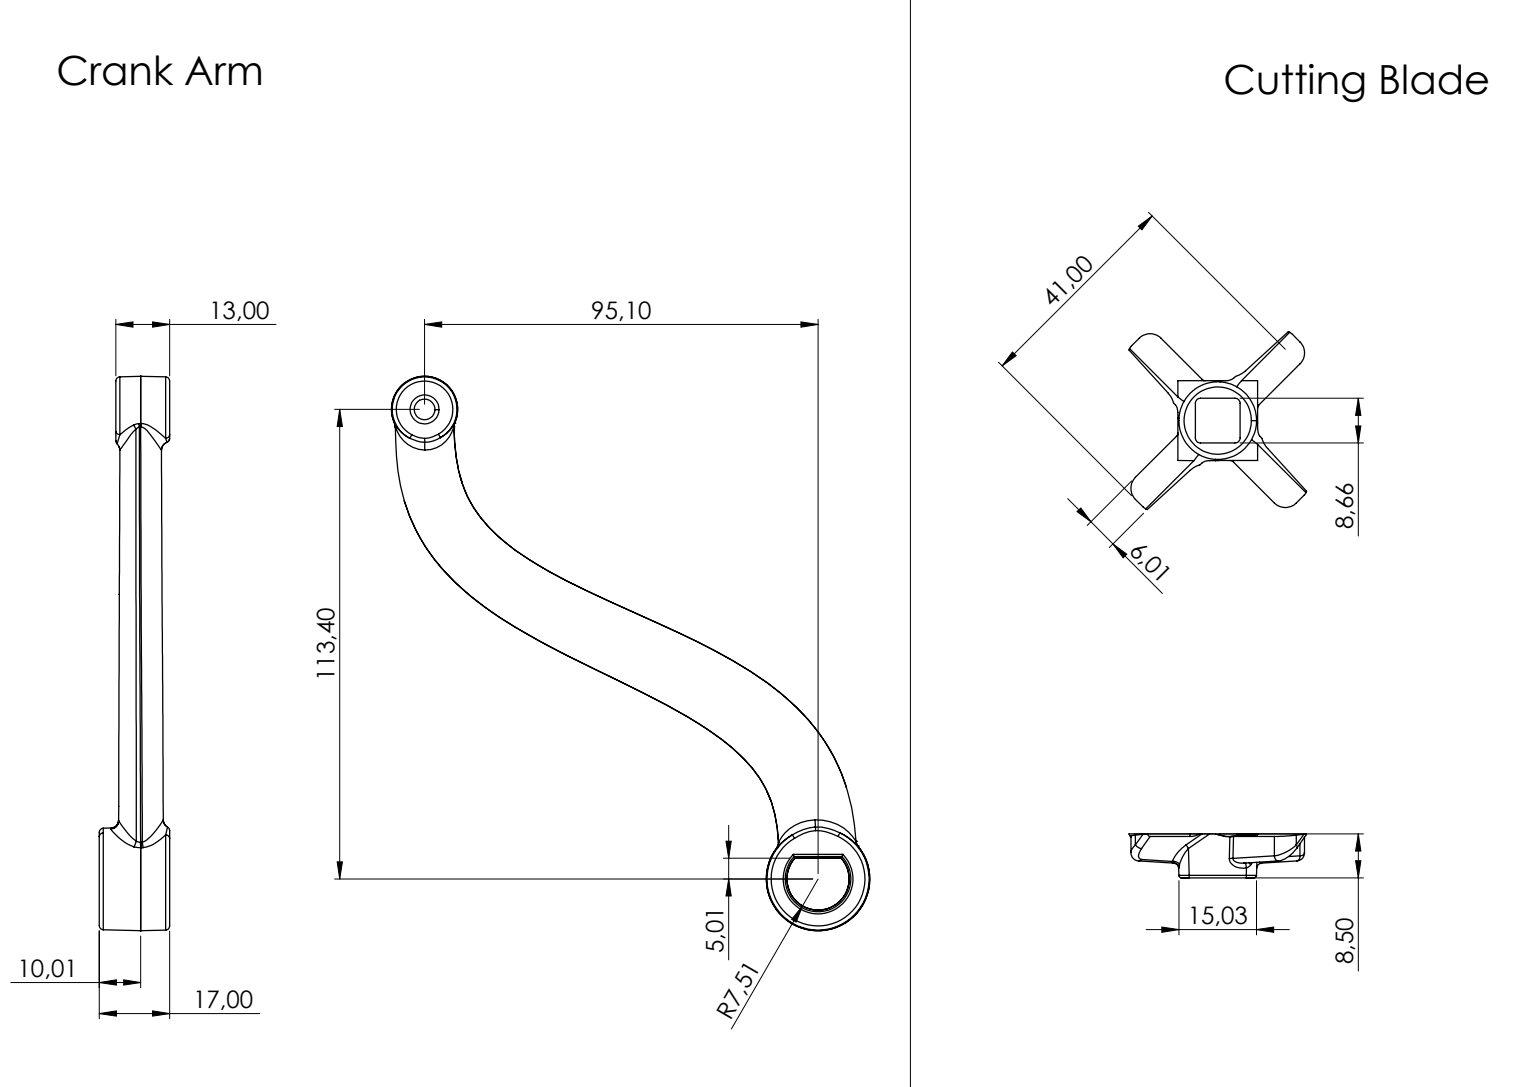
ISO-10303-21;
HEADER;
FILE_DESCRIPTION (('STEP AP214'),
    '1' );
FILE_NAME ('Crank Arm.step',
    '2026-10-06T09:49:54',
    ( '' ),
    ( '' ),
    'SwSTEP 2.0',
    'SolidWorks 2020',
    '' );
FILE_SCHEMA (( 'AUTOMOTIVE_DESIGN' ));
ENDSEC;

DATA;
#26=CARTESIAN_POINT ( 'NONE',  ( 1.285879139104720042E-15, 1391.913060387289988, 209.1218459572589836 ) ) ;
#31=CARTESIAN_POINT ( 'NONE',  ( -109.1321487942470014, 1384.869787291219836, 311.2644937792119322 ) ) ;
#38=CARTESIAN_POINT ( 'NONE',  ( -12.43709857819999876, 1391.584050621440156, 209.7498280055400244 ) ) ;
#39=CARTESIAN_POINT ( 'NONE',  ( -76.44887139282280941, 1385.142738521940146, 277.8929079653030385 ) ) ;
#40=CARTESIAN_POINT ( 'NONE',  ( -11.42765938226460065, 1391.913060387289988, 211.2666090369880010 ) ) ;
#42=ORIENTED_EDGE ( 'NONE', *, *, #61891, .F. ) ;
#48=CARTESIAN_POINT ( 'NONE',  ( -109.4839102700000097, 1384.920896159549784, 311.2841190732590348 ) ) ;
#82=CARTESIAN_POINT ( 'NONE',  ( -12.50903734399489942, 1378.842647904740033, 209.0065662253330174 ) ) ;
#89=ORIENTED_EDGE ( 'NONE', *, *, #96759, .T. ) ;
#109=CARTESIAN_POINT ( 'NONE',  ( -98.27039657997829636, 1384.868559307870100, 295.9020111865049785 ) ) ;
#127=CARTESIAN_POINT ( 'NONE',  ( -16.54254117820000047, 1379.596826475559965, 208.2028925074129688 ) ) ;
#137=DIRECTION ( 'NONE',  ( -1.000000000000000000, 0.000000000000000000, 0.000000000000000000 ) ) ;
#154=DIRECTION ( 'NONE',  ( -0.02617375475769094517, 0.9996573249755578150, 0.0004088821302708953143 ) ) ;
#161=CARTESIAN_POINT ( 'NONE',  ( -7.567241880450000124, 1385.515695150829970, 219.0512258816089854 ) ) ;
#174=EDGE_CURVE ( 'NONE', #66491, #29176, #106889, .T. ) ;
#176=CARTESIAN_POINT ( 'NONE',  ( -12.26345067459182658, 1378.041391332198373, 210.3086285185297868 ) ) ;
#182=CARTESIAN_POINT ( 'NONE',  ( -76.22674438190679780, 1384.646826080419942, 301.0779023118020064 ) ) ;
#183=CARTESIAN_POINT ( 'NONE',  ( -21.60464161394589766, 1384.953571151939968, 202.1045221056799903 ) ) ;
#189=CIRCLE ( 'NONE', #57423, 12.49965726619999984 ) ;
#199=CIRCLE ( 'NONE', #3805, 0.5000000000000157652 ) ;
#212=CARTESIAN_POINT ( 'NONE',  ( -31.38187927383859943, 1379.627610869280034, 219.3043553578710032 ) ) ;
#218=CARTESIAN_POINT ( 'NONE',  ( -106.9777543680000065, 1379.497227361900059, 308.7284971550590171 ) ) ;
#247=CARTESIAN_POINT ( 'NONE',  ( -18.61085923841566014, 1379.601406803549708, 208.6983520666371419 ) ) ;
#248=CARTESIAN_POINT ( 'NONE',  ( -18.76550561599999867, 1380.296266888499986, 210.4015402955490117 ) ) ;
#274=CARTESIAN_POINT ( 'NONE',  ( -62.99252469870000937, 1388.208599921950054, 284.2099993179589887 ) ) ;
#276=CARTESIAN_POINT ( 'NONE',  ( -56.29735061249719763, 1385.085427587770027, 274.2983070328880331 ) ) ;
#299=CARTESIAN_POINT ( 'NONE',  ( -107.7923298369999969, 1386.973993580999831, 297.6574877858589616 ) ) ;
#353=CARTESIAN_POINT ( 'NONE',  ( -8.173822499230000815, 1384.405547763340110, 199.6789892872290011 ) ) ;
#361=EDGE_LOOP ( 'NONE', ( #97319, #80641, #79673, #74910 ) ) ;
#362=DIRECTION ( 'NONE',  ( 1.836970198721029688E-16, 1.000000000000000000, -2.953460612019999929E-19 ) ) ;
#374=ORIENTED_EDGE ( 'NONE', *, *, #31699, .T. ) ;
#375=CARTESIAN_POINT ( 'NONE',  ( -109.5441724410000006, 1374.437034645689891, 304.2218460466590386 ) ) ;
#379=AXIS2_PLACEMENT_3D ( 'NONE', #95016, #67622, #7691 ) ;
#382=CARTESIAN_POINT ( 'NONE',  ( -39.58883837791880467, 1384.581576029320104, 212.5204386266630081 ) ) ;
#389=CARTESIAN_POINT ( 'NONE',  ( -36.13018326403506109, 1379.645813938799392, 224.1534624346936937 ) ) ;
#392=ADVANCED_FACE ( 'NONE', ( #11528 ), #84870, .F. ) ;
#395=CARTESIAN_POINT ( 'NONE',  ( -68.60472032309999690, 1379.747634528509707, 279.7221279746590312 ) ) ;
#404=CARTESIAN_POINT ( 'NONE',  ( -73.55923423229999969, 1384.652831667379814, 298.9494481685590017 ) ) ;
#406=CARTESIAN_POINT ( 'NONE',  ( -13.74298021802130165, 1385.299105108359981, 219.1768037944160028 ) ) ;
#424=CARTESIAN_POINT ( 'NONE',  ( -109.1307141485102790, 1384.906036703127711, 311.2647582669765711 ) ) ;
#446=CARTESIAN_POINT ( 'NONE',  ( -54.30401535559919779, 1383.804998114640057, 270.0689160511349769 ) ) ;
#453=CARTESIAN_POINT ( 'NONE',  ( -53.45887188369999876, 1384.635297440300064, 230.7554238970589893 ) ) ;
#463=CARTESIAN_POINT ( 'NONE',  ( -108.1525126060000019, 1382.602476773729904, 297.8175945742589761 ) ) ;
#465=CARTESIAN_POINT ( 'NONE',  ( -8.752237007995399054, 1384.883920018590061, 220.6821560429810063 ) ) ;
#486=CARTESIAN_POINT ( 'NONE',  ( -105.7100346900000005, 1391.009939533860006, 306.5104643349590106 ) ) ;
#499=EDGE_CURVE ( 'NONE', #98535, #40166, #189, .T. ) ;
#526=EDGE_CURVE ( 'NONE', #91726, #23648, #37737, .T. ) ;
#530=DIRECTION ( 'NONE',  ( 0.03782478994198348876, 0.9992229352747146187, 0.01108200734653209431 ) ) ;
#535=CARTESIAN_POINT ( 'NONE',  ( -8.746878246584900021E-16, 1386.598172472869919, 199.6218459572590120 ) ) ;
#536=CARTESIAN_POINT ( 'NONE',  ( -9.252564866275420741, 1386.194685219555595, 218.4639695156267578 ) ) ;
#544=CARTESIAN_POINT ( 'NONE',  ( -9.786751275049999421, 1380.128435987210196, 216.7642765186190275 ) ) ;
#550=CARTESIAN_POINT ( 'NONE',  ( -13.17267676139999999, 1389.960074679450145, 205.5617118964289887 ) ) ;
#580=CARTESIAN_POINT ( 'NONE',  ( -109.8949752469999908, 1384.902872212460125, 297.0284569597590121 ) ) ;
#584=CARTESIAN_POINT ( 'NONE',  ( -13.93561471908700078, 1390.368461153759881, 210.8007146514599981 ) ) ;
#588=CARTESIAN_POINT ( 'NONE',  ( -107.2899050854710055, 1379.886892357829993, 309.1794776302379546 ) ) ;
#590=CARTESIAN_POINT ( 'NONE',  ( -12.92544628329999945, 1379.594338187410131, 211.1425626820590082 ) ) ;
#591=CARTESIAN_POINT ( 'NONE',  ( -11.31021147849999942, 1391.913060277239993, 206.0247873240190302 ) ) ;
#592=CARTESIAN_POINT ( 'NONE',  ( -73.83470183118490127, 1385.130927357710107, 273.3978214202909953 ) ) ;
#593=CARTESIAN_POINT ( 'NONE',  ( -9.878631019772029731, 1391.913060387289988, 214.6972032143189892 ) ) ;
#628=B_SPLINE_CURVE_WITH_KNOTS ( 'NONE', 3,
 ( #92990, #23025, #91894, #57227, #91357, #49357, #48822, #7343, #24119, #83486, #42053, #109808, #82946 ),
 .UNSPECIFIED., .F., .F.,
 ( 4, 3, 3, 3, 4 ),
 ( -3.958900035302570064, -3.804518807040609740, -3.535848030339469705, -3.399392778577199792, -3.112795747787960199 ),
 .UNSPECIFIED. ) ;
#653=CARTESIAN_POINT ( 'NONE',  ( -88.76367195209469685, 1384.833741781400022, 291.7667102089239961 ) ) ;
#654=ORIENTED_EDGE ( 'NONE', *, *, #54816, .F. ) ;
#670=CARTESIAN_POINT ( 'NONE',  ( -18.79413418600000085, 1379.714553871910084, 209.1009770162550012 ) ) ;
#686=CARTESIAN_POINT ( 'NONE',  ( -8.604752758000000057, 1384.917533019219945, 199.8686412392590057 ) ) ;
#691=CARTESIAN_POINT ( 'NONE',  ( 12.50000000000000000, 1384.913060387289988, 209.1218459572589836 ) ) ;
#723=CARTESIAN_POINT ( 'NONE',  ( -63.98295147832750018, 1384.681148330740143, 287.2755451078210172 ) ) ;
#724=CARTESIAN_POINT ( 'NONE',  ( -27.30672991563199759, 1384.963778074569746, 204.2309128032860031 ) ) ;
#737=ADVANCED_FACE ( 'NONE', ( #27645 ), #103907, .T. ) ;
#741=CARTESIAN_POINT ( 'NONE',  ( -8.579104367239999362, 1382.291193835669901, 200.1141359521089953 ) ) ;
#756=CARTESIAN_POINT ( 'NONE',  ( -59.53909452845530126, 1379.721836142610073, 264.8166016163610266 ) ) ;
#762=CARTESIAN_POINT ( 'NONE',  ( -107.5863934789999945, 1379.032352484299963, 308.9389182505590270 ) ) ;
#779=CARTESIAN_POINT ( 'NONE',  ( -5.013279353754826140, 1375.417533171782679, 203.5257404570949973 ) ) ;
#789=CARTESIAN_POINT ( 'NONE',  ( -57.75160514174648796, 1379.717046060986377, 256.2888408195211696 ) ) ;
#790=CARTESIAN_POINT ( 'NONE',  ( -26.65670438269999920, 1376.179549128069993, 211.2412313610989827 ) ) ;
#794=CARTESIAN_POINT ( 'NONE',  ( -105.5244021762739948, 1378.591211549419995, 305.0228942085889798 ) ) ;
#796=ORIENTED_EDGE ( 'NONE', *, *, #6343, .F. ) ;
#817=CARTESIAN_POINT ( 'NONE',  ( -73.59349969589999318, 1386.581895584289896, 298.9135147644589665 ) ) ;
#842=ADVANCED_FACE ( 'NONE', ( #71348 ), #98540, .T. ) ;
#846=CARTESIAN_POINT ( 'NONE',  ( -109.2380410539999929, 1385.254002988119964, 297.1509341280589638 ) ) ;
#862=CARTESIAN_POINT ( 'NONE',  ( -16.22265104649770251, 1384.873541373520084, 219.7134262672329896 ) ) ;
#891=EDGE_LOOP ( 'NONE', ( #56379, #88097, #94429, #5501 ) ) ;
#908=B_SPLINE_SURFACE_WITH_KNOTS ( 'NONE', 5, 5, ( 
 ( #76165, #109767, #85650, #40900, #100792, #42561 ),
 ( #24083, #8951, #42016, #68898, #58817, #50433 ),
 ( #50973, #580, #49321, #49872, #23545, #57737 ),
 ( #109231, #76714, #83447, #43124, #32515, #51518 ),
 ( #58272, #7306, #75632, #6742, #92956, #67235 ),
 ( #93499, #67780, #16770, #91855, #85103, #33047 ) ),
 .UNSPECIFIED., .F., .F., .F.,
 ( 6, 6 ),
 ( 6, 6 ),
 ( 29.54622938989999881, 29.61002813500000030 ),
 ( 0.000000000000000000, 2.000000000000000000 ),
 .UNSPECIFIED. ) ;
#920=CARTESIAN_POINT ( 'NONE',  ( -113.4000000000000057, 1374.720597897390007, 302.6503168488589495 ) ) ;
#922=CARTESIAN_POINT ( 'NONE',  ( -106.1401956836040057, 1378.913060387289988, 302.5623463823779957 ) ) ;
#927=CARTESIAN_POINT ( 'NONE',  ( -75.49934453870000084, 1384.893650425089845, 276.6853632062590123 ) ) ;
#928=CARTESIAN_POINT ( 'NONE',  ( -51.30093226525310257, 1384.625592632969756, 227.3549881365390206 ) ) ;
#930=CARTESIAN_POINT ( 'NONE',  ( -109.1320112420000044, 1384.953741877089897, 311.2644403302589353 ) ) ;
#939=CARTESIAN_POINT ( 'NONE',  ( -68.65285585769998988, 1379.747727628990106, 279.8365758267589740 ) ) ;
#947=CARTESIAN_POINT ( 'NONE',  ( -54.13887208369999371, 1385.096747890979941, 270.3642349231589606 ) ) ;
#993=CARTESIAN_POINT ( 'NONE',  ( -69.93979052779329209, 1383.785293178040092, 294.7370205497300049 ) ) ;
#994=CIRCLE ( 'NONE', #29578, 2.000079901618746270 ) ;
#995=CARTESIAN_POINT ( 'NONE',  ( -108.2039566672529958, 1378.913060387289988, 299.7295690038039879 ) ) ;
#1001=CARTESIAN_POINT ( 'NONE',  ( -59.38610754540000158, 1383.797318715759957, 279.8430129459590034 ) ) ;
#1013=CARTESIAN_POINT ( 'NONE',  ( -107.7596963679999931, 1382.859817520469733, 297.6961126062590210 ) ) ;
#1046=CARTESIAN_POINT ( 'NONE',  ( -9.503490513250000049, 1386.215136675220037, 200.2136258941289952 ) ) ;
#1081=ORIENTED_EDGE ( 'NONE', *, *, #10293, .T. ) ;
#1084=B_SPLINE_SURFACE_WITH_KNOTS ( 'NONE', 5, 5, ( 
 ( #42749, #102620, #93139, #762, #85849, #103180 ),
 ( #34890, #218, #51153, #9687, #84733, #92581 ),
 ( #33232, #25920, #67975, #26482, #60118, #94804 ),
 ( #15853, #33779, #18079, #52274, #42199, #76350 ),
 ( #75802, #78002, #24807, #32689, #110499, #109953 ),
 ( #66869, #100977, #24273, #102083, #67421, #101520 ),
 ( #25366, #70203, #78561, #19744, #46081, #11906 ),
 ( #105977, #61246, #70749, #11367, #10810, #46631 ),
 ( #12446, #89158, #54491, #28149, #104860, #88626 ) ),
 .UNSPECIFIED., .F., .F., .F.,
 ( 6, 3, 6 ),
 ( 6, 6 ),
 ( 0.000000000000000000, 5.531936552890000414, 12.17660274970000067 ),
 ( 0.000000000000000000, 1.000000000000000000 ),
 .UNSPECIFIED. ) ;
#1086=CARTESIAN_POINT ( 'NONE',  ( -13.39809219260000006, 1386.967483829560024, 218.7383260501090092 ) ) ;
#1095=CARTESIAN_POINT ( 'NONE',  ( -10.13100692099999911, 1382.082910451279986, 217.5460056582589914 ) ) ;
#1101=CARTESIAN_POINT ( 'NONE',  ( -11.29470234270000084, 1390.474510999679978, 203.7985412330889972 ) ) ;
#1129=CARTESIAN_POINT ( 'NONE',  ( -8.083483728235815846, 1386.109445660887104, 199.6283091834757215 ) ) ;
#1136=CARTESIAN_POINT ( 'NONE',  ( -13.26126580242469899, 1390.209151648439956, 212.6158348635119921 ) ) ;
#1140=CARTESIAN_POINT ( 'NONE',  ( -108.8427904636022134, 1381.850845790319909, 310.6994421841279745 ) ) ;
#1141=CARTESIAN_POINT ( 'NONE',  ( -12.26108091377107634, 1377.626920165065258, 208.0100024370453298 ) ) ;
#1144=CARTESIAN_POINT ( 'NONE',  ( -86.70549396914439910, 1385.182048704240060, 290.2386611732610504 ) ) ;
#1146=CARTESIAN_POINT ( 'NONE',  ( -9.946516861848831326, 1391.913060387289988, 214.5797999757839989 ) ) ;
#1147=CARTESIAN_POINT ( 'NONE',  ( -32.53397683490000247, 1379.726329037039932, 216.1069825312089847 ) ) ;
#1175=DIRECTION ( 'NONE',  ( -0.9998780014336184907, 0.000000000000000000, 0.01561993114942984012 ) ) ;
#1203=CARTESIAN_POINT ( 'NONE',  ( -97.03291587454688738, 1384.864417997589953, 295.5831496746029643 ) ) ;
#1220=CARTESIAN_POINT ( 'NONE',  ( -16.52535657530000179, 1379.585817439869743, 208.2843806234300246 ) ) ;
#1224=CARTESIAN_POINT ( 'NONE',  ( -68.75533708345575690, 1379.747887839387431, 280.3280563178295210 ) ) ;
#1239=CARTESIAN_POINT ( 'NONE',  ( -13.57816498729999921, 1379.569537801319939, 207.8818212186490086 ) ) ;
#1266=AXIS2_PLACEMENT_3D ( 'NONE', #76000, #101734, #93889 ) ;
#1271=CARTESIAN_POINT ( 'NONE',  ( -77.89971934322829838, 1384.643069586999900, 302.3865563694679963 ) ) ;
#1272=CARTESIAN_POINT ( 'NONE',  ( -18.95953277411649651, 1384.948900335349890, 201.3970670253520154 ) ) ;
#1289=CARTESIAN_POINT ( 'NONE',  ( -8.219449892280000114, 1384.003553985900226, 199.7324766670489851 ) ) ;
#1301=CIRCLE ( 'NONE', #74597, 2.000013666866326201 ) ;
#1302=CARTESIAN_POINT ( 'NONE',  ( -66.37701120922260145, 1379.742216766350111, 277.0613536044180023 ) ) ;
#1310=CARTESIAN_POINT ( 'NONE',  ( -7.767687465479999886, 1384.983142744430097, 218.9170564598889825 ) ) ;
#1329=AXIS2_PLACEMENT_3D ( 'NONE', #10990, #55217, #12641 ) ;
#1333=CARTESIAN_POINT ( 'NONE',  ( -49.27402874327646742, 1379.685930775072848, 238.1797779762692926 ) ) ;
#1349=CARTESIAN_POINT ( 'NONE',  ( 3.555115653736739510E-15, 1384.926148861439970, 209.1218459572589836 ) ) ;
#1352=CARTESIAN_POINT ( 'NONE',  ( -104.6408027911641483, 1379.604531764216517, 304.0225355773446836 ) ) ;
#1361=CARTESIAN_POINT ( 'NONE',  ( -73.55519582189999994, 1385.011955127469946, 298.9534985252589649 ) ) ;
#1372=CARTESIAN_POINT ( 'NONE',  ( -108.8616956595720069, 1383.655566382730058, 311.0497432310580166 ) ) ;
#1421=CARTESIAN_POINT ( 'NONE',  ( -109.5441724370000003, 1379.437061298989875, 305.1680627026370303 ) ) ;
#1450=B_SPLINE_SURFACE_WITH_KNOTS ( 'NONE', 5, 5, ( 
 ( #90304, #23657, #57839, #21975, #56167, #91966 ),
 ( #81906, #38256, #5775, #72439, #106571, #29857 ),
 ( #39364, #98160, #89765, #73538, #75188, #85766 ),
 ( #58381, #66797, #17432, #24733, #33156, #58930 ),
 ( #75733, #25842, #67896, #686, #7958, #109877 ),
 ( #110422, #67345, #101443, #93061, #16335, #17998 ) ),
 .UNSPECIFIED., .F., .F., .F.,
 ( 6, 6 ),
 ( 6, 6 ),
 ( 0.9322655043309999723, 1.047387711740000116 ),
 ( 0.000000000000000000, 2.000000000000000000 ),
 .UNSPECIFIED. ) ;
#1454=CARTESIAN_POINT ( 'NONE',  ( -87.43041093610000303, 1379.577971548199912, 299.9734862988590294 ) ) ;
#1456=ADVANCED_FACE ( 'NONE', ( #108738 ), #94755, .F. ) ;
#1466=CARTESIAN_POINT ( 'NONE',  ( -58.30221543510000259, 1384.791840522580060, 240.0691493971590091 ) ) ;
#1468=CARTESIAN_POINT ( 'NONE',  ( -65.89286211545359606, 1384.710728713680055, 257.0461978634630213 ) ) ;
#1471=CARTESIAN_POINT ( 'NONE',  ( -103.5990824459999970, 1389.912137903419989, 305.4537645068589882 ) ) ;
#1480=CARTESIAN_POINT ( 'NONE',  ( -68.67274465469999711, 1379.748163774529985, 279.9618448723590518 ) ) ;
#1482=CARTESIAN_POINT ( 'NONE',  ( -115.5939564047259296, 1379.013060387289897, 305.4204098037694735 ) ) ;
#1489=CARTESIAN_POINT ( 'NONE',  ( -38.49223698079999423, 1385.058880994630044, 239.3118539506589855 ) ) ;
#1491=CARTESIAN_POINT ( 'NONE',  ( -105.7942887633819993, 1378.913060387289988, 304.0474587704230203 ) ) ;
#1508=B_SPLINE_CURVE_WITH_KNOTS ( 'NONE', 3,
 ( #110150, #9352, #101176, #24470, #42390, #60313 ),
 .UNSPECIFIED., .F., .F.,
 ( 4, 2, 4 ),
 ( 0.000000000000000000, 0.5000000000000000000, 1.000000000000000000 ),
 .UNSPECIFIED. ) ;
#1535=CIRCLE ( 'NONE', #87369, 12.26364123839999998 ) ;
#1538=CARTESIAN_POINT ( 'NONE',  ( -75.52559667918460207, 1383.780383530929839, 300.2699059305949731 ) ) ;
#1545=VERTEX_POINT ( 'NONE', #63867 ) ;
#1547=CARTESIAN_POINT ( 'NONE',  ( -87.19453865519999169, 1382.337400661289848, 307.1204035211590053 ) ) ;
#1557=CARTESIAN_POINT ( 'NONE',  ( -109.2768968829999920, 1384.496076674440019, 297.1408104247589677 ) ) ;
#1573=FACE_OUTER_BOUND ( 'NONE', #66351, .T. ) ;
#1601=EDGE_CURVE ( 'NONE', #93351, #108323, #72640, .T. ) ;
#1634=CARTESIAN_POINT ( 'NONE',  ( -20.33527840200000014, 1390.981646659919761, 210.8560405308990084 ) ) ;
#1635=CARTESIAN_POINT ( 'NONE',  ( -14.24353422718318463, 1390.369519709444148, 210.8398536836253356 ) ) ;
#1645=CARTESIAN_POINT ( 'NONE',  ( -8.680550271810000496, 1382.887713811429876, 218.3027530060789729 ) ) ;
#1662=CARTESIAN_POINT ( 'NONE',  ( -106.3976693117229928, 1390.939243848519936, 307.7527733253859878 ) ) ;
#1671=CARTESIAN_POINT ( 'NONE',  ( -31.84935467931069297, 1383.839719338520126, 229.8416280207219984 ) ) ;
#1680=CARTESIAN_POINT ( 'NONE',  ( -1.458447685501650145E-16, 1382.910363916049846, 199.8625637235290071 ) ) ;
#1687=CARTESIAN_POINT ( 'NONE',  ( -14.52654072983339972, 1379.768571760160057, 208.3454318067070119 ) ) ;
#1695=CARTESIAN_POINT ( 'NONE',  ( -12.08187496630000091, 1391.708070121689843, 207.0208056324590018 ) ) ;
#1696=CARTESIAN_POINT ( 'NONE',  ( -98.94538731745480220, 1385.218168442259866, 296.0687099710040115 ) ) ;
#1731=FACE_OUTER_BOUND ( 'NONE', #74136, .T. ) ;
#1739=CARTESIAN_POINT ( 'NONE',  ( -13.86717347501279995, 1379.678627288110192, 208.3009849253440109 ) ) ;
#1749=ORIENTED_EDGE ( 'NONE', *, *, #3895, .F. ) ;
#1763=CARTESIAN_POINT ( 'NONE',  ( -102.6485531311329993, 1384.882470662279957, 296.6730287615140469 ) ) ;
#1781=CARTESIAN_POINT ( 'NONE',  ( -41.95996988479999601, 1379.671663521220125, 226.0894461641589999 ) ) ;
#1784=CARTESIAN_POINT ( 'NONE',  ( -68.56276905708799063, 1379.747764319654607, 280.1490247722647950 ) ) ;
#1797=ORIENTED_EDGE ( 'NONE', *, *, #100031, .F. ) ;
#1799=CARTESIAN_POINT ( 'NONE',  ( -7.545064063707340729, 1384.907232462019920, 219.0876311385090105 ) ) ;
#1817=DIRECTION ( 'NONE',  ( 0.1225044380228070551, 0.9831695928899274461, -0.1355367635786350333 ) ) ;
#1824=CARTESIAN_POINT ( 'NONE',  ( -7.628194758486819715, 1383.866806825199774, 218.9897990120470013 ) ) ;
#1837=CARTESIAN_POINT ( 'NONE',  ( -69.10968088804719400, 1384.665037752149829, 294.0407317603679758 ) ) ;
#1838=CARTESIAN_POINT ( 'NONE',  ( -15.47609788629169891, 1384.942714744960085, 200.6910050388860043 ) ) ;
#1852=CARTESIAN_POINT ( 'NONE',  ( -106.6950745027010043, 1391.913060387289988, 305.9031442834140080 ) ) ;
#1857=CARTESIAN_POINT ( 'NONE',  ( -14.08318393682589864, 1379.709325990200114, 211.5303917806009792 ) ) ;
#1871=CARTESIAN_POINT ( 'NONE',  ( -65.43163292693739663, 1379.743657604059763, 275.4463174256679849 ) ) ;
#1903=CARTESIAN_POINT ( 'NONE',  ( -44.66902661210603043, 1379.669579522011190, 230.0472852312407497 ) ) ;
#1915=EDGE_CURVE ( 'NONE', #68857, #40412, #43486, .T. ) ;
#1924=CARTESIAN_POINT ( 'NONE',  ( -105.0581303879369983, 1379.236400313860031, 304.0328620142400382 ) ) ;
#1933=CARTESIAN_POINT ( 'NONE',  ( -74.25289801200000284, 1388.141632471819776, 298.2335420860590034 ) ) ;
#1944=CARTESIAN_POINT ( 'NONE',  ( -105.6599733740739993, 1378.369188341159997, 305.5461949359690266 ) ) ;
#1967=AXIS2_PLACEMENT_3D ( 'NONE', #95143, #19521, #53727 ) ;
#1972=CARTESIAN_POINT ( 'NONE',  ( -9.627136608023121767, 1384.891069265470151, 218.7309310236159945 ) ) ;
#2027=CARTESIAN_POINT ( 'NONE',  ( -77.18524044800000183, 1379.656469663269945, 292.4664101653590365 ) ) ;
#2034=CARTESIAN_POINT ( 'NONE',  ( -113.4000000000000057, 1385.138976307909843, 297.2272069998589927 ) ) ;
#2035=CARTESIAN_POINT ( 'NONE',  ( -60.36450283880899548, 1384.675237924389876, 244.7949774597909993 ) ) ;
#2047=CARTESIAN_POINT ( 'NONE',  ( -65.32973268749998397, 1379.744446857699813, 273.2270638632589908 ) ) ;
#2055=CARTESIAN_POINT ( 'NONE',  ( -38.48821451509999747, 1384.926710553620069, 239.3141293533589931 ) ) ;
#2103=CARTESIAN_POINT ( 'NONE',  ( -101.9385972633359927, 1383.762759256019990, 310.8318512473720148 ) ) ;
#2106=CARTESIAN_POINT ( 'NONE',  ( -109.0682903905509988, 1384.413520338990111, 311.2316106067269743 ) ) ;
#2112=CARTESIAN_POINT ( 'NONE',  ( -85.86261655710001151, 1384.821806127680020, 289.6800030968590249 ) ) ;
#2122=CARTESIAN_POINT ( 'NONE',  ( -109.9959328080000063, 1384.355667310579975, 296.9977477969590041 ) ) ;
#2199=CARTESIAN_POINT ( 'NONE',  ( -24.70417392370000087, 1389.604960788569997, 206.5185001640990095 ) ) ;
#2238=CARTESIAN_POINT ( 'NONE',  ( -35.56111957166950077, 1383.834697306850103, 234.6955540351449940 ) ) ;
#2248=CARTESIAN_POINT ( 'NONE',  ( -105.0581303879369983, 1379.236400313860031, 304.0328620142400382 ) ) ;
#2249=CARTESIAN_POINT ( 'NONE',  ( -8.296934851823509760, 1386.806139525614526, 199.8388016180733473 ) ) ;
#2255=CARTESIAN_POINT ( 'NONE',  ( -12.31958819330829868, 1391.699967522870111, 210.6753496357469828 ) ) ;
#2259=ADVANCED_FACE ( 'NONE', ( #50931 ), #6146, .T. ) ;
#2263=CARTESIAN_POINT ( 'NONE',  ( -7.966114795899199130, 1384.917223774180002, 199.4892816035240060 ) ) ;
#2264=CARTESIAN_POINT ( 'NONE',  ( -102.2538918586309933, 1385.226474943340008, 296.6373044331759843 ) ) ;
#2291=CARTESIAN_POINT ( 'NONE',  ( -106.6038969349999945, 1381.976044154610008, 298.3535665123590093 ) ) ;
#2321=CARTESIAN_POINT ( 'NONE',  ( -12.25307189289999954, 1391.743053431310045, 210.3744810088190036 ) ) ;
#2339=CARTESIAN_POINT ( 'NONE',  ( -44.27735363219999698, 1379.663868217249956, 229.4728106293590031 ) ) ;
#2343=CARTESIAN_POINT ( 'NONE',  ( -67.15060528499047621, 1379.747519056922101, 278.1647121854331886 ) ) ;
#2350=CARTESIAN_POINT ( 'NONE',  ( -67.08107980928619440, 1385.034953735319959, 291.5504916563910456 ) ) ;
#2352=CARTESIAN_POINT ( 'NONE',  ( -8.970890765399998301, 1384.951408361539961, 199.9338804842589923 ) ) ;
#2366=DIRECTION ( 'NONE',  ( 0.0001171895853481130984, -0.004053780167009412259, -0.9999917765326665764 ) ) ;
#2385=CARTESIAN_POINT ( 'NONE',  ( -7.768355502971520110, 1383.288536228370049, 218.8604790520440133 ) ) ;
#2399=CARTESIAN_POINT ( 'NONE',  ( -76.64144279794061276, 1384.645875352879784, 301.4166218965220310 ) ) ;
#2400=CARTESIAN_POINT ( 'NONE',  ( -31.39107788089150120, 1384.971443476370041, 206.3467394566210089 ) ) ;
#2407=CARTESIAN_POINT ( 'NONE',  ( -8.847848347470000263, 1384.943898188619869, 199.9248160043189841 ) ) ;
#2417=CARTESIAN_POINT ( 'NONE',  ( -9.813982587879999997, 1383.225161719749849, 200.4195862986289853 ) ) ;
#2430=CARTESIAN_POINT ( 'NONE',  ( -65.82654097011999283, 1379.741992558670063, 276.1399068737349580 ) ) ;
#2443=CARTESIAN_POINT ( 'NONE',  ( -106.0207696801649888, 1378.913060388890017, 305.3967244531619940 ) ) ;
#2456=CIRCLE ( 'NONE', #52702, 8.432239102140000497 ) ;
#2460=CARTESIAN_POINT ( 'NONE',  ( -8.862374925020001015, 1384.916129524170174, 218.6851829152190305 ) ) ;
#2463=CARTESIAN_POINT ( 'NONE',  ( -49.26428229891999422, 1379.685895086444134, 238.1610838164967845 ) ) ;
#2477=CARTESIAN_POINT ( 'NONE',  ( 10.11243515225073253, 1384.926148861439970, 216.4689601570716206 ) ) ;
#2484=CARTESIAN_POINT ( 'NONE',  ( -104.8708816957486079, 1379.440243493634625, 304.0281164857488534 ) ) ;
#2487=CARTESIAN_POINT ( 'NONE',  ( -9.094257307180781069, 1384.874748761890260, 199.9429999480310016 ) ) ;
#2492=CARTESIAN_POINT ( 'NONE',  ( -102.7364941740000006, 1384.940050820800025, 311.2335147922589726 ) ) ;
#2503=CARTESIAN_POINT ( 'NONE',  ( -105.9021060456189929, 1378.331563972840058, 306.6119379298179979 ) ) ;
#2529=CARTESIAN_POINT ( 'NONE',  ( -21.51311642161260096, 1384.857552017839907, 221.6326953624779890 ) ) ;
#2563=CARTESIAN_POINT ( 'NONE',  ( -107.2481891120000057, 1387.964334016630119, 309.9317261882590628 ) ) ;
#2585=CARTESIAN_POINT ( 'NONE',  ( -77.18524045069999318, 1374.656469662890004, 292.4664101653590365 ) ) ;
#2586=CARTESIAN_POINT ( 'NONE',  ( -106.9163825377050046, 1378.913060387289988, 301.2728918013489761 ) ) ;
#2594=DIRECTION ( 'NONE',  ( -1.000000000000000000, 0.000000000000000000, 0.000000000000000000 ) ) ;
#2597=CARTESIAN_POINT ( 'NONE',  ( -8.743435183079999007, 1384.548231727749908, 218.5812667456789882 ) ) ;
#2602=CARTESIAN_POINT ( 'NONE',  ( -65.82430152899999598, 1379.749194687180079, 274.2810710116589803 ) ) ;
#2611=CARTESIAN_POINT ( 'NONE',  ( -47.38272174249999580, 1385.138016709929843, 256.2741787814589998 ) ) ;
#2613=CARTESIAN_POINT ( 'NONE',  ( -33.03375078350489957, 1385.219055440710008, 231.5328850939089875 ) ) ;
#2657=CARTESIAN_POINT ( 'NONE',  ( -93.71881660438820916, 1383.767977992140004, 309.5718267011319540 ) ) ;
#2659=CARTESIAN_POINT ( 'NONE',  ( -109.2480983758639894, 1384.372607579929991, 311.2262217477910440 ) ) ;
#2666=CARTESIAN_POINT ( 'NONE',  ( -92.78435512849998190, 1384.849527344140142, 294.1459074807589786 ) ) ;
#2672=CARTESIAN_POINT ( 'NONE',  ( -109.3498435130000104, 1384.940401497779931, 297.1386112594590259 ) ) ;
#2704=CARTESIAN_POINT ( 'NONE',  ( -113.4000000000000057, 1390.913060387289988, 304.2218459572590064 ) ) ;
#2737=CARTESIAN_POINT ( 'NONE',  ( -11.65147249325539924, 1391.913060387150153, 208.7366933367970034 ) ) ;
#2748=CARTESIAN_POINT ( 'NONE',  ( -25.91586689989999925, 1384.961148014880109, 203.4475886829490037 ) ) ;
#2755=CARTESIAN_POINT ( 'NONE',  ( -8.001312726290001009, 1383.415254610280044, 218.6981543553289953 ) ) ;
#2773=CARTESIAN_POINT ( 'NONE',  ( -109.8950784940000034, 1385.179886903279794, 297.0358873837590181 ) ) ;
#2777=FACE_OUTER_BOUND ( 'NONE', #106070, .T. ) ;
#2784=CARTESIAN_POINT ( 'NONE',  ( -23.70810543552709859, 1383.849544535609994, 222.6483769287150096 ) ) ;
#2787=DIRECTION ( 'NONE',  ( 1.835183309750130004E-16, 1.000000000000000000, 1.599799320660000123E-19 ) ) ;
#2792=CARTESIAN_POINT ( 'NONE',  ( -8.911791977641406959, 1388.063585253917608, 200.4736995634368100 ) ) ;
#2801=CARTESIAN_POINT ( 'NONE',  ( -12.56550536004469976, 1389.228114667070031, 215.4313542344819723 ) ) ;
#2808=CARTESIAN_POINT ( 'NONE',  ( -104.7009857956030032, 1385.232336910320100, 296.9001550543150074 ) ) ;
#2831=ORIENTED_EDGE ( 'NONE', *, *, #37412, .T. ) ;
#2837=LINE ( 'NONE', #28569, #78414 ) ;
#2881=CARTESIAN_POINT ( 'NONE',  ( -108.8461099330000081, 1385.969494106900129, 297.2525754554590094 ) ) ;
#2886=EDGE_CURVE ( 'NONE', #77278, #33852, #29899, .T. ) ;
#2889=CARTESIAN_POINT ( 'NONE',  ( -62.71435643172744534, 1379.746901600607089, 270.6043089139369613 ) ) ;
#2895=CARTESIAN_POINT ( 'NONE',  ( -55.66345240404490369, 1385.088922544829984, 273.0910554044640435 ) ) ;
#2897=CARTESIAN_POINT ( 'NONE',  ( -8.848347859410001348, 1384.947984491080206, 199.9153136718090025 ) ) ;
#2923=CIRCLE ( 'NONE', #49338, 3.500000000000003109 ) ;
#2924=CARTESIAN_POINT ( 'NONE',  ( -12.31353720152530151, 1377.792119713679995, 208.8773538342209974 ) ) ;
#2944=CARTESIAN_POINT ( 'NONE',  ( -109.1111611177930030, 1384.583257041720117, 311.2497810013429671 ) ) ;
#2945=CARTESIAN_POINT ( 'NONE',  ( -30.61862460611610359, 1384.969957910880112, 205.9038405460119918 ) ) ;
#2961=CARTESIAN_POINT ( 'NONE',  ( -107.1805148838380006, 1391.913060387289988, 307.0819323254360143 ) ) ;
#2965=CARTESIAN_POINT ( 'NONE',  ( -12.26059043289999906, 1378.259319071080199, 207.8536745223389914 ) ) ;
#2977=CARTESIAN_POINT ( 'NONE',  ( -67.97495219347740658, 1379.746072679010013, 279.4294113511920159 ) ) ;
#2983=CARTESIAN_POINT ( 'NONE',  ( -109.1312185580000005, 1384.935967175139922, 311.2646235902590206 ) ) ;
#2999=CARTESIAN_POINT ( 'NONE',  ( -11.03495751070000175, 1391.553749705140035, 203.9031261639289880 ) ) ;
#3000=ORIENTED_EDGE ( 'NONE', *, *, #54836, .F. ) ;
#3006=CARTESIAN_POINT ( 'NONE',  ( -8.298094033859999996, 1384.915121724699929, 218.7036151108189870 ) ) ;
#3009=CARTESIAN_POINT ( 'NONE',  ( -68.43938665331394589, 1379.747307078699578, 279.3521370341155148 ) ) ;
#3011=ADVANCED_FACE ( 'NONE', ( #66387 ), #102765, .F. ) ;
#3016=ORIENTED_EDGE ( 'NONE', *, *, #24009, .F. ) ;
#3023=CARTESIAN_POINT ( 'NONE',  ( -23.99542451635583262, 1379.613613144763121, 214.7981695600689704 ) ) ;
#3042=CARTESIAN_POINT ( 'NONE',  ( -75.53845940079999366, 1389.374618531590158, 296.9084575487589746 ) ) ;
#3054=CARTESIAN_POINT ( 'NONE',  ( -105.4833704291039993, 1380.472658686770046, 307.8541256062359821 ) ) ;
#3080=CARTESIAN_POINT ( 'NONE',  ( -26.69200297127330046, 1384.840286869720103, 224.9839128895910108 ) ) ;
#3096=CARTESIAN_POINT ( 'NONE',  ( -14.31906343784990021, 1380.323795378649947, 209.9058136714729983 ) ) ;
#3103=CARTESIAN_POINT ( 'NONE',  ( -76.47832706378659395, 1379.656496316390076, 293.1148347572179773 ) ) ;
#3112=CARTESIAN_POINT ( 'NONE',  ( -8.737946438520001635, 1383.987033302019881, 218.5474386001390030 ) ) ;
#3136=CARTESIAN_POINT ( 'NONE',  ( -94.75917112700000189, 1379.224093153639842, 301.3391293692590125 ) ) ;
#3137=CARTESIAN_POINT ( 'NONE',  ( -105.8293410826149881, 1378.913060387450059, 303.6100817853489957 ) ) ;
#3149=CARTESIAN_POINT ( 'NONE',  ( -3.078458293690000236, 1384.210421809239961, 218.5154548192989807 ) ) ;
#3154=CARTESIAN_POINT ( 'NONE',  ( -65.39677373169999441, 1379.739124186490017, 273.1945630607590374 ) ) ;
#3164=CARTESIAN_POINT ( 'NONE',  ( -102.7364477239999871, 1384.825249911479887, 311.2346497062589492 ) ) ;
#3166=CARTESIAN_POINT ( 'NONE',  ( -36.10181457510150693, 1385.203388602290033, 235.7704352495559874 ) ) ;
#3170=DIRECTION ( 'NONE',  ( -0.9076061524720632212, 0.000000000000000000, 0.4198226673190215696 ) ) ;
#3175=CARTESIAN_POINT ( 'NONE',  ( -5.789140635075909813, 1391.897372272190069, 215.0545055588169987 ) ) ;
#3196=CARTESIAN_POINT ( 'NONE',  ( -111.2060435952740676, 1390.913060387289988, 303.0232821107484824 ) ) ;
#3212=CARTESIAN_POINT ( 'NONE',  ( -93.31501789313530537, 1383.768231546839843, 309.4758065345690170 ) ) ;
#3218=B_SPLINE_CURVE_WITH_KNOTS ( 'NONE', 3,
 ( #27078, #69654, #94819, #779, #62355, #77478 ),
 .UNSPECIFIED., .F., .F.,
 ( 4, 2, 4 ),
 ( -0.08353783071465489818, -0.08289724164866060785, -0.08222331866850060567 ),
 .UNSPECIFIED. ) ;
#3219=CARTESIAN_POINT ( 'NONE',  ( -84.23427087509999467, 1380.672444284130052, 291.6063032490590103 ) ) ;
#3224=CARTESIAN_POINT ( 'NONE',  ( -109.8949053929999877, 1384.921907949040133, 297.0284378280589976 ) ) ;
#3296=ADVANCED_FACE ( 'NONE', ( #71789 ), #3304, .T. ) ;
#3298=CARTESIAN_POINT ( 'NONE',  ( -37.25179242459999784, 1388.439297844689918, 234.7543419479590057 ) ) ;
#3299=CARTESIAN_POINT ( 'NONE',  ( -9.094257307180781069, 1384.874748761890260, 199.9429999480310016 ) ) ;
#3304=TOROIDAL_SURFACE ( 'NONE', #110537, 8.432239102140000497, 0.5000000000000000000 ) ;
#3320=AXIS2_PLACEMENT_3D ( 'NONE', #70591, #45924, #21217 ) ;
#3327=B_SPLINE_CURVE_WITH_KNOTS ( 'NONE', 3,
 ( #6516, #74842, #32271, #58038, #92718, #103883, #76476, #101651, #34476, #27183, #50725, #75926, #77041 ),
 .UNSPECIFIED., .F., .F.,
 ( 4, 3, 3, 3, 4 ),
 ( 0.9031056323884600889, 0.9451379527402459235, 0.9933535966189359634, 1.028735865613630063, 1.041569240497630000 ),
 .UNSPECIFIED. ) ;
#3328=FACE_OUTER_BOUND ( 'NONE', #62628, .T. ) ;
#3339=CARTESIAN_POINT ( 'NONE',  ( -22.49235462320989853, 1383.850897880320190, 221.9470685874750018 ) ) ;
#3345=ORIENTED_EDGE ( 'NONE', *, *, #72188, .T. ) ;
#3347=CARTESIAN_POINT ( 'NONE',  ( -10.88383664749751745, 1390.636386471471496, 203.2482663326153158 ) ) ;
#3353=CARTESIAN_POINT ( 'NONE',  ( -11.56183394306549950, 1388.455280331700123, 216.7304925199499905 ) ) ;
#3361=CARTESIAN_POINT ( 'NONE',  ( -89.02070098190330327, 1385.189645878620240, 291.9514036105480272 ) ) ;
#3362=DIRECTION ( 'NONE',  ( 1.836970198721029688E-16, 1.000000000000000000, 0.000000000000000000 ) ) ;
#3401=CARTESIAN_POINT ( 'NONE',  ( -6.355004503879999156, 1384.926023117790010, 199.7181650675090054 ) ) ;
#3403=ORIENTED_EDGE ( 'NONE', *, *, #51030, .F. ) ;
#3440=CARTESIAN_POINT ( 'NONE',  ( -55.35242389386650075, 1385.090656389910237, 272.4922876094810249 ) ) ;
#3441=B_SPLINE_SURFACE_WITH_KNOTS ( 'NONE', 5, 5, ( 
 ( #25923, #43857, #8032, #33234, #60120, #94238 ),
 ( #17513, #51711, #30752, #105829, #55426, #64933 ),
 ( #55974, #72777, #4468, #90098, #37506, #95362 ),
 ( #18623, #39145, #12847, #72237, #99046, #106363 ),
 ( #13381, #29649, #89558, #81154, #98505, #106904 ),
 ( #47028, #35450, #47569, #30191, #64385, #20679 ),
 ( #38597, #107457, #21773, #11752, #81694, #5000 ),
 ( #22324, #1310, #80058, #45923, #73320, #56526 ),
 ( #63836, #69638, #3930, #97948, #46484, #54336 ) ),
 .UNSPECIFIED., .F., .F., .F.,
 ( 6, 3, 6 ),
 ( 6, 6 ),
 ( 10.04884080650000122, 10.52102568589999976, 10.99321056540000008 ),
 ( 0.000000000000000000, 2.000000000000000000 ),
 .UNSPECIFIED. ) ;
#3465=VECTOR ( 'NONE', #20873, 1000.000000000000000 ) ;
#3469=CARTESIAN_POINT ( 'NONE',  ( -13.68999425486880028, 1379.602495655479970, 208.0136990666040049 ) ) ;
#3476=CARTESIAN_POINT ( 'NONE',  ( -7.655626746931960547, 1383.726789944049870, 218.9639101100850098 ) ) ;
#3490=CARTESIAN_POINT ( 'NONE',  ( -95.18509927322880060, 1384.609717790749983, 310.0734934036659638 ) ) ;
#3491=CARTESIAN_POINT ( 'NONE',  ( -46.36155058326189504, 1385.007142338620042, 220.0507881939000185 ) ) ;
#3492=CARTESIAN_POINT ( 'NONE',  ( -5.436526647126479261, 1374.917605893529981, 214.9039629178479913 ) ) ;
#3498=CARTESIAN_POINT ( 'NONE',  ( -8.604502001330001093, 1384.928348898680042, 199.8686409361690153 ) ) ;
#3525=CARTESIAN_POINT ( 'NONE',  ( -67.80648804034809984, 1379.745630162259886, 279.2148224231119684 ) ) ;
#3556=CARTESIAN_POINT ( 'NONE',  ( -8.022926871310001928, 1384.932834875369963, 218.7874489595089926 ) ) ;
#3559=CARTESIAN_POINT ( 'NONE',  ( -12.34121275650000094, 1378.648013544750029, 208.9830469583500019 ) ) ;
#3560=CARTESIAN_POINT ( 'NONE',  ( -63.72440971995120407, 1379.735940357757272, 269.6083204700776719 ) ) ;
#3573=DIRECTION ( 'NONE',  ( 1.836970198721029688E-16, 1.000000000000000000, -1.262177448353620010E-31 ) ) ;
#3603=CARTESIAN_POINT ( 'NONE',  ( -106.8758219270079906, 1380.995759212869871, 309.1925272263990223 ) ) ;
#3628=CARTESIAN_POINT ( 'NONE',  ( -39.33111985152770274, 1384.790562297770066, 240.9749358342589858 ) ) ;
#3630=CARTESIAN_POINT ( 'NONE',  ( -105.7427259770000063, 1378.913061773969957, 302.9732994362589693 ) ) ;
#3655=CARTESIAN_POINT ( 'NONE',  ( -62.88192661074859302, 1379.821258371850035, 270.0876200625010028 ) ) ;
#3658=CARTESIAN_POINT ( 'NONE',  ( -16.67901052306879706, 1379.616296946549937, 212.0685361777370304 ) ) ;
#3665=CARTESIAN_POINT ( 'NONE',  ( -105.3795479729999869, 1390.980567596649962, 304.2017031079589628 ) ) ;
#3689=CARTESIAN_POINT ( 'NONE',  ( -79.28273665509999546, 1377.156469662599875, 290.5424571711589579 ) ) ;
#3695=CARTESIAN_POINT ( 'NONE',  ( -106.7756681249999957, 1385.009182713600012, 297.1165651138589965 ) ) ;
#3705=CARTESIAN_POINT ( 'NONE',  ( -65.00001850430001582, 1379.749314314899948, 272.6104031607590059 ) ) ;
#3707=CARTESIAN_POINT ( 'NONE',  ( -109.9855944279999989, 1384.926148861439970, 311.4562326602589906 ) ) ;
#3711=ORIENTED_EDGE ( 'NONE', *, *, #526, .T. ) ;
#3716=CARTESIAN_POINT ( 'NONE',  ( -25.11140045820960154, 1385.255350696510050, 223.7582419935289977 ) ) ;
#3718=CIRCLE ( 'NONE', #78837, 7.513264357030008611 ) ;
#3749=CARTESIAN_POINT ( 'NONE',  ( -105.0536199400000044, 1379.378595376449994, 303.3386746932590086 ) ) ;
#3762=CARTESIAN_POINT ( 'NONE',  ( -92.91140151093370037, 1383.768484979190134, 309.3741002178249460 ) ) ;
#3763=CARTESIAN_POINT ( 'NONE',  ( -109.6813523066950182, 1383.874575646420226, 311.2769763007889878 ) ) ;
#3767=CARTESIAN_POINT ( 'NONE',  ( -106.7756681350000036, 1384.894991215109940, 297.1173194602590115 ) ) ;
#3773=CARTESIAN_POINT ( 'NONE',  ( -109.7179059649999999, 1384.924775326750023, 297.0861727099589871 ) ) ;
#3805=AXIS2_PLACEMENT_3D ( 'NONE', #47369, #8103, #110024 ) ;
#3853=CARTESIAN_POINT ( 'NONE',  ( -9.092535821413379793, 1384.806370746179937, 199.9443633485050213 ) ) ;
#3868=VECTOR ( 'NONE', #53553, 1000.000000000000000 ) ;
#3872=CARTESIAN_POINT ( 'NONE',  ( -12.31045119098629925, 1378.376187953739873, 209.7947064970520046 ) ) ;
#3875=CARTESIAN_POINT ( 'NONE',  ( -109.7216215100000056, 1385.013037790159842, 297.0870309045589579 ) ) ;
#3885=CARTESIAN_POINT ( 'NONE',  ( -19.85258526977679949, 1383.853738160929879, 220.7008533539980135 ) ) ;
#3894=CARTESIAN_POINT ( 'NONE',  ( -17.51956951369999871, 1383.856177979750100, 219.7926916635590260 ) ) ;
#3895=EDGE_CURVE ( 'NONE', #110498, #7502, #103397, .T. ) ;
#3901=CARTESIAN_POINT ( 'NONE',  ( -10.88641269510000065, 1390.488938065530192, 215.1023730057590058 ) ) ;
#3909=CARTESIAN_POINT ( 'NONE',  ( -90.62803924738049943, 1385.194695644730018, 292.9449760712819852 ) ) ;
#3911=CARTESIAN_POINT ( 'NONE',  ( -68.68489780340000550, 1379.748151576980035, 279.9908545622590168 ) ) ;
#3930=CARTESIAN_POINT ( 'NONE',  ( -8.022927361009998037, 1384.932834884869862, 218.7874485825090005 ) ) ;
#3953=CARTESIAN_POINT ( 'NONE',  ( -3.078458355199999996, 1384.777566036459802, 199.6697850883389833 ) ) ;
#3968=ORIENTED_EDGE ( 'NONE', *, *, #56195, .T. ) ;
#3981=CARTESIAN_POINT ( 'NONE',  ( -108.2868634315222067, 1380.916857273249434, 298.2057793955574425 ) ) ;
#3992=CARTESIAN_POINT ( 'NONE',  ( -81.63072053611109880, 1384.989726998269816, 304.8882203442400396 ) ) ;
#3995=EDGE_LOOP ( 'NONE', ( #51836, #93827, #100561, #103653, #100469 ) ) ;
#4021=CARTESIAN_POINT ( 'NONE',  ( -7.702631097496129620, 1383.525349896430043, 218.9204624055510067 ) ) ;
#4035=CARTESIAN_POINT ( 'NONE',  ( -88.81502644064428864, 1384.621400043609810, 308.2893549430740450 ) ) ;
#4036=CARTESIAN_POINT ( 'NONE',  ( -37.08409534967810117, 1384.983166705460008, 210.3120036977730081 ) ) ;
#4044=CARTESIAN_POINT ( 'NONE',  ( -109.4838093930000014, 1384.905744133400049, 311.2841432912590562 ) ) ;
#4052=CARTESIAN_POINT ( 'NONE',  ( -107.0252682235529988, 1391.913060387289988, 306.7492100420760153 ) ) ;
#4056=CARTESIAN_POINT ( 'NONE',  ( -11.72622114699999862, 1378.269058748980115, 205.1826066712690135 ) ) ;
#4068=CARTESIAN_POINT ( 'NONE',  ( -68.16711561486698656, 1379.746493480949994, 279.7015904451550341 ) ) ;
#4095=CARTESIAN_POINT ( 'NONE',  ( -8.023454095920000029, 1384.914900298040038, 218.7875189542389762 ) ) ;
#4098=CARTESIAN_POINT ( 'NONE',  ( -68.38408895284545963, 1379.747196019225385, 279.2321024377919798 ) ) ;
#4102=CARTESIAN_POINT ( 'NONE',  ( -55.49204166402299876, 1384.646788494520024, 234.8063369579010100 ) ) ;
#4109=CARTESIAN_POINT ( 'NONE',  ( -7.966081143649218710, 1384.918389534460175, 199.4892681243580057 ) ) ;
#4117=DIRECTION ( 'NONE',  ( 0.9991156138703696232, -3.961952592064073292E-33, -0.04204747460233797945 ) ) ;
#4136=EDGE_CURVE ( 'NONE', #61054, #22898, #54923, .T. ) ;
#4161=DIRECTION ( 'NONE',  ( 0.07285353650440702655, -0.004327861288661672377, 0.9973332601670652497 ) ) ;
#4163=CARTESIAN_POINT ( 'NONE',  ( -26.14268957564699747, 1384.842186362059920, 224.5499447472220140 ) ) ;
#4164=CARTESIAN_POINT ( 'NONE',  ( -105.1761031979999927, 1379.258906148879987, 302.7941945437589766 ) ) ;
#4182=CARTESIAN_POINT ( 'NONE',  ( -56.99285471647699808, 1379.895685281439910, 259.6123875215530461 ) ) ;
#4186=ORIENTED_EDGE ( 'NONE', *, *, #47356, .F. ) ;
#4193=CARTESIAN_POINT ( 'NONE',  ( -9.075785912040000625, 1383.961100907409900, 218.5571957096990161 ) ) ;
#4215=CARTESIAN_POINT ( 'NONE',  ( -13.72133526636149981, 1380.332343284469971, 209.6969764857090013 ) ) ;
#4219=CARTESIAN_POINT ( 'NONE',  ( -56.57961477790000515, 1375.243914315939946, 252.6055042413589717 ) ) ;
#4230=CARTESIAN_POINT ( 'NONE',  ( -22.68195036590000058, 1384.853989887049920, 222.0405270882590116 ) ) ;
#4235=CARTESIAN_POINT ( 'NONE',  ( -67.66215561869999817, 1379.745947391239952, 277.8420489690590216 ) ) ;
#4244=CARTESIAN_POINT ( 'NONE',  ( -81.17886098919998972, 1384.990453609069846, 304.9592558327589700 ) ) ;
#4247=CARTESIAN_POINT ( 'NONE',  ( -25.62888669017269905, 1385.253130175059823, 224.1332055726419981 ) ) ;
#4271=EDGE_CURVE ( 'NONE', #33840, #61557, #45293, .T. ) ;
#4279=CARTESIAN_POINT ( 'NONE',  ( -105.5774848019999865, 1391.233264612319999, 302.6220608442590105 ) ) ;
#4285=CARTESIAN_POINT ( 'NONE',  ( -105.5846564840000070, 1377.935450406140035, 304.0481634900589825 ) ) ;
#4296=EDGE_CURVE ( 'NONE', #46346, #13675, #23821, .T. ) ;
#4299=CARTESIAN_POINT ( 'NONE',  ( -108.9848104056970044, 1383.828915778130067, 311.1014354137989812 ) ) ;
#4308=CARTESIAN_POINT ( 'NONE',  ( -109.8956305769999915, 1384.931289674369964, 297.0283802634589847 ) ) ;
#4350=B_SPLINE_CURVE_WITH_KNOTS ( 'NONE', 3,
 ( #14924, #82143, #55873, #65924, #13819, #65375, #98394, #39601, #73772, #107896, #37954, #38485, #106790, #72663, #55318, #13269, #12742, #91098, #73206, #49119, #99479, #23334, #64832, #46925, #56966, #30080, #100046, #4886, #14376, #82704, #81043, #89994, #4357, #106252, #29538, #107350, #63725, #47459, #97835, #39027, #30646, #8182, #17109, #32833, #40697, #92201, #76504, #15474, #77073, #51299, #33945, #110653, #7642, #24428, #93298, #16560, #83801, #41254, #68679, #101682, #32301, #66485, #92747, #50754, #84891, #58616, #16024, #17670, #102786, #109565, #26081, #93839, #60272, #382, #68139, #23873, #74869, #7098, #59719, #109018, #84351, #102250, #24971, #100592, #42349, #25529, #94390, #50223, #33380, #41796, #75956, #110107, #49669, #85436, #67576, #83251, #59178, #58069, #67027, #75428, #8734, #42917, #34503, #6547, #101133, #63476, #97595, #52431, #9853, #38773, #70352, #928, #20866, #64015, #104464, #72949, #44575, #78719, #35051, #38226, #36168, #107085, #98126, #30374, #47195, #4102, #103342, #43471, #86557, #29829, #9308, #52982, #13009, #4635, #89188, #72409, #87114, #44021, #69233, #61394, #55061, #10404, #95515, #94967, #55612, #2035, #81321, #89735, #21402, #12481, #64564, #98683, #18236, #29281, #18785, #106540, #78157, #51872, #86008, #69795, #46663, #77616, #26644, #60842, #1468, #80796, #35602, #103913, #27213, #57809, #57269, #40427, #74052, #39333, #81875, #73506, #82444, #92472, #65653, #23626, #6279, #15207, #109847, #41544, #75700, #107641, #99770, #23059, #66219, #47740, #74603, #65103, #5177, #66766, #30925, #99215, #14113, #33124, #82987, #22493, #100338, #91396, #15742, #5742, #49943, #56694, #91933, #90830, #49398, #84081, #14673, #39885, #21944, #109304, #48304, #83524, #108181, #6818, #100866, #108739, #32030, #48861, #40977, #75157, #31472, #32590, #24157, #58347, #7379, #67311, #56137, #90272, #13554, #51597, #76241, #68971, #25257, #18510, #68417, #60568, #653, #26373, #50504, #103072, #52707, #60009, #85180, #101408, #77896, #33668, #52156, #76792, #94688, #35336, #51047, #58896, #110388, #17961, #67860, #95246, #69525, #86289, #86842, #7923, #43745, #10134, #101971, #1203, #59460, #16300, #103645, #44306, #84626, #109, #34784, #9573, #42639, #34231, #35901, #78449, #16845, #42093, #8466, #26943, #61132, #1763, #24700, #93029, #93570, #102519, #25811, #94130, #17401, #9029, #85730, #43200, #77351, #89590, #45420, #20176, #79562, #45957, #46516, #11258 ),
 .UNSPECIFIED., .F., .F.,
 ( 4, 3, 3, 3, 3, 3, 3, 3, 3, 3, 3, 3, 3, 3, 3, 3, 3, 3, 3, 3, 3, 3, 3, 3, 3, 3, 3, 3, 3, 3, 3, 3, 3, 3, 3, 3, 3, 3, 3, 3, 3, 3, 3, 3, 3, 3, 3, 3, 3, 3, 3, 3, 3, 3, 3, 3, 3, 3, 3, 3, 3, 3, 3, 3, 3, 3, 3, 3, 3, 3, 3, 3, 3, 3, 3, 3, 3, 3, 3, 3, 3, 3, 3, 3, 3, 3, 3, 3, 3, 3, 3, 3, 3, 3, 3, 3, 3, 3, 3, 3, 3, 4 ),
 ( 8.528903892709999823, 10.11079874316899918, 11.96402179552659994, 13.55545591726709986, 14.93540995916639957, 15.39383910902119901, 16.53784965764519654, 17.65533335631520018, 18.74952487047229965, 19.85344026384639804, 20.89947257251949964, 21.93049568398669891, 22.94770232675979571, 23.95212381599139917, 24.93878849665829733, 25.91622982162849809, 26.88014850494499797, 27.58084801746479542, 28.63695919667589607, 29.71615375306799933, 30.81911651081409786, 31.94529991305369521, 33.12652436437380032, 34.29236762325579946, 35.45927563792669446, 36.61824151545220474, 37.81245501749270232, 38.92511934700599596, 40.01843177764789772, 41.08438201573959958, 41.39509552361419509, 42.90409533968830402, 44.42289876441959962, 45.95738695247120376, 47.50856733623960082, 49.07757088809649559, 50.66567512639480242, 52.27433300125469628, 53.93242794869799894, 55.59996648682680132, 57.29321361784219846, 59.01465425201970305, 60.78527615218369817, 62.58728134439490276, 64.44454181919989821, 65.53909258080051359, 67.04475135045599643, 68.62894058153921151, 70.27967536058729081, 72.01761458325029253, 73.87891071221881134, 75.94929923628670565, 78.63951486550050163, 80.97143900281349715, 82.94603025408429176, 84.75425470534629824, 86.41460430148269722, 88.01672707843430032, 89.54556736663739969, 90.91108773679130195, 93.82957164518428783, 96.80547043545971064, 99.57405818404620845, 102.2141381765199952, 104.7420692361749985, 107.1759481923769926, 109.5308444734030076, 111.7884715630940065, 113.9994590479840042, 116.1473335953590009, 117.6367619673870024, 119.0967884077180088, 120.5520899153760013, 122.0392533098840175, 123.4344489772180253, 124.8001882596219900, 126.1366051610670098, 127.4449720650600142, 128.7132937358369986, 129.9615380000630012, 131.2054675357509836, 132.4493970714400177, 133.6727958913919565, 135.0110548064769773, 136.6141698558100188, 138.3143900939450077, 139.6965082775570011, 140.9764010850390150, 142.1130208664269787, 143.2066028786510117, 144.2502205449540043, 144.8160795074840053, 146.1142711068380038, 147.4422065578220042, 148.8126880694590000, 150.2044901557419792, 151.6094053898760023, 153.0744782599189762, 154.4631086672829952, 155.8325814729020067, 157.1697943162390061, 157.4696968700480113 ),
 .UNSPECIFIED. ) ;
#4357=CARTESIAN_POINT ( 'NONE',  ( -24.53717461995699978, 1384.543544838199978, 203.1111072970969929 ) ) ;
#4388=B_SPLINE_CURVE_WITH_KNOTS ( 'NONE', 5,
 ( #32962, #32430, #90110, #76090, #88222, #34630 ),
 .UNSPECIFIED., .F., .F.,
 ( 6, 6 ),
 ( -1.999999982688239974, 0.000000000000000000 ),
 .UNSPECIFIED. ) ;
#4410=CARTESIAN_POINT ( 'NONE',  ( -109.7017504620000068, 1385.317244295069941, 297.1054320267589901 ) ) ;
#4412=ORIENTED_EDGE ( 'NONE', *, *, #61891, .T. ) ;
#4423=CARTESIAN_POINT ( 'NONE',  ( -45.92082474586209884, 1383.818659492949791, 252.9957497693810069 ) ) ;
#4431=CARTESIAN_POINT ( 'NONE',  ( -39.64173303379999425, 1383.033670297620120, 212.5860353986090274 ) ) ;
#4438=CARTESIAN_POINT ( 'NONE',  ( -11.41029669623840093, 1391.349546573489988, 213.9346477860329969 ) ) ;
#4448=CARTESIAN_POINT ( 'NONE',  ( -68.33454988889999981, 1379.748399532440089, 279.2380605676589767 ) ) ;
#4459=CARTESIAN_POINT ( 'NONE',  ( -109.3962244350000077, 1384.944647467069899, 311.2791233102589672 ) ) ;
#4468=CARTESIAN_POINT ( 'NONE',  ( -8.034992631979999800, 1385.326470000059999, 218.7648172177289894 ) ) ;
#4490=CARTESIAN_POINT ( 'NONE',  ( -2.274251696913569793E-15, 1384.485850024879937, 199.6505477045689929 ) ) ;
#4492=ORIENTED_EDGE ( 'NONE', *, *, #36509, .T. ) ;
#4520=CARTESIAN_POINT ( 'NONE',  ( 0.000000000000000000, 1384.913060387289988, 209.1218459572589836 ) ) ;
#4526=CARTESIAN_POINT ( 'NONE',  ( -101.2221464535970057, 1384.943467076989918, 310.9552930315260255 ) ) ;
#4529=CARTESIAN_POINT ( 'NONE',  ( -9.481266696980000575, 1388.680743057909922, 201.1014716156689985 ) ) ;
#4553=EDGE_CURVE ( 'NONE', #23910, #49801, #58521, .T. ) ;
#4571=CARTESIAN_POINT ( 'NONE',  ( -90.82321950335810357, 1384.617696737160259, 308.9652747753909807 ) ) ;
#4572=CARTESIAN_POINT ( 'NONE',  ( -43.37668113294960648, 1384.998540390349945, 216.4009036113180002 ) ) ;
#4579=CARTESIAN_POINT ( 'NONE',  ( -109.9850615409999932, 1384.906745092810070, 311.4561455232590106 ) ) ;
#4603=CARTESIAN_POINT ( 'NONE',  ( -68.34061848820969942, 1379.747312853899984, 279.8872088319540126 ) ) ;
#4631=CARTESIAN_POINT ( 'NONE',  ( -63.44223337645949101, 1379.735152652233410, 269.0017066445272462 ) ) ;
#4635=CARTESIAN_POINT ( 'NONE',  ( -57.67880930100110248, 1384.659099901070249, 239.1381722207320024 ) ) ;
#4696=CARTESIAN_POINT ( 'NONE',  ( -40.12232014923479539, 1384.787011377809904, 242.3469171355359890 ) ) ;
#4717=CARTESIAN_POINT ( 'NONE',  ( -75.76943313550691528, 1379.211134910969804, 293.7650760281990188 ) ) ;
#4728=CARTESIAN_POINT ( 'NONE',  ( -104.4930944259999990, 1390.118374325210198, 304.1821532511589794 ) ) ;
#4744=CARTESIAN_POINT ( 'NONE',  ( -109.8576740279066115, 1385.955398400293006, 311.3643922957008385 ) ) ;
#4752=CARTESIAN_POINT ( 'NONE',  ( -56.57961477790000515, 1379.628839295709895, 252.6055042428589843 ) ) ;
#4763=CARTESIAN_POINT ( 'NONE',  ( -67.10855885389999287, 1384.077638385570026, 292.1367942583589752 ) ) ;
#4768=CARTESIAN_POINT ( 'NONE',  ( -50.74207601739999518, 1379.687644451550113, 241.2614600171590098 ) ) ;
#4775=CARTESIAN_POINT ( 'NONE',  ( -86.93157266469999911, 1384.741940548570028, 307.7299721360590183 ) ) ;
#4777=CARTESIAN_POINT ( 'NONE',  ( -26.43298866905689692, 1385.249642334559894, 224.7510168897049994 ) ) ;
#4782=CARTESIAN_POINT ( 'NONE',  ( -107.2902847454959954, 1391.913060387289988, 307.3027153792770036 ) ) ;
#4803=CARTESIAN_POINT ( 'NONE',  ( -105.5084658100000041, 1391.296568505289997, 303.1147108145589755 ) ) ;
#4828=CARTESIAN_POINT ( 'NONE',  ( -113.4000000000000057, 1379.423458858030017, 303.3195241032590275 ) ) ;
#4834=CARTESIAN_POINT ( 'NONE',  ( -1.658081806242819971E-15, 1375.886883438980021, 209.1218459572589836 ) ) ;
#4869=CARTESIAN_POINT ( 'NONE',  ( -11.15738487964140013, 1390.939238811560017, 203.8452351040699853 ) ) ;
#4886=CARTESIAN_POINT ( 'NONE',  ( -22.47842407610009730, 1384.538925626759919, 202.4009993073999851 ) ) ;
#4893=EDGE_CURVE ( 'NONE', #106524, #26498, #73231, .T. ) ;
#4900=CARTESIAN_POINT ( 'NONE',  ( -68.78495875209999610, 1379.747964692090136, 280.2437115059590269 ) ) ;
#4915=CARTESIAN_POINT ( 'NONE',  ( -9.100602447694548403, 1384.657749302420143, 199.9536881146249812 ) ) ;
#4930=CARTESIAN_POINT ( 'NONE',  ( -5.432410439650000811, 1391.426148861440197, 209.1218459572589836 ) ) ;
#4949=CARTESIAN_POINT ( 'NONE',  ( -40.03127858458480404, 1383.828107059689955, 241.8368436171929829 ) ) ;
#4959=CARTESIAN_POINT ( 'NONE',  ( -22.77753075879999756, 1378.937177693190051, 211.3942171327190067 ) ) ;
#4965=CARTESIAN_POINT ( 'NONE',  ( -12.48191901824699990, 1389.982499505159922, 213.9369507849619936 ) ) ;
#4974=CARTESIAN_POINT ( 'NONE',  ( -108.9665184055720033, 1385.242083167919873, 297.1409723503389841 ) ) ;
#4976=CARTESIAN_POINT ( 'NONE',  ( -67.96433663839999895, 1379.748578009009861, 278.4994408155590122 ) ) ;
#4984=EDGE_CURVE ( 'NONE', #6840, #23910, #66807, .T. ) ;
#4988=CARTESIAN_POINT ( 'NONE',  ( -109.8240211180000045, 1384.930942008709962, 311.3852198412590155 ) ) ;
#4993=B_SPLINE_CURVE_WITH_KNOTS ( 'NONE', 5,
 ( #19595, #71146, #87935, #54882, #49107, #71715, #12295, #96876, #2291, #80620, #5433, #45927, #45388, #105267, #20145, #80062, #54342, #70594 ),
 .UNSPECIFIED., .F., .F.,
 ( 6, 3, 3, 3, 3, 6 ),
 ( 0.000000000000000000, 0.2202946003694152555, 0.3397378414386151846, 0.5088681883646077875, 0.8372692437405104826, 1.000000000000000000 ),
 .UNSPECIFIED. ) ;
#5000=CARTESIAN_POINT ( 'NONE',  ( -8.859600949860000796, 1385.023751217870085, 218.6831814923290267 ) ) ;
#5001=CARTESIAN_POINT ( 'NONE',  ( -14.44139730133570154, 1379.629733965419973, 208.1340535457149770 ) ) ;
#5028=CONICAL_SURFACE ( 'NONE', #96245, 0.9999999999999857891, 0.7853981633970000820 ) ;
#5049=CARTESIAN_POINT ( 'NONE',  ( -109.3435511536187903, 1382.472266926233942, 297.4003323660738261 ) ) ;
#5061=CARTESIAN_POINT ( 'NONE',  ( -92.03063779543769840, 1384.964829711410175, 309.3299059855730206 ) ) ;
#5062=CARTESIAN_POINT ( 'NONE',  ( -8.618443112799999639, 1386.703020315259892, 200.0643205304990033 ) ) ;
#5105=CARTESIAN_POINT ( 'NONE',  ( -12.30373392569999957, 1378.362863315840059, 209.9037182927540073 ) ) ;
#5106=CARTESIAN_POINT ( 'NONE',  ( -107.0634112298879899, 1384.587327643060007, 311.2343609292589690 ) ) ;
#5107=CARTESIAN_POINT ( 'NONE',  ( -54.03892782705099762, 1385.034468983960096, 232.0668901380410034 ) ) ;
#5119=CARTESIAN_POINT ( 'NONE',  ( -109.4871642380000054, 1384.813187038689875, 311.2830328522589980 ) ) ;
#5141=CARTESIAN_POINT ( 'NONE',  ( -68.16062186043509996, 1379.746616918160043, 279.7065836077829886 ) ) ;
#5146=ORIENTED_EDGE ( 'NONE', *, *, #42524, .F. ) ;
#5156=PRODUCT_CONTEXT ( 'NONE', #93479, 'mechanical' ) ;
#5172=CARTESIAN_POINT ( 'NONE',  ( -68.07264245651541046, 1379.746555617447939, 278.5801731380780097 ) ) ;
#5177=CARTESIAN_POINT ( 'NONE',  ( -74.59470942271289573, 1384.765139218380000, 274.7532847296519662 ) ) ;
#5209=CARTESIAN_POINT ( 'NONE',  ( -113.4000000000000057, 1386.449969320030050, 311.2218459572590064 ) ) ;
#5215=CARTESIAN_POINT ( 'NONE',  ( -109.9659341548349971, 1384.416896023069967, 311.4329124691320203 ) ) ;
#5228=DIRECTION ( 'NONE',  ( 0.9996573249755517088, 0.02617694830808742559, 0.000000000000000000 ) ) ;
#5246=CARTESIAN_POINT ( 'NONE',  ( -29.34764347683880104, 1384.830841659480029, 227.3863593227910087 ) ) ;
#5250=CARTESIAN_POINT ( 'NONE',  ( -105.4205408459999944, 1379.023436635359985, 302.8723641076589956 ) ) ;
#5271=CARTESIAN_POINT ( 'NONE',  ( -86.54208378602990592, 1379.132636796130100, 301.6681089792259627 ) ) ;
#5274=CARTESIAN_POINT ( 'NONE',  ( -14.05185835220319923, 1379.611218837149863, 211.6671715642569893 ) ) ;
#5284=CARTESIAN_POINT ( 'NONE',  ( -8.407635077709999294, 1384.019446811960051, 218.5970489128289955 ) ) ;
#5301=CARTESIAN_POINT ( 'NONE',  ( -109.8944536047824130, 1385.812234818686193, 311.3867069332368374 ) ) ;
#5304=CARTESIAN_POINT ( 'NONE',  ( -13.19407264773069954, 1379.711643100160245, 208.4819402826470025 ) ) ;
#5308=CARTESIAN_POINT ( 'NONE',  ( -55.86512536059999690, 1374.936376805820146, 252.9328197391589867 ) ) ;
#5322=CARTESIAN_POINT ( 'NONE',  ( -89.66120661540000469, 1384.333980646620148, 308.7172663300589761 ) ) ;
#5326=CARTESIAN_POINT ( 'NONE',  ( -54.30030265850000859, 1379.725094345220214, 248.9924859156590173 ) ) ;
#5334=CARTESIAN_POINT ( 'NONE',  ( -109.9987472809999929, 1384.922094923150098, 311.2741087182590149 ) ) ;
#5335=CARTESIAN_POINT ( 'NONE',  ( -26.83711809360000089, 1388.514028352690048, 223.1242661799589939 ) ) ;
#5336=ORIENTED_EDGE ( 'NONE', *, *, #103310, .T. ) ;
#5337=CARTESIAN_POINT ( 'NONE',  ( -40.64111485381250333, 1385.178332084029762, 243.2412163901340136 ) ) ;
#5347=CARTESIAN_POINT ( 'NONE',  ( -7.968704128189949998, 1384.504568802437689, 199.5050640420236618 ) ) ;
#5364=CARTESIAN_POINT ( 'NONE',  ( -108.3356498620000110, 1388.869567454079970, 298.1379939792590221 ) ) ;
#5370=CARTESIAN_POINT ( 'NONE',  ( -105.4154991850000016, 1378.862308729909955, 303.3418524678589847 ) ) ;
#5384=CARTESIAN_POINT ( 'NONE',  ( -103.9411501300010059, 1383.761452288409828, 310.9608569221110201 ) ) ;
#5389=CARTESIAN_POINT ( 'NONE',  ( -109.9987472819999965, 1383.757409383979848, 311.0847451122589860 ) ) ;
#5420=CARTESIAN_POINT ( 'NONE',  ( -8.369575833189999869, 1384.742689880740045, 199.7789889385390154 ) ) ;
#5430=ORIENTED_EDGE ( 'NONE', *, *, #24009, .T. ) ;
#5433=CARTESIAN_POINT ( 'NONE',  ( -105.5320588160000028, 1381.208403848540001, 299.1971426474589748 ) ) ;
#5474=CARTESIAN_POINT ( 'NONE',  ( -14.08481621004247231, 1379.673254536278591, 211.5737053288229106 ) ) ;
#5478=DIRECTION ( 'NONE',  ( 1.836970198721029688E-16, 1.000000000000000000, 0.000000000000000000 ) ) ;
#5492=CARTESIAN_POINT ( 'NONE',  ( -106.4840262270000011, 1379.607751643809934, 300.2526974370589983 ) ) ;
#5501=ORIENTED_EDGE ( 'NONE', *, *, #56826, .F. ) ;
#5505=CARTESIAN_POINT ( 'NONE',  ( -113.4000000000000057, 1379.913060387289988, 304.2218459572590064 ) ) ;
#5508=B_SPLINE_CURVE_WITH_KNOTS ( 'NONE', 3,
 ( #93820, #15463, #17097, #110643 ),
 .UNSPECIFIED., .F., .F.,
 ( 4, 4 ),
 ( 0.7259150538130000330, 23.36254398669999688 ),
 .UNSPECIFIED. ) ;
#5511=CARTESIAN_POINT ( 'NONE',  ( -53.52129292230850410, 1383.806223322539836, 268.5146929885909799 ) ) ;
#5518=ORIENTED_EDGE ( 'NONE', *, *, #24049, .F. ) ;
#5520=CARTESIAN_POINT ( 'NONE',  ( -25.42483392789999641, 1381.467239109759930, 204.6897922305890063 ) ) ;
#5528=CARTESIAN_POINT ( 'NONE',  ( -8.237282586322759670, 1385.788991056809891, 218.6757492481600025 ) ) ;
#5532=CARTESIAN_POINT ( 'NONE',  ( -107.8192228660000040, 1380.324541384940176, 298.6453595191590011 ) ) ;
#5552=EDGE_CURVE ( 'NONE', #6840, #89045, #108619, .T. ) ;
#5554=FACE_OUTER_BOUND ( 'NONE', #89313, .T. ) ;
#5565=CARTESIAN_POINT ( 'NONE',  ( -14.25270368724149961, 1379.587364531829962, 207.9005521859079977 ) ) ;
#5579=CARTESIAN_POINT ( 'NONE',  ( -107.8301892023879986, 1378.913060387359792, 300.1602841119429854 ) ) ;
#5611=CARTESIAN_POINT ( 'NONE',  ( -109.0700496325590194, 1382.022296823163288, 297.5851204363052602 ) ) ;
#5624=CARTESIAN_POINT ( 'NONE',  ( -90.41568981223930734, 1384.968564493010035, 308.8481792632660472 ) ) ;
#5626=CARTESIAN_POINT ( 'NONE',  ( -8.184850705000000559, 1385.671368857289963, 199.6841148114490068 ) ) ;
#5640=CARTESIAN_POINT ( 'NONE',  ( -109.6028426828606541, 1386.884535610056219, 297.2361425596885738 ) ) ;
#5667=CARTESIAN_POINT ( 'NONE',  ( -105.3305948020004763, 1381.132964647196104, 308.7816990702884254 ) ) ;
#5674=CARTESIAN_POINT ( 'NONE',  ( -14.31906252709999983, 1380.323795378420073, 209.9058135456940022 ) ) ;
#5676=CARTESIAN_POINT ( 'NONE',  ( -49.73786273469480790, 1385.018151718609943, 224.8464017876140133 ) ) ;
#5706=CARTESIAN_POINT ( 'NONE',  ( -68.62400269330709079, 1379.747572044880144, 280.2354522863200259 ) ) ;
#5710=CARTESIAN_POINT ( 'NONE',  ( -8.799867317537470868, 1381.167308713387229, 217.8608335803399143 ) ) ;
#5719=CARTESIAN_POINT ( 'NONE',  ( -106.5054120343349808, 1378.913060387289988, 306.4287628433619943 ) ) ;
#5742=CARTESIAN_POINT ( 'NONE',  ( -78.64846761883408988, 1384.787391290499954, 281.2434142473900351 ) ) ;
#5772=CARTESIAN_POINT ( 'NONE',  ( -106.4193210029999932, 1386.474088513239849, 311.3161121332589687 ) ) ;
#5775=CARTESIAN_POINT ( 'NONE',  ( -8.371350849009999706, 1384.898375639480037, 199.7750114592789998 ) ) ;
#5780=CARTESIAN_POINT ( 'NONE',  ( -65.55053502199999116, 1379.787846393009886, 274.7583384239589464 ) ) ;
#5810=CARTESIAN_POINT ( 'NONE',  ( -108.6616353267809956, 1383.758284946439971, 311.0749865448200353 ) ) ;
#5813=CARTESIAN_POINT ( 'NONE',  ( -56.61892686578349299, 1384.709670891599899, 274.9079990654900030 ) ) ;
#5817=CARTESIAN_POINT ( 'NONE',  ( -106.0599097820000054, 1379.082397735959830, 301.3386546664589787 ) ) ;
#5827=CARTESIAN_POINT ( 'NONE',  ( -12.88197598446049952, 1379.383856360359914, 211.4143069029759943 ) ) ;
#5837=CARTESIAN_POINT ( 'NONE',  ( -11.18060534273650042, 1378.990352783300068, 211.8621521335040256 ) ) ;
#5864=CARTESIAN_POINT ( 'NONE',  ( -108.4554037492093812, 1388.504189957043081, 310.3907579481389121 ) ) ;
#5866=CARTESIAN_POINT ( 'NONE',  ( -13.86945421516830024, 1379.876352634179966, 208.3687925243430072 ) ) ;
#5867=ORIENTED_EDGE ( 'NONE', *, *, #25998, .F. ) ;
#5870=CARTESIAN_POINT ( 'NONE',  ( -55.15130194409999831, 1374.936376805820146, 253.2598301361589961 ) ) ;
#5881=CARTESIAN_POINT ( 'NONE',  ( -62.08642864540000517, 1384.386629093810143, 284.7566818690589798 ) ) ;
#5893=CARTESIAN_POINT ( 'NONE',  ( -49.90786910739999627, 1388.283118323920007, 226.7687942016589773 ) ) ;
#5895=CARTESIAN_POINT ( 'NONE',  ( -52.00221346620590168, 1385.110007062809927, 265.8307340536850347 ) ) ;
#5924=CARTESIAN_POINT ( 'NONE',  ( -107.3811602000000107, 1388.471954844699894, 298.6581246683589939 ) ) ;
#5926=CARTESIAN_POINT ( 'NONE',  ( -106.3262284460000018, 1391.611664250580134, 301.2004810296590449 ) ) ;
#5942=EDGE_CURVE ( 'NONE', #67300, #78937, #106545, .T. ) ;
#5945=CARTESIAN_POINT ( 'NONE',  ( -113.4000000000000057, 1380.809950924229952, 299.4484696716589838 ) ) ;
#5973=CARTESIAN_POINT ( 'NONE',  ( -8.846250282050000635, 1384.840587597319882, 199.9252785036290163 ) ) ;
#6003=CARTESIAN_POINT ( 'NONE',  ( -13.83438311809999810, 1379.888128081619925, 206.0089139935990090 ) ) ;
#6022=DIRECTION ( 'NONE',  ( 1.836970198721029688E-16, 1.000000000000000000, -1.793662034335764721E-47 ) ) ;
#6043=CARTESIAN_POINT ( 'NONE',  ( -109.1656546792999904, 1384.956445601399992, 297.1328575267269798 ) ) ;
#6055=DIRECTION ( 'NONE',  ( -1.000000000000000000, 0.000000000000000000, 0.000000000000000000 ) ) ;
#6060=CARTESIAN_POINT ( 'NONE',  ( -48.06877316588859372, 1383.815103002690194, 257.3679311951680120 ) ) ;
#6068=CARTESIAN_POINT ( 'NONE',  ( -27.74315420650000164, 1383.844892876249787, 225.5041886164589755 ) ) ;
#6072=CARTESIAN_POINT ( 'NONE',  ( -7.726443128496979895, 1385.956550061749795, 218.9144042117120250 ) ) ;
#6078=CARTESIAN_POINT ( 'NONE',  ( -104.5771061929999917, 1379.756820536730174, 302.9490267888589869 ) ) ;
#6094=CARTESIAN_POINT ( 'NONE',  ( -108.2808028870000072, 1386.465776205880047, 310.9170304772590043 ) ) ;
#6103=CARTESIAN_POINT ( 'NONE',  ( -14.20352129384949968, 1379.588683704130062, 207.8472577655950033 ) ) ;
#6115=CARTESIAN_POINT ( 'NONE',  ( -107.9362316764580072, 1378.913060387339783, 300.0379977988180258 ) ) ;
#6119=ORIENTED_EDGE ( 'NONE', *, *, #25408, .T. ) ;
#6121=CARTESIAN_POINT ( 'NONE',  ( -62.45667138380000694, 1385.073369564110180, 249.3006260568589880 ) ) ;
#6146=B_SPLINE_SURFACE_WITH_KNOTS ( 'NONE', 5, 5, ( 
 ( #94017, #8906, #50391, #66648, #41429, #92357, #59894, #85059, #23505 ),
 ( #8350, #24586, #42514, #76673, #40863, #110267, #85606, #31909, #110823 ),
 ( #58779, #66098, #83412, #25696, #34116, #68306, #76126, #84519, #49283 ),
 ( #100224, #93457, #24035, #102414, #33544, #17282, #25144, #57697, #41974 ),
 ( #6707, #67742, #100750, #51475, #15090, #16189, #74493, #109190, #108621 ),
 ( #91811, #32475, #75039, #109726, #59349, #7807, #33003, #58233, #16728 ),
 ( #75595, #92917, #15629, #101851, #49836, #7265, #83965, #67189, #101290 ),
 ( #95136, #544, #54261, #62113, #88388, #43083, #60446, #19514, #96798 ),
 ( #77785, #61009, #69964, #17838, #71070, #43635, #1095, #26823, #18397 ),
 ( #78333, #86730, #45306, #70518, #96237, #104633, #52595, #27930, #10021 ),
 ( #77244, #53719, #44752, #52041, #1645, #87856, #44191, #9470, #61554 ),
 ( #35223, #79444, #2755, #11144, #34668, #27372, #104078, #26258, #35781 ) ),
 .UNSPECIFIED., .F., .F., .F.,
 ( 6, 3, 3, 6 ),
 ( 6, 3, 6 ),
 ( 33.18405829000000296, 37.67969033829999859, 42.57359936619999985, 50.39824048690000069 ),
 ( 0.000000000000000000, 1.000000000000000000, 2.000000000000000000 ),
 .UNSPECIFIED. ) ;
#6149=TOROIDAL_SURFACE ( 'NONE', #7909, 11.34254167809999991, 1.000000000000000000 ) ;
#6152=CARTESIAN_POINT ( 'NONE',  ( -105.7010335431549919, 1391.686106122180036, 304.9005242218860303 ) ) ;
#6154=B_SPLINE_CURVE_WITH_KNOTS ( 'NONE', 3,
 ( #85637, #17871, #86758, #93487, #52621, #52069, #67222, #77811, #86202, #9493, #85088, #16757, #43660, #10047, #69436, #42003, #44220, #33032, #24611, #92945, #50420, #76151, #16217, #8379, #76700, #7834, #33575, #67767, #54292, #55379, #62711, #97360, #21172, #104109, #3885, #36352, #19544, #20629, #71665, #96830, #45881, #80018, #11176, #79475, #54833, #3339, #37463, #36904, #105785, #29068, #2784, #88957, #63251, #12249, #71099, #46438, #80570, #69994, #27397, #38016, #72196, #87885, #20099, #105223, #28510, #78363, #53175, #106316, #27958, #53752, #29598, #70544, #45336, #11708, #63783, #97900, #89511, #61580, #88418, #12802, #1671, #62141, #95712, #18978, #35812, #87317, #10612, #44781, #78931, #2238, #104661, #96267, #48073, #74942, #109089, #64335, #100653, #30143, #107962, #22834, #55929, #90049, #99550, #58134, #4949, #98458, #31259, #31810, #14989, #40213, #91166, #73835, #23939, #6611, #72727, #65439, #90608, #106851, #46982, #13887, #14441, #82205, #21727, #40763, #48638, #39667, #32370, #57040, #4423, #92267, #81106, #82767, #30705, #65999, #6060, #66551, #22275, #74393, #56476, #13332, #38548, #98998, #39091, #108519, #47523, #100118, #81645, #23403, #57591, #91715, #73269, #107409, #49186, #64891, #83315, #5511, #59790, #84423, #51367, #446, #109629, #110724, #34567, #69302, #41325, #51935, #7708, #67645, #68752, #8800, #34013, #93909, #68208, #60907, #84955, #35121, #32900, #102311, #59244, #8247, #42415, #101198, #76570, #16088, #102855, #110173, #50825, #101754, #58683, #93363, #25598, #86077, #15537, #9373, #43536, #49735, #41867, #94456, #83864, #26713, #33445, #7167, #17734, #25042, #75495, #77681, #993, #26151, #16628, #76020, #60339, #103409, #17177, #85503, #24494, #67095, #42982, #77141, #92817, #50295, #1538, #36231, #20506, #46320, #105659, #53613, #11037, #27832, #45204, #71538, #79345, #70977, #96701, #72078, #10476, #12127, #105092, #52495, #63133, #11586, #45762, #70416, #80449, #36784, #19972, #79899, #62584, #37896, #28382, #95583, #54715, #28944, #61457, #86624, #104536, #44647, #97234, #88842, #87186, #54166, #106192, #27273, #78227, #62013, #96133, #3762, #3212, #2657, #19411, #29474, #88291, #37341, #95033, #87755, #18302, #9917, #44089, #78789, #35672, #69859, #103978, #18851, #53048, #2103, #107289, #64773, #5384, #98883, #65310, #82078, #49060, #57468, #12682, #22150, #73715 ),
 .UNSPECIFIED., .F., .F.,
 ( 4, 3, 3, 3, 3, 3, 3, 3, 3, 3, 3, 3, 3, 3, 3, 3, 3, 3, 3, 3, 3, 3, 3, 3, 3, 3, 3, 3, 3, 3, 3, 3, 3, 3, 3, 3, 3, 3, 3, 3, 3, 3, 3, 3, 3, 3, 3, 3, 3, 3, 3, 3, 3, 3, 3, 3, 3, 3, 3, 3, 3, 3, 3, 3, 3, 3, 3, 3, 3, 3, 3, 3, 3, 3, 3, 3, 3, 3, 3, 3, 3, 3, 3, 3, 3, 3, 3, 3, 3, 3, 3, 3, 3, 3, 3, 3, 3, 3, 4 ),
 ( 9.791890430535840295, 11.09285369171509927, 12.23580266145529905, 13.32189124266249891, 14.35786517582680055, 15.39383910899119989, 16.43170384348270119, 17.51424454637329831, 18.65578198009049871, 19.94097596983310083, 21.40871796212839939, 23.18825047988780241, 24.57707236516490212, 25.82694388649679951, 26.96416132553860123, 27.58084801741189906, 28.69213975917609716, 29.83228324127160036, 31.00605439822959752, 32.21975478572630180, 33.50968302461040338, 34.86206544079449543, 36.29158701301099654, 37.84399942373840275, 39.41521477598699619, 40.90066773311090742, 41.39509552353548827, 43.78336362953579908, 46.21013510696290894, 48.47057239092100644, 50.60413741464040527, 52.51664332244290279, 54.35176539055790101, 56.12437305792799691, 57.84500552525899764, 59.52142888499740536, 61.14147335462639887, 62.73422932219951065, 64.28850022341509884, 65.53909258067669441, 67.16750662264719551, 68.87443876010290467, 70.68916954752430115, 72.66968054463819726, 75.04465672271381038, 77.84631887446640519, 79.90746703447679522, 81.76360575179620582, 83.49913842151880772, 85.15038425320570070, 86.70972796428270613, 88.22871214351719971, 89.69423399335190084, 90.91108773661989062, 92.83291460103269799, 94.80415031745300780, 96.80839894437879423, 98.81724224162638848, 100.7996825303579982, 102.7346356577239987, 104.5974014464039925, 106.3969924060370005, 108.1506441523539905, 109.8627096898800062, 111.5372853772309867, 113.1614624162640013, 114.7605425252640003, 116.3232191975509977, 117.6367619671650004, 119.0824689242389951, 120.5712865488890060, 122.0980518405219897, 123.6174000461700047, 125.1072950620849724, 126.5560501033809970, 128.0293868453329935, 129.3730365330290226, 130.6858248218609901, 131.9587287906659867, 132.4493970711910151, 133.5505940240470011, 134.6525636770870165, 135.7548240709300273, 136.8874810004660105, 137.9883391253270020, 139.0879140777240082, 140.1858124869349922, 141.2816593830939951, 142.3738793671560074, 143.4636526237109990, 144.5496010613929911, 144.8160795072120095, 146.5657509711560067, 148.3964307047820057, 150.2900657918840182, 152.1597978627970065, 153.9625895061970198, 155.6511879984489894, 157.1997893379999880 ),
 .UNSPECIFIED. ) ;
#6161=CARTESIAN_POINT ( 'NONE',  ( -101.9070034985570032, 1384.941843689829966, 311.0171509276760275 ) ) ;
#6163=CARTESIAN_POINT ( 'NONE',  ( -9.923943078109999760, 1386.701148096399947, 200.5013422001489687 ) ) ;
#6201=CARTESIAN_POINT ( 'NONE',  ( -103.8994048364797038, 1380.124163244008969, 306.1807731449942480 ) ) ;
#6209=CARTESIAN_POINT ( 'NONE',  ( -59.88312530457670135, 1385.060781597019968, 243.7364172681270134 ) ) ;
#6221=CARTESIAN_POINT ( 'NONE',  ( -109.6586398049999929, 1384.698294257620091, 311.3175481042590036 ) ) ;
#6222=DIRECTION ( 'NONE',  ( -0.02359658529091402182, 0.000000000000000000, 0.9997215618173935781 ) ) ;
#6227=CARTESIAN_POINT ( 'NONE',  ( -13.54126559747050074, 1379.893680670693811, 213.5390542146629684 ) ) ;
#6240=CARTESIAN_POINT ( 'NONE',  ( -68.56276905719998638, 1379.747764319660064, 280.1490247721590094 ) ) ;
#6243=CARTESIAN_POINT ( 'NONE',  ( -7.769784805680000517, 1383.283764732429972, 218.8591787099389876 ) ) ;
#6277=CARTESIAN_POINT ( 'NONE',  ( -10.94175501169999976, 1391.017587509790019, 214.8528411101989661 ) ) ;
#6279=CARTESIAN_POINT ( 'NONE',  ( -69.86210931808770397, 1384.736379523699952, 265.6221797416770301 ) ) ;
#6283=ORIENTED_EDGE ( 'NONE', *, *, #8891, .F. ) ;
#6303=ORIENTED_EDGE ( 'NONE', *, *, #22691, .T. ) ;
#6307=CARTESIAN_POINT ( 'NONE',  ( -113.4000000000000057, 1378.913060387289988, 304.2218459572590064 ) ) ;
#6333=CARTESIAN_POINT ( 'NONE',  ( -9.068330085084843617, 1389.039739579077832, 217.5674789938883293 ) ) ;
#6336=DIRECTION ( 'NONE',  ( -1.836970198721029688E-16, -1.000000000000000000, 0.000000000000000000 ) ) ;
#6343=EDGE_CURVE ( 'NONE', #110657, #68857, #33541, .T. ) ;
#6350=CARTESIAN_POINT ( 'NONE',  ( -44.91925906889510145, 1384.764579480920020, 251.3795836030480189 ) ) ;
#6356=CIRCLE ( 'NONE', #52821, 0.9999999999999956701 ) ;
#6368=CARTESIAN_POINT ( 'NONE',  ( -12.17177947439780006, 1377.637977345770196, 211.0179508916049826 ) ) ;
#6378=CARTESIAN_POINT ( 'NONE',  ( -18.28964772222979818, 1379.850932135969970, 212.2591649744949791 ) ) ;
#6380=CARTESIAN_POINT ( 'NONE',  ( -54.31440902440569829, 1379.704595983870149, 254.1403834083770334 ) ) ;
#6389=CARTESIAN_POINT ( 'NONE',  ( -2.541451598548929826E-15, 1375.913060387289988, 209.1218459572589836 ) ) ;
#6410=CARTESIAN_POINT ( 'NONE',  ( -109.5086524770909762, 1386.853415303551856, 311.1534610470823168 ) ) ;
#6412=CARTESIAN_POINT ( 'NONE',  ( -14.53481814003150063, 1379.710746619959991, 208.2793821099419915 ) ) ;
#6418=CARTESIAN_POINT ( 'NONE',  ( -51.56180980459999574, 1379.702544246149955, 241.8087128069590221 ) ) ;
#6428=ORIENTED_EDGE ( 'NONE', *, *, #31071, .T. ) ;
#6431=CARTESIAN_POINT ( 'NONE',  ( -36.11870846930000312, 1384.478883252080095, 235.4680142451589973 ) ) ;
#6445=CARTESIAN_POINT ( 'NONE',  ( -64.47258353809999676, 1386.692755172200123, 254.0625783103589868 ) ) ;
#6447=CARTESIAN_POINT ( 'NONE',  ( -43.14998543848509627, 1385.163626048319884, 247.9000986097850046 ) ) ;
#6470=CARTESIAN_POINT ( 'NONE',  ( -104.5812090319999896, 1389.496436508050010, 300.7817575048589447 ) ) ;
#6472=CARTESIAN_POINT ( 'NONE',  ( -105.6984031270000060, 1391.691901357969982, 303.4437319069589876 ) ) ;
#6489=ADVANCED_FACE ( 'NONE', ( #25185 ), #908, .F. ) ;
#6492=VERTEX_POINT ( 'NONE', #15131 ) ;
#6516=CARTESIAN_POINT ( 'NONE',  ( -110.0636332773229924, 1384.926148836659877, 296.9511394268049571 ) ) ;
#6533=ADVANCED_FACE ( 'NONE', ( #41472, #101331 ), #24621, .F. ) ;
#6547=CARTESIAN_POINT ( 'NONE',  ( -48.74781190723079760, 1384.614220091390052, 223.3886898673410144 ) ) ;
#6556=CARTESIAN_POINT ( 'NONE',  ( -14.17772861730700207, 1379.591530685439920, 207.8208986668599891 ) ) ;
#6561=CARTESIAN_POINT ( 'NONE',  ( -68.78255321330000527, 1379.747970357369923, 280.2961343352589552 ) ) ;
#6572=FACE_OUTER_BOUND ( 'NONE', #78820, .T. ) ;
#6611=CARTESIAN_POINT ( 'NONE',  ( -42.25319127006149955, 1383.824624454990044, 245.8538586339880112 ) ) ;
#6619=CARTESIAN_POINT ( 'NONE',  ( -50.83427392639999454, 1384.622306023270085, 226.1831986462590010 ) ) ;
#6629=CARTESIAN_POINT ( 'NONE',  ( -107.7291480230000076, 1380.506275884730030, 298.7287515308590287 ) ) ;
#6648=CARTESIAN_POINT ( 'NONE',  ( -109.9855944269999952, 1384.926148861439970, 311.4562326602589906 ) ) ;
#6676=ORIENTED_EDGE ( 'NONE', *, *, #54836, .T. ) ;
#6677=CARTESIAN_POINT ( 'NONE',  ( -68.70832551159999468, 1385.106080149109857, 263.4315270082590246 ) ) ;
#6707=CARTESIAN_POINT ( 'NONE',  ( -11.18595519959999862, 1378.367123367120030, 214.3754839606289977 ) ) ;
#6713=CARTESIAN_POINT ( 'NONE',  ( -107.6372536681080021, 1384.927886973209979, 311.2581927475170005 ) ) ;
#6714=CARTESIAN_POINT ( 'NONE',  ( -9.778401456010000103, 1386.774025706429939, 200.5312082851889954 ) ) ;
#6742=CARTESIAN_POINT ( 'NONE',  ( -109.5354675709999981, 1384.888714447859911, 297.1231980247589490 ) ) ;
#6744=CARTESIAN_POINT ( 'NONE',  ( -5.444242866291430616, 1391.534755755089918, 203.3364090815709915 ) ) ;
#6746=CARTESIAN_POINT ( 'NONE',  ( -104.0047667647111780, 1380.199657110949147, 306.4945035597083347 ) ) ;
#6752=CARTESIAN_POINT ( 'NONE',  ( -13.62224074200000068, 1380.247549972129946, 210.4815130236790139 ) ) ;
#6754=CARTESIAN_POINT ( 'NONE',  ( -56.94461646417340717, 1385.046987227980026, 237.6273277843820040 ) ) ;
#6765=CARTESIAN_POINT ( 'NONE',  ( -109.6535179219999918, 1384.622105623380094, 311.3127935212589819 ) ) ;
#6783=CARTESIAN_POINT ( 'NONE',  ( -68.71522126961548338, 1379.747817121739899, 280.3072533349409809 ) ) ;
#6785=CARTESIAN_POINT ( 'NONE',  ( -12.02612939183720009, 1377.659857216290220, 211.7505375168460091 ) ) ;
#6787=( GEOMETRIC_REPRESENTATION_CONTEXT ( 3 ) GLOBAL_UNCERTAINTY_ASSIGNED_CONTEXT ( ( #62554 ) ) GLOBAL_UNIT_ASSIGNED_CONTEXT ( ( #41521, #76220, #93548 ) ) REPRESENTATION_CONTEXT ( 'NONE', 'WORKASPACE' ) );
#6817=CARTESIAN_POINT ( 'NONE',  ( -10.07692313350000113, 1391.913060387289988, 214.3555494166390076 ) ) ;
#6818=CARTESIAN_POINT ( 'NONE',  ( -82.75703543348309665, 1384.807624658469877, 286.4509065024590200 ) ) ;
#6840=VERTEX_POINT ( 'NONE', #43364 ) ;
#6853=CARTESIAN_POINT ( 'NONE',  ( -109.9672919399559987, 1384.428774922700086, 311.4339036070600173 ) ) ;
#6857=DIRECTION ( 'NONE',  ( -6.162707975952100561E-15, -1.000000000000000000, -1.094450614310000083E-14 ) ) ;
#6872=CARTESIAN_POINT ( 'NONE',  ( -8.903760273451595708, 1388.803743861253452, 217.7495020015849434 ) ) ;
#6891=CARTESIAN_POINT ( 'NONE',  ( -49.76313179303890166, 1384.741186450630039, 261.2525457107669808 ) ) ;
#6892=CARTESIAN_POINT ( 'NONE',  ( -107.1386201206849904, 1391.913060387289988, 301.4226135078189941 ) ) ;
#6900=CARTESIAN_POINT ( 'NONE',  ( -9.709241970235968466, 1380.610007537143929, 201.4292193300254326 ) ) ;
#6915=CARTESIAN_POINT ( 'NONE',  ( -9.094910673856409389, 1384.931050598509955, 199.9427862989620053 ) ) ;
#6921=CARTESIAN_POINT ( 'NONE',  ( -41.40576702097160222, 1380.117442311619925, 227.6002273774099933 ) ) ;
#6923=CARTESIAN_POINT ( 'NONE',  ( -29.73889674292890106, 1379.618472333520003, 218.1103683386099874 ) ) ;
#6938=( NAMED_UNIT ( * ) PLANE_ANGLE_UNIT ( ) SI_UNIT ( $, .RADIAN. ) );
#6951=CARTESIAN_POINT ( 'NONE',  ( -108.9749535673422116, 1387.771090604488109, 310.7965837917592467 ) ) ;
#6959=CARTESIAN_POINT ( 'NONE',  ( -7.611657828400000270, 1376.295363933120143, 206.9293838565190242 ) ) ;
#6972=CARTESIAN_POINT ( 'NONE',  ( -86.94413116030000310, 1384.337889815429889, 307.7010151988590110 ) ) ;
#6987=CARTESIAN_POINT ( 'NONE',  ( -57.13410461910000038, 1390.772211217349877, 257.4385327720589771 ) ) ;
#6989=CARTESIAN_POINT ( 'NONE',  ( -44.92722774579330292, 1385.152941095250071, 251.3752464619300042 ) ) ;
#6998=CARTESIAN_POINT ( 'NONE',  ( -7.544733521170000401, 1384.899971913130003, 219.0877090843589770 ) ) ;
#7018=CARTESIAN_POINT ( 'NONE',  ( -108.7811652620000018, 1387.776015447450163, 297.7301139582590395 ) ) ;
#7026=B_SPLINE_CURVE_WITH_KNOTS ( 'NONE', 5,
 ( #86304, #104763, #105314, #44321, #45433, #28048, #96364, #19643, #53846, #2881, #87983, #79577 ),
 .UNSPECIFIED., .F., .F.,
 ( 6, 3, 3, 6 ),
 ( 0.000000000000000000, 0.5093891872483979899, 0.7698042424308239040, 1.000000000000000000 ),
 .UNSPECIFIED. ) ;
#7047=CARTESIAN_POINT ( 'NONE',  ( -8.861482052969998691, 1384.950957082100103, 218.6848127019790127 ) ) ;
#7053=CARTESIAN_POINT ( 'NONE',  ( -44.32302097390000029, 1380.083786706710043, 232.1686497034590104 ) ) ;
#7074=CARTESIAN_POINT ( 'NONE',  ( -8.156254627529998302, 1384.896657259020003, 199.6468325161289954 ) ) ;
#7093=CARTESIAN_POINT ( 'NONE',  ( -109.5441724459999904, 1379.129497135580095, 302.6503169382589817 ) ) ;
#7098=CARTESIAN_POINT ( 'NONE',  ( -40.95419143721069588, 1384.585776280029904, 213.8410145222069900 ) ) ;
#7167=CARTESIAN_POINT ( 'NONE',  ( -68.31774780045299167, 1383.786899405800114, 292.8199513039460271 ) ) ;
#7177=CARTESIAN_POINT ( 'NONE',  ( -53.33610125319999895, 1383.102638364699942, 230.8253073736590011 ) ) ;
#7188=CARTESIAN_POINT ( 'NONE',  ( -106.8622583199999951, 1380.214950530570150, 299.5452633442590127 ) ) ;
#7196=CARTESIAN_POINT ( 'NONE',  ( -12.02612939183720009, 1377.659857216290220, 211.7505375168460091 ) ) ;
#7209=CARTESIAN_POINT ( 'NONE',  ( -108.5111915540000069, 1387.700385856930097, 310.5423399582590491 ) ) ;
#7236=CARTESIAN_POINT ( 'NONE',  ( -50.84508920509999541, 1384.755135372010045, 226.1764230024589892 ) ) ;
#7245=CARTESIAN_POINT ( 'NONE',  ( -10.80488858036439836, 1391.913060387170162, 205.5034207131209882 ) ) ;
#7265=CARTESIAN_POINT ( 'NONE',  ( -11.52159655330000021, 1380.583467895319927, 215.6172400537489864 ) ) ;
#7272=CARTESIAN_POINT ( 'NONE',  ( -12.84952252529999939, 1390.894616655729806, 209.7716342346369913 ) ) ;
#7277=CARTESIAN_POINT ( 'NONE',  ( -8.861333410889999485, 1384.870662623839962, 218.6848950059789729 ) ) ;
#7287=AXIS2_PLACEMENT_3D ( 'NONE', #9205, #94857, #34942 ) ;
#7306=CARTESIAN_POINT ( 'NONE',  ( -109.8952781789999875, 1384.897890919899965, 297.0284440182589947 ) ) ;
#7311=CARTESIAN_POINT ( 'NONE',  ( -103.6636288076488341, 1379.952131678016485, 305.1582356039069737 ) ) ;
#7318=CARTESIAN_POINT ( 'NONE',  ( -53.14982994521080428, 1385.030877996189929, 230.4728250025019918 ) ) ;
#7320=CARTESIAN_POINT ( 'NONE',  ( -11.66275644280949919, 1391.913060387289988, 209.7846402079380255 ) ) ;
#7322=ORIENTED_EDGE ( 'NONE', *, *, #96614, .F. ) ;
#7330=CARTESIAN_POINT ( 'NONE',  ( -109.9814243290000064, 1384.586435984209857, 311.4451819562590345 ) ) ;
#7343=CARTESIAN_POINT ( 'NONE',  ( -109.1321617031399995, 1384.741658746849907, 311.2608059278249470 ) ) ;
#7345=CARTESIAN_POINT ( 'NONE',  ( -68.61213284361410558, 1379.747544145440088, 280.2245858376650176 ) ) ;
#7357=SURFACE_STYLE_FILL_AREA ( #76768 ) ;
#7364=CARTESIAN_POINT ( 'NONE',  ( -120.2678896395927666, 1379.913060387289988, 304.3291340586740716 ) ) ;
#7378=CARTESIAN_POINT ( 'NONE',  ( -12.18027861210000040, 1391.555521559479985, 211.6651143923290306 ) ) ;
#7379=CARTESIAN_POINT ( 'NONE',  ( -85.67554441382009145, 1384.820767901929912, 289.3504411783320052 ) ) ;
#7397=CARTESIAN_POINT ( 'NONE',  ( -65.11626332599999500, 1379.739664436940075, 272.5544191705590151 ) ) ;
#7449=CARTESIAN_POINT ( 'NONE',  ( -44.38402502188429821, 1384.767141598809758, 250.3222099174190021 ) ) ;
#7450=CARTESIAN_POINT ( 'NONE',  ( -106.6236903171660089, 1391.913060387289988, 302.6845673397129985 ) ) ;
#7452=CARTESIAN_POINT ( 'NONE',  ( -107.1425330629999877, 1379.500016098490050, 299.4908666160590087 ) ) ;
#7456=CARTESIAN_POINT ( 'NONE',  ( -9.730454605791324596, 1380.582231750482379, 201.4572460339118436 ) ) ;
#7465=CARTESIAN_POINT ( 'NONE',  ( -12.32144544124709995, 1378.870868370589960, 211.6518144768560035 ) ) ;
#7476=CARTESIAN_POINT ( 'NONE',  ( -3.771520276259990201, 1377.996768148150068, 211.7927965281820093 ) ) ;
#7479=CARTESIAN_POINT ( 'NONE',  ( -40.65834370721180591, 1379.654954877820046, 229.2787104343509839 ) ) ;
#7494=( NAMED_UNIT ( * ) SI_UNIT ( $, .STERADIAN. ) SOLID_ANGLE_UNIT ( ) );
#7502=VERTEX_POINT ( 'NONE', #106412 ) ;
#7511=CARTESIAN_POINT ( 'NONE',  ( -11.40322695539999920, 1375.342188321910044, 209.3118815522890088 ) ) ;
#7527=CARTESIAN_POINT ( 'NONE',  ( -113.4000000000000057, 1384.574445395800012, 311.2057750932590352 ) ) ;
#7541=CARTESIAN_POINT ( 'NONE',  ( -56.97380248630000210, 1389.509217074559956, 269.0144898038590213 ) ) ;
#7542=ORIENTED_EDGE ( 'NONE', *, *, #86442, .T. ) ;
#7543=CARTESIAN_POINT ( 'NONE',  ( -51.29381094165059807, 1385.114229371170040, 264.3850473588399836 ) ) ;
#7544=AXIS2_PLACEMENT_3D ( 'NONE', #45884, #2787, #35815 ) ;
#7568=CARTESIAN_POINT ( 'NONE',  ( -108.7478840269999978, 1386.424881223649891, 297.4056966952589960 ) ) ;
#7598=ADVANCED_FACE ( 'NONE', ( #85596 ), #95679, .F. ) ;
#7599=CARTESIAN_POINT ( 'NONE',  ( -12.29413384569110157, 1378.302811799279880, 210.0202395160829951 ) ) ;
#7616=CARTESIAN_POINT ( 'NONE',  ( -9.104938183539999841, 1384.618211218890110, 199.9573581933690036 ) ) ;
#7634=CARTESIAN_POINT ( 'NONE',  ( -109.5441724399999970, 1379.437034645699896, 304.2218460466590386 ) ) ;
#7642=CARTESIAN_POINT ( 'NONE',  ( -31.76456352044490572, 1384.560446604800063, 206.5901853932080030 ) ) ;
#7649=CARTESIAN_POINT ( 'NONE',  ( -18.22628348410981047, 1379.600014138350616, 212.7175748282816414 ) ) ;
#7651=CARTESIAN_POINT ( 'NONE',  ( -10.73113664029999903, 1382.357287394640252, 201.1356155892590039 ) ) ;
#7655=CARTESIAN_POINT ( 'NONE',  ( -68.30075113750000071, 1379.746851987089940, 279.1016318162590437 ) ) ;
#7673=EDGE_CURVE ( 'NONE', #109170, #48273, #85146, .T. ) ;
#7688=FACE_OUTER_BOUND ( 'NONE', #89830, .T. ) ;
#7691=DIRECTION ( 'NONE',  ( 1.000000000000000000, 0.000000000000000000, 0.000000000000000000 ) ) ;
#7708=CARTESIAN_POINT ( 'NONE',  ( -56.45588150975670061, 1383.801723053599972, 274.2314575997830275 ) ) ;
#7716=CARTESIAN_POINT ( 'NONE',  ( -51.11582849079999846, 1379.961985591460007, 254.5469988028590365 ) ) ;
#7718=ORIENTED_EDGE ( 'NONE', *, *, #56962, .F. ) ;
#7721=CARTESIAN_POINT ( 'NONE',  ( -8.747709872648618656, 1385.329978680540080, 218.6507686934189962 ) ) ;
#7723=DIRECTION ( 'NONE',  ( 5.497413460834789123E-05, 0.09152419561177496665, -0.9958028512689959255 ) ) ;
#7726=CARTESIAN_POINT ( 'NONE',  ( -107.4285199579999954, 1381.409267714380121, 298.6311223556590448 ) ) ;
#7749=CARTESIAN_POINT ( 'NONE',  ( -106.1392238060000039, 1388.866019527689787, 308.9234258288589672 ) ) ;
#7780=VERTEX_POINT ( 'NONE', #32348 ) ;
#7807=CARTESIAN_POINT ( 'NONE',  ( -11.79942310750000090, 1380.362273894700138, 215.1811282860990104 ) ) ;
#7814=CARTESIAN_POINT ( 'NONE',  ( -12.49220149360000143, 1391.410447351959874, 209.7524444900410003 ) ) ;
#7834=CARTESIAN_POINT ( 'NONE',  ( -16.59345386669420108, 1383.857040005859972, 219.6283172069809666 ) ) ;
#7850=CARTESIAN_POINT ( 'NONE',  ( -5.485381178602870555, 1391.646552095490051, 203.3186572502850140 ) ) ;
#7860=CARTESIAN_POINT ( 'NONE',  ( -80.90147208277250002, 1385.161082712429788, 284.2695106278820276 ) ) ;
#7862=CARTESIAN_POINT ( 'NONE',  ( -11.46257124287919993, 1391.913060387289988, 211.1273318420540193 ) ) ;
#7882=VERTEX_POINT ( 'NONE', #102829 ) ;
#7885=CARTESIAN_POINT ( 'NONE',  ( -68.65513241966479541, 1379.747663328290173, 280.2694831111389817 ) ) ;
#7887=CARTESIAN_POINT ( 'NONE',  ( -10.87959984532081315, 1378.671789283537464, 214.9412694382895950 ) ) ;
#7895=EDGE_CURVE ( 'NONE', #13762, #35724, #67873, .T. ) ;
#7898=CARTESIAN_POINT ( 'NONE',  ( -12.33979512284740032, 1378.416654683770048, 209.3708442725699967 ) ) ;
#7907=VERTEX_POINT ( 'NONE', #86600 ) ;
#7909=AXIS2_PLACEMENT_3D ( 'NONE', #48143, #74457, #48700 ) ;
#7912=CARTESIAN_POINT ( 'NONE',  ( -14.26759209886279933, 1380.297660956990057, 210.2716803301690334 ) ) ;
#7922=CARTESIAN_POINT ( 'NONE',  ( -10.33438234840000014, 1391.913060387289988, 213.9065263758590163 ) ) ;
#7923=CARTESIAN_POINT ( 'NONE',  ( -95.92809462355350547, 1384.860634349370230, 295.2544286719970046 ) ) ;
#7941=CARTESIAN_POINT ( 'NONE',  ( -56.72784561730000519, 1379.717687562220135, 254.3030452203590244 ) ) ;
#7946=ADVANCED_FACE ( 'NONE', ( #103954 ), #88770, .F. ) ;
#7958=CARTESIAN_POINT ( 'NONE',  ( -8.848550363540001129, 1384.918645891350025, 199.9247479929690030 ) ) ;
#7992=CARTESIAN_POINT ( 'NONE',  ( -11.92422183665363633, 1391.277242661766650, 212.8274714238102945 ) ) ;
#7994=CARTESIAN_POINT ( 'NONE',  ( -59.28208669626069849, 1384.698609697830079, 279.7264640965560147 ) ) ;
#7998=B_SPLINE_SURFACE_WITH_KNOTS ( 'NONE', 5, 5, ( 
 ( #10244, #44420, #93140, #70204, #16408, #84734 ),
 ( #8031, #33780, #76351, #102084, #93673, #59559 ),
 ( #89159, #72382, #97565, #53945, #11368, #2983 ),
 ( #106511, #37104, #10811, #97025, #104310, #71303 ),
 ( #28709, #29800, #11907, #20837, #27601, #38743 ),
 ( #37656, #46632, #80766, #54492, #80214, #105978 ) ),
 .UNSPECIFIED., .F., .F., .F.,
 ( 6, 6 ),
 ( 6, 6 ),
 ( 29.60743822950000137, 29.67279265790000053 ),
 ( 0.000000000000000000, 2.000000000000000000 ),
 .UNSPECIFIED. ) ;
#8003=CARTESIAN_POINT ( 'NONE',  ( -11.09965908892124986, 1378.958238937004126, 203.7193492967838324 ) ) ;
#8006=B_SPLINE_SURFACE_WITH_KNOTS ( 'NONE', 5, 5, ( 
 ( #30003, #107272, #23256, #40622, #57995, #64194 ),
 ( #91582, #23803, #5926, #38951, #92128, #64757 ),
 ( #48495, #14856, #80975, #13741, #73130, #46846 ),
 ( #4279, #82635, #100524, #38409, #98316, #40072 ),
 ( #74251, #83182, #6472, #47378, #108383, #31664 ),
 ( #89916, #56886, #98868, #47925, #21595, #55800 ) ),
 .UNSPECIFIED., .F., .F., .F.,
 ( 6, 6 ),
 ( 6, 6 ),
 ( 0.000000000000000000, 8.626417477929999578 ),
 ( 0.000000000000000000, 1.000000000000000000 ),
 .UNSPECIFIED. ) ;
#8010=CARTESIAN_POINT ( 'NONE',  ( -7.547972033258790958, 1385.319132597686121, 219.0723451529433987 ) ) ;
#8012=CARTESIAN_POINT ( 'NONE',  ( -12.11165857595690021, 1378.231759176429932, 211.4183186711239841 ) ) ;
#8024=CARTESIAN_POINT ( 'NONE',  ( -25.86321635541839825, 1379.618046691589825, 215.5872060442630129 ) ) ;
#8031=CARTESIAN_POINT ( 'NONE',  ( -109.9850237230000118, 1384.918752160720032, 311.4561207072590037 ) ) ;
#8032=CARTESIAN_POINT ( 'NONE',  ( -8.045796819630000485, 1385.423934774039935, 218.7531554344589892 ) ) ;
#8047=ORIENTED_EDGE ( 'NONE', *, *, #44567, .T. ) ;
#8048=ORIENTED_EDGE ( 'NONE', *, *, #5552, .T. ) ;
#8056=CARTESIAN_POINT ( 'NONE',  ( -7.543040680839999901, 1375.366160259910203, 209.1218465795010104 ) ) ;
#8067=EDGE_LOOP ( 'NONE', ( #90257, #48479, #13275, #15713, #25224 ) ) ;
#8070=DIRECTION ( 'NONE',  ( 0.03215278745245312569, -0.09160167974437756488, 0.9952765095826616726 ) ) ;
#8083=CARTESIAN_POINT ( 'NONE',  ( -73.03571372650000626, 1386.716914434789942, 272.3853015438590432 ) ) ;
#8085=CARTESIAN_POINT ( 'NONE',  ( -59.96058067096299737, 1385.066329289970099, 280.8915114855749948 ) ) ;
#8093=CARTESIAN_POINT ( 'NONE',  ( -8.580669785819999618, 1384.878224714429962, 218.6695462856689858 ) ) ;
#8103=DIRECTION ( 'NONE',  ( 0.5877852522921419576, -1.082133391535728970E-16, -0.8090169943751880366 ) ) ;
#8109=CARTESIAN_POINT ( 'NONE',  ( -109.3562791650000037, 1385.704763654729959, 297.1818586587590403 ) ) ;
#8141=CARTESIAN_POINT ( 'NONE',  ( -12.29651836606130111, 1378.320268164070058, 209.9934040429740207 ) ) ;
#8159=CARTESIAN_POINT ( 'NONE',  ( -8.395462808959999634, 1384.396046010230066, 199.8129347473389998 ) ) ;
#8182=CARTESIAN_POINT ( 'NONE',  ( -28.05711651015590036, 1384.551594447279967, 204.6011676599970031 ) ) ;
#8190=CARTESIAN_POINT ( 'NONE',  ( -64.48963914116505691, 1379.738450935989476, 274.0683424708428788 ) ) ;
#8194=CARTESIAN_POINT ( 'NONE',  ( -68.53407989799998745, 1379.748277114789971, 279.6522222015589705 ) ) ;
#8199=CARTESIAN_POINT ( 'NONE',  ( -7.965865502150356825, 1384.923562076983444, 199.4891873544885925 ) ) ;
#8237=EDGE_LOOP ( 'NONE', ( #98778, #49873, #65399 ) ) ;
#8247=CARTESIAN_POINT ( 'NONE',  ( -60.79172661048330184, 1383.795642611730045, 281.9543892178000419 ) ) ;
#8256=CARTESIAN_POINT ( 'NONE',  ( -44.05982002580000056, 1379.037918066350130, 230.4561377212590116 ) ) ;
#8268=CARTESIAN_POINT ( 'NONE',  ( -108.0221525909999940, 1382.696190293120026, 297.7913543730589936 ) ) ;
#8292=CARTESIAN_POINT ( 'NONE',  ( -106.9262462220000032, 1389.757047639990105, 308.9264214093590226 ) ) ;
#8341=CARTESIAN_POINT ( 'NONE',  ( -3.078458294640000315, 1387.009338736269910, 218.3238323482389944 ) ) ;
#8350=CARTESIAN_POINT ( 'NONE',  ( -11.90934194029999915, 1377.744960516140054, 212.2952750262290067 ) ) ;
#8357=CARTESIAN_POINT ( 'NONE',  ( -12.24194870120000012, 1391.816349958050068, 206.8907653080489979 ) ) ;
#8379=CARTESIAN_POINT ( 'NONE',  ( -15.99001483674529922, 1383.857625886600090, 219.4777900789640057 ) ) ;
#8402=CARTESIAN_POINT ( 'NONE',  ( -12.10628020709999930, 1391.855112016120074, 208.7312492313569976 ) ) ;
#8403=CARTESIAN_POINT ( 'NONE',  ( -85.40914635034850733, 1385.177617968390223, 289.1223791820979727 ) ) ;
#8404=CARTESIAN_POINT ( 'NONE',  ( -11.52275967872940043, 1391.913060387289988, 210.8564297640039911 ) ) ;
#8442=FILL_AREA_STYLE_COLOUR ( '', #96168 ) ;
#8443=CARTESIAN_POINT ( 'NONE',  ( -12.70021235298639972, 1379.087509944640033, 208.7980280935229871 ) ) ;
#8466=CARTESIAN_POINT ( 'NONE',  ( -101.4814120043199921, 1384.878864375810053, 296.5146955053820079 ) ) ;
#8483=CARTESIAN_POINT ( 'NONE',  ( -62.03809624990000060, 1379.749343316239901, 266.3689138319589915 ) ) ;
#8507=FACE_BOUND ( 'NONE', #89066, .T. ) ;
#8518=CARTESIAN_POINT ( 'NONE',  ( -10.67458942334280003, 1390.939239166159950, 215.3172498179779666 ) ) ;
#8535=CARTESIAN_POINT ( 'NONE',  ( -12.23039686304473506, 1377.875207865813309, 210.5705953414277189 ) ) ;
#8540=CARTESIAN_POINT ( 'NONE',  ( -66.03589273005509597, 1384.674347821650144, 290.1675141113110499 ) ) ;
#8546=CARTESIAN_POINT ( 'NONE',  ( -106.6639532879999877, 1379.150924026149823, 300.4020406703589856 ) ) ;
#8551=CARTESIAN_POINT ( 'NONE',  ( -8.361580061790082397, 1382.865204230077325, 199.9025052525546471 ) ) ;
#8559=CARTESIAN_POINT ( 'NONE',  ( -9.249153156179998447, 1382.907106044650163, 200.4653998181289865 ) ) ;
#8573=CARTESIAN_POINT ( 'NONE',  ( -31.33310914745869624, 1379.622867399459892, 219.3631401044190170 ) ) ;
#8629=CARTESIAN_POINT ( 'NONE',  ( -64.53706522309998661, 1385.084217465399888, 254.0329369609589776 ) ) ;
#8631=CARTESIAN_POINT ( 'NONE',  ( -61.29450154859880229, 1385.059859360860173, 283.1170003335910224 ) ) ;
#8642=CARTESIAN_POINT ( 'NONE',  ( -108.5927978296600003, 1383.291025085730098, 310.9196457646229987 ) ) ;
#8689=CARTESIAN_POINT ( 'NONE',  ( -28.76039927569999932, 1380.228231664269970, 215.0392276715589901 ) ) ;
#8701=VERTEX_POINT ( 'NONE', #100831 ) ;
#8729=CARTESIAN_POINT ( 'NONE',  ( -113.4000000000000057, 1375.342264060499929, 302.0293834673589686 ) ) ;
#8734=CARTESIAN_POINT ( 'NONE',  ( -47.74144289124880203, 1384.610046507420066, 221.9457723244100009 ) ) ;
#8746=CARTESIAN_POINT ( 'NONE',  ( -68.67770101600000032, 1379.747952267379787, 279.9599199388590023 ) ) ;
#8753=CARTESIAN_POINT ( 'NONE',  ( -25.94018854349999970, 1385.115782246259869, 224.2425052717590006 ) ) ;
#8755=CARTESIAN_POINT ( 'NONE',  ( -13.02200731483190133, 1385.301542061540204, 219.0627894650050109 ) ) ;
#8779=CARTESIAN_POINT ( 'NONE',  ( -7.544963895292410072, 1384.924630418719971, 219.0875845435980125 ) ) ;
#8800=CARTESIAN_POINT ( 'NONE',  ( -57.43579072256620321, 1383.800285040919789, 276.0605554277290139 ) ) ;
#8801=EDGE_CURVE ( 'NONE', #17951, #82950, #110035, .T. ) ;
#8802=FACE_OUTER_BOUND ( 'NONE', #12727, .T. ) ;
#8808=CARTESIAN_POINT ( 'NONE',  ( -43.68437696189999997, 1382.328028760530287, 247.2103273439589941 ) ) ;
#8813=DIRECTION ( 'NONE',  ( 0.000000000000000000, 0.000000000000000000, 1.000000000000000000 ) ) ;
#8818=CARTESIAN_POINT ( 'NONE',  ( -109.6762195290000079, 1383.310342075810013, 297.1796156746589759 ) ) ;
#8842=CARTESIAN_POINT ( 'NONE',  ( -108.6169391080000111, 1387.815304053930049, 310.5755581212589505 ) ) ;
#8871=VERTEX_POINT ( 'NONE', #66727 ) ;
#8881=CARTESIAN_POINT ( 'NONE',  ( -11.66261279208220181, 1391.913060387180167, 208.8812267457540202 ) ) ;
#8891=EDGE_CURVE ( 'NONE', #50916, #13762, #628, .T. ) ;
#8895=CARTESIAN_POINT ( 'NONE',  ( -1.311629847093230189E-15, 1388.651670832440004, 217.0323832392490147 ) ) ;
#8906=CARTESIAN_POINT ( 'NONE',  ( -12.04245058450000094, 1377.963961494360092, 211.7131635816590176 ) ) ;
#8911=CARTESIAN_POINT ( 'NONE',  ( -109.0150999517360049, 1384.924420285359929, 311.2646967347890268 ) ) ;
#8914=CARTESIAN_POINT ( 'NONE',  ( -11.02152004010000041, 1388.222241134549904, 201.9217105854090164 ) ) ;
#8920=CARTESIAN_POINT ( 'NONE',  ( -8.941769890295299561, 1384.291477174050215, 218.6298190130140142 ) ) ;
#8923=B_SPLINE_SURFACE_WITH_KNOTS ( 'NONE', 5, 5, ( 
 ( #95875, #19713, #44951, #19140, #79098, #94769 ),
 ( #88051, #69606, #37072, #3498, #87492, #96436 ),
 ( #53345, #43824, #10779, #71269, #80183, #103724 ),
 ( #45508, #28679, #28117, #62311, #103150, #36524 ),
 ( #27026, #46051, #70718, #27569, #2407, #11880 ),
 ( #61752, #37625, #26452, #11336, #60645, #18046 ) ),
 .UNSPECIFIED., .F., .F., .F.,
 ( 6, 6 ),
 ( 6, 6 ),
 ( 55.36927774709999994, 55.41785034089999584 ),
 ( 0.000000000000000000, 2.000000000000000000 ),
 .UNSPECIFIED. ) ;
#8951=CARTESIAN_POINT ( 'NONE',  ( -109.8948805359999881, 1384.905360643249878, 297.0284598854590286 ) ) ;
#8953=CARTESIAN_POINT ( 'NONE',  ( -5.932239102140000497, 1391.913060387289988, 203.1292509007990077 ) ) ;
#8954=CARTESIAN_POINT ( 'NONE',  ( -14.44996707430120075, 1380.126493376779763, 208.9404713352460021 ) ) ;
#8964=CARTESIAN_POINT ( 'NONE',  ( -11.29271012839999955, 1391.598770344190143, 204.5551124859889853 ) ) ;
#8965=CARTESIAN_POINT ( 'NONE',  ( -86.18995079829420547, 1385.180302516739857, 289.8088348423220282 ) ) ;
#8966=CARTESIAN_POINT ( 'NONE',  ( -11.61119566721579943, 1391.913060387289988, 210.3328882169209919 ) ) ;
#9004=CARTESIAN_POINT ( 'NONE',  ( -12.32239476379200127, 1378.308289425619932, 209.4637424472300040 ) ) ;
#9019=CARTESIAN_POINT ( 'NONE',  ( -14.16245236182539813, 1380.070782178959917, 210.9945578494510130 ) ) ;
#9029=CARTESIAN_POINT ( 'NONE',  ( -105.9631781526499879, 1384.892373102839883, 296.9815194618109899 ) ) ;
#9046=CARTESIAN_POINT ( 'NONE',  ( -37.70074109930000361, 1379.690292948239858, 220.7037071814589808 ) ) ;
#9066=AXIS2_PLACEMENT_3D ( 'NONE', #89631, #98025, #46558 ) ;
#9082=FACE_OUTER_BOUND ( 'NONE', #40093, .T. ) ;
#9105=CARTESIAN_POINT ( 'NONE',  ( -62.97033459889760110, 1384.684685141620093, 285.7574506432820272 ) ) ;
#9115=EDGE_CURVE ( 'NONE', #43749, #7780, #71276, .T. ) ;
#9142=CARTESIAN_POINT ( 'NONE',  ( -61.41519970972449727, 1379.731749473010041, 268.3043120641129917 ) ) ;
#9151=CARTESIAN_POINT ( 'NONE',  ( 11.33251049156513623, 1390.913060387289988, 208.6449207241230965 ) ) ;
#9159=SHAPE_REPRESENTATION_RELATIONSHIP ( 'NONE' , 'NONE' ,  #105979, #89391 ) ;
#9176=CARTESIAN_POINT ( 'NONE',  ( -48.43983358086703106, 1379.682889511459052, 236.6015797132022840 ) ) ;
#9177=CARTESIAN_POINT ( 'NONE',  ( 5.063121802906949550E-14, 1380.105522877180192, 207.5503168488490076 ) ) ;
#9205=CARTESIAN_POINT ( 'NONE',  ( 2.375285482014719999E-15, 1391.913060387289988, 209.1218459572589836 ) ) ;
#9208=CARTESIAN_POINT ( 'NONE',  ( -96.40267507759999432, 1388.053540364059927, 309.6952036672590225 ) ) ;
#9210=CARTESIAN_POINT ( 'NONE',  ( -61.96478079158669772, 1385.056723827129872, 284.1920504743239917 ) ) ;
#9221=CARTESIAN_POINT ( 'NONE',  ( -108.9104367519260137, 1382.394069908770007, 310.7972601483250514 ) ) ;
#9225=EDGE_CURVE ( 'NONE', #33248, #66491, #48837, .T. ) ;
#9235=CARTESIAN_POINT ( 'NONE',  ( -110.0482598020000040, 1385.373316571109854, 296.9711117078589950 ) ) ;
#9266=CARTESIAN_POINT ( 'NONE',  ( -109.9705007746040053, 1384.459140194019938, 311.4363103139680220 ) ) ;
#9300=CARTESIAN_POINT ( 'NONE',  ( -105.8625943240260057, 1378.913060387430050, 303.4239291982839859 ) ) ;
#9307=CARTESIAN_POINT ( 'NONE',  ( -37.20406409030000106, 1384.574232116320218, 210.1855829817990013 ) ) ;
#9308=CARTESIAN_POINT ( 'NONE',  ( -56.93619473763489935, 1384.654825375539986, 237.6350669292930036 ) ) ;
#9310=CARTESIAN_POINT ( 'NONE',  ( -14.47191459792289869, 1379.648775954749908, 208.1784578746709826 ) ) ;
#9313=ORIENTED_EDGE ( 'NONE', *, *, #24203, .F. ) ;
#9320=CARTESIAN_POINT ( 'NONE',  ( -68.46677781809999885, 1379.747208428909971, 279.4303135323589800 ) ) ;
#9329=CARTESIAN_POINT ( 'NONE',  ( -59.22773397600000322, 1384.821783028959999, 279.9294092910590166 ) ) ;
#9332=CARTESIAN_POINT ( 'NONE',  ( -15.66293008586210078, 1385.292435055019951, 219.5539821970690184 ) ) ;
#9342=CARTESIAN_POINT ( 'NONE',  ( -8.861482052969998691, 1384.950957082100103, 218.6848127019790127 ) ) ;
#9352=CARTESIAN_POINT ( 'NONE',  ( -103.9882530059674366, 1389.939798169118376, 304.1779183652306529 ) ) ;
#9373=CARTESIAN_POINT ( 'NONE',  ( -65.51159983505390016, 1383.789895811200040, 289.1595459118140070 ) ) ;
#9380=CARTESIAN_POINT ( 'NONE',  ( -79.49322724790000905, 1384.792572819600082, 282.9493281527590511 ) ) ;
#9390=CARTESIAN_POINT ( 'NONE',  ( -107.3889684650000049, 1382.148098258449863, 298.1845384890590367 ) ) ;
#9409=DIRECTION ( 'NONE',  ( 0.8775825618903714265, 0.000000000000000000, -0.4794255386042053368 ) ) ;
#9413=CARTESIAN_POINT ( 'NONE',  ( -108.8041703540000071, 1388.049276877389957, 310.6816495622589969 ) ) ;
#9470=CARTESIAN_POINT ( 'NONE',  ( -9.293841415499999314, 1383.221401683169915, 218.3140282643789760 ) ) ;
#9476=CARTESIAN_POINT ( 'NONE',  ( -12.37283350289999895, 1389.341656536749952, 203.7773294880390154 ) ) ;
#9493=CARTESIAN_POINT ( 'NONE',  ( -12.10555811194709896, 1383.861219994169915, 218.7921266527899888 ) ) ;
#9509=CARTESIAN_POINT ( 'NONE',  ( -13.79678095129150073, 1390.295210315099894, 211.7643565397299881 ) ) ;
#9512=CARTESIAN_POINT ( 'NONE',  ( -107.7718053235308275, 1380.453959893709680, 309.7418186890203060 ) ) ;
#9514=CARTESIAN_POINT ( 'NONE',  ( -12.28855864720000035, 1378.253615876029926, 210.0769071395779974 ) ) ;
#9515=CARTESIAN_POINT ( 'NONE',  ( -11.54008407269999914, 1391.635629144820086, 205.2048422470390108 ) ) ;
#9516=CARTESIAN_POINT ( 'NONE',  ( -69.45868144126460209, 1385.109595529130047, 264.7776320710389655 ) ) ;
#9552=CARTESIAN_POINT ( 'NONE',  ( -13.31507528231309934, 1379.509187062359842, 208.4414898241909953 ) ) ;
#9565=CARTESIAN_POINT ( 'NONE',  ( -14.22198381479079998, 1380.226902504789905, 210.5888445733199887 ) ) ;
#9573=CARTESIAN_POINT ( 'NONE',  ( -98.94755837794630793, 1384.870786900800113, 296.0572709506019464 ) ) ;
#9591=CARTESIAN_POINT ( 'NONE',  ( -30.40156113259999771, 1379.643953478429921, 214.3104896918690088 ) ) ;
#9634=DIRECTION ( 'NONE',  ( 0.02622235658550479270, -0.9995718917029567940, -0.01297772447215353626 ) ) ;
#9642=CARTESIAN_POINT ( 'NONE',  ( -83.32488467863339565, 1384.631840452700089, 305.8394389779119820 ) ) ;
#9643=CARTESIAN_POINT ( 'NONE',  ( -16.02315411856420013, 1384.943691493999950, 200.7859781080500170 ) ) ;
#9665=CARTESIAN_POINT ( 'NONE',  ( -8.762022473709999204, 1382.501695996660146, 200.2807315899889886 ) ) ;
#9681=CARTESIAN_POINT ( 'NONE',  ( -61.47253991419999863, 1379.746604392980089, 268.2739652322590018 ) ) ;
#9687=CARTESIAN_POINT ( 'NONE',  ( -107.2728094030000108, 1379.016579441009753, 308.4876107606589812 ) ) ;
#9716=CARTESIAN_POINT ( 'NONE',  ( -34.04422864232062551, 1379.637802395616518, 217.1019886382790389 ) ) ;
#9746=CARTESIAN_POINT ( 'NONE',  ( -89.08896662849998904, 1386.751329644390125, 292.3648858342590415 ) ) ;
#9758=CARTESIAN_POINT ( 'NONE',  ( -109.3809973283789958, 1382.669152972790243, 311.0761981651330643 ) ) ;
#9792=EDGE_CURVE ( 'NONE', #19741, #34413, #3218, .T. ) ;
#9812=CARTESIAN_POINT ( 'NONE',  ( -105.6263533753079997, 1379.015674155129773, 306.1169297802109668 ) ) ;
#9822=( BOUNDED_CURVE ( )  B_SPLINE_CURVE ( 3, ( #43569, #75527, #101787, #103448 ),
 .UNSPECIFIED., .F., .F. ) 
 B_SPLINE_CURVE_WITH_KNOTS ( ( 4, 4 ),
 ( 4.613321846721008868, 4.741587033746983870 ),
 .UNSPECIFIED. ) 
 CURVE ( )  GEOMETRIC_REPRESENTATION_ITEM ( )  RATIONAL_B_SPLINE_CURVE ( ( 1.000000000000000000, 0.9986294733265421719, 0.9986294733265421719, 1.000000000000000000 ) ) 
 REPRESENTATION_ITEM ( '' )  );
#9846=CARTESIAN_POINT ( 'NONE',  ( -69.36674279230000195, 1374.746858117589909, 280.1513224085589968 ) ) ;
#9847=CARTESIAN_POINT ( 'NONE',  ( -105.8174845808659938, 1378.913060387339783, 303.6992540374549776 ) ) ;
#9852=CARTESIAN_POINT ( 'NONE',  ( -89.15245910350000713, 1385.190331364289932, 292.2648985219589690 ) ) ;
#9853=CARTESIAN_POINT ( 'NONE',  ( -50.36207809872559693, 1384.621281085180044, 225.8468432978239662 ) ) ;
#9863=CARTESIAN_POINT ( 'NONE',  ( -68.59837639049999325, 1379.747520377230103, 279.7248781293590127 ) ) ;
#9866=CIRCLE ( 'NONE', #70828, 7.999657266239995401 ) ;
#9869=ORIENTED_EDGE ( 'NONE', *, *, #94615, .F. ) ;
#9872=CARTESIAN_POINT ( 'NONE',  ( -19.17332639309999820, 1385.003280231690042, 220.5251654938589922 ) ) ;
#9874=CARTESIAN_POINT ( 'NONE',  ( -18.64720036659560165, 1385.281482332319911, 220.4066171626870130 ) ) ;
#9885=CARTESIAN_POINT ( 'NONE',  ( -8.866353092783899825, 1385.153809896229859, 218.6758262535360018 ) ) ;
#9894=UNCERTAINTY_MEASURE_WITH_UNIT (LENGTH_MEASURE( 1.000000000000000082E-05 ), #22054, 'distance_accuracy_value', 'NONE');
#9915=DIRECTION ( 'NONE',  ( 0.01668530547205106240, -0.7071067811868640973, -0.7069098956591685079 ) ) ;
#9917=CARTESIAN_POINT ( 'NONE',  ( -96.51683378141680691, 1383.766218890880054, 310.1534002763809781 ) ) ;
#9925=CARTESIAN_POINT ( 'NONE',  ( -65.46515651720000051, 1380.024545039450004, 282.7246703598589761 ) ) ;
#9937=CARTESIAN_POINT ( 'NONE',  ( -109.6436185679999937, 1384.428537382530067, 297.1050702840590247 ) ) ;
#9979=EDGE_CURVE ( 'NONE', #93351, #6492, #101916, .T. ) ;
#10012=CARTESIAN_POINT ( 'NONE',  ( -8.711610717349350286E-16, 1387.020289398270052, 218.3670623203690013 ) ) ;
#10021=CARTESIAN_POINT ( 'NONE',  ( -9.959589622450000235, 1382.751681251990021, 218.0704319110489848 ) ) ;
#10047=CARTESIAN_POINT ( 'NONE',  ( -13.22271691091419932, 1383.860216996029976, 218.9433012605030058 ) ) ;
#10055=CARTESIAN_POINT ( 'NONE',  ( -8.325264604675567170, 1386.880005921131669, 199.8668364905755368 ) ) ;
#10062=CARTESIAN_POINT ( 'NONE',  ( -14.37394065297739942, 1380.292840319920060, 209.5077344925099965 ) ) ;
#10069=CARTESIAN_POINT ( 'NONE',  ( -11.65327852769999950, 1391.913060471080144, 207.1342100345190147 ) ) ;
#10070=CARTESIAN_POINT ( 'NONE',  ( -71.11683232987380165, 1385.117871785510260, 268.1819042305770040 ) ) ;
#10072=CARTESIAN_POINT ( 'NONE',  ( -65.00001850430001582, 1379.749314314899948, 272.6104031607590059 ) ) ;
#10078=DIRECTION ( 'NONE',  ( -0.02701649886402238826, 0.9995674067478985680, -0.01162360341768371545 ) ) ;
#10103=DIRECTION ( 'NONE',  ( 1.836970198721029688E-16, 1.000000000000000000, -7.703719777548939991E-34 ) ) ;
#10134=CARTESIAN_POINT ( 'NONE',  ( -96.48208606500890028, 1384.862543659289940, 295.4255336162560184 ) ) ;
#10151=CARTESIAN_POINT ( 'NONE',  ( -32.76203973510000367, 1379.634334059360071, 215.8302746649189885 ) ) ;
#10173=LINE ( 'NONE', #691, #62937 ) ;
#10183=DIRECTION ( 'NONE',  ( -4.481801771516530428E-20, -1.000000000000000000, -2.868959329816139585E-18 ) ) ;
#10186=CARTESIAN_POINT ( 'NONE',  ( -12.32335714446040065, 1378.400099640540020, 208.6449807495420146 ) ) ;
#10193=CARTESIAN_POINT ( 'NONE',  ( -7.595232024581050290, 1384.066046907910049, 219.0217700005140102 ) ) ;
#10206=CARTESIAN_POINT ( 'NONE',  ( -70.52881574989599756, 1384.661057111879927, 295.6545454185069843 ) ) ;
#10207=CARTESIAN_POINT ( 'NONE',  ( -16.57194402519859722, 1384.944668023739723, 200.8899537780140179 ) ) ;
#10223=CARTESIAN_POINT ( 'NONE',  ( -10.39382043080000173, 1382.190468632969896, 201.2536150431689919 ) ) ;
#10228=AXIS2_PLACEMENT_3D ( 'NONE', #75333, #50664, #76978 ) ;
#10237=CARTESIAN_POINT ( 'NONE',  ( -64.35649047367049036, 1379.742209816759896, 273.6236211245889649 ) ) ;
#10244=CARTESIAN_POINT ( 'NONE',  ( -109.9849727219999949, 1384.916905217840167, 311.4561123622590344 ) ) ;
#10267=CARTESIAN_POINT ( 'NONE',  ( -22.74071171259225821, 1379.610629053026287, 210.0440409253812675 ) ) ;
#10286=AXIS2_PLACEMENT_3D ( 'NONE', #107278, #80981, #64763 ) ;
#10293=EDGE_CURVE ( 'NONE', #6840, #110498, #24412, .T. ) ;
#10296=CARTESIAN_POINT ( 'NONE',  ( -96.24445620069998597, 1386.506167415560185, 310.5622141132590173 ) ) ;
#10310=CARTESIAN_POINT ( 'NONE',  ( -107.9019887798300061, 1382.633163608059931, 310.5403456482189881 ) ) ;
#10327=DIRECTION ( 'NONE',  ( 1.836970198721029688E-16, 1.000000000000000000, -2.953460612019999929E-19 ) ) ;
#10337=CARTESIAN_POINT ( 'NONE',  ( -22.01162841000270021, 1384.855953449889967, 221.8868375699159969 ) ) ;
#10357=CARTESIAN_POINT ( 'NONE',  ( -109.9782865922809947, 1384.547503231000064, 311.4425668244260237 ) ) ;
#10396=CARTESIAN_POINT ( 'NONE',  ( -77.77200720220001529, 1379.656469662929794, 291.9281914769590003 ) ) ;
#10398=CARTESIAN_POINT ( 'NONE',  ( -105.8561346205080014, 1378.913060387450059, 303.4563273789140112 ) ) ;
#10403=CARTESIAN_POINT ( 'NONE',  ( -98.86683315710000386, 1385.218296336320009, 296.2584199137589849 ) ) ;
#10404=CARTESIAN_POINT ( 'NONE',  ( -59.39287138243709308, 1384.669285364579991, 242.7124994448570021 ) ) ;
#10412=CARTESIAN_POINT ( 'NONE',  ( -26.04564454490000003, 1383.846902489159902, 224.1106665064590118 ) ) ;
#10417=CARTESIAN_POINT ( 'NONE',  ( -66.38361129989999654, 1379.743368401719863, 275.3027083311590104 ) ) ;
#10426=CARTESIAN_POINT ( 'NONE',  ( -62.06510066419999561, 1384.932470540059967, 284.7693340512589657 ) ) ;
#10429=CARTESIAN_POINT ( 'NONE',  ( -19.06873360288100017, 1385.279875393399834, 220.5578134822330014 ) ) ;
#10442=ORIENTED_EDGE ( 'NONE', *, *, #110315, .T. ) ;
#10476=CARTESIAN_POINT ( 'NONE',  ( -81.44223561470580819, 1383.775960391189983, 304.5617243241840129 ) ) ;
#10485=CARTESIAN_POINT ( 'NONE',  ( -63.74074695120000911, 1380.989849089459995, 283.7619814212590086 ) ) ;
#10495=CARTESIAN_POINT ( 'NONE',  ( -109.7136633519999975, 1383.888121385389923, 297.1243086093589909 ) ) ;
#10562=ORIENTED_EDGE ( 'NONE', *, *, #96759, .F. ) ;
#10571=CARTESIAN_POINT ( 'NONE',  ( -48.13349220509999782, 1389.567894374660000, 227.8887496536589765 ) ) ;
#10573=CARTESIAN_POINT ( 'NONE',  ( -11.56174262037960077, 1388.455307283889624, 216.7304434050078044 ) ) ;
#10595=CARTESIAN_POINT ( 'NONE',  ( -12.31888605675350057, 1378.301144730269925, 209.5654755735049832 ) ) ;
#10612=CARTESIAN_POINT ( 'NONE',  ( -34.42280635277390388, 1383.836280062859942, 233.0998386971220100 ) ) ;
#10622=CARTESIAN_POINT ( 'NONE',  ( -9.639940909925840019E-16, 1380.874075505639894, 216.4545132979889956 ) ) ;
#10628=CARTESIAN_POINT ( 'NONE',  ( -14.35128743697329945, 1380.312783049660084, 209.6729884863009943 ) ) ;
#10635=CARTESIAN_POINT ( 'NONE',  ( -11.32737004039999995, 1391.820807817859986, 205.2942467584589679 ) ) ;
#10636=CARTESIAN_POINT ( 'NONE',  ( -100.3556198889290130, 1385.221765029460130, 296.3440159043000222 ) ) ;
#10644=DIRECTION ( 'NONE',  ( 0.07284846526757217389, 0.01356562619974717963, 0.9972507582819719607 ) ) ;
#10646=ORIENTED_EDGE ( 'NONE', *, *, #81643, .T. ) ;
#10665=CARTESIAN_POINT ( 'NONE',  ( -68.75491282716379260, 1379.747882944909861, 280.3318558483960601 ) ) ;
#10701=ORIENTED_EDGE ( 'NONE', *, *, #98017, .T. ) ;
#10717=CARTESIAN_POINT ( 'NONE',  ( -44.38987040500000347, 1379.668466784379916, 229.4021183653589731 ) ) ;
#10721=CARTESIAN_POINT ( 'NONE',  ( -31.51240728497394628, 1379.723496874464445, 219.1466601198638386 ) ) ;
#10727=CARTESIAN_POINT ( 'NONE',  ( -113.3174119514818301, 1378.913060387289988, 300.7228204909002329 ) ) ;
#10730=CARTESIAN_POINT ( 'NONE',  ( -8.727481514770000004, 1384.944701276459909, 199.8872933186289913 ) ) ;
#10762=CARTESIAN_POINT ( 'NONE',  ( -7.544607327050279366, 1384.638857144239864, 219.0792297806210058 ) ) ;
#10772=CARTESIAN_POINT ( 'NONE',  ( -73.29286402757139740, 1384.653836098580086, 298.4869674903130203 ) ) ;
#10773=CARTESIAN_POINT ( 'NONE',  ( -34.05251678726769882, 1384.976729253169879, 208.0367919944089863 ) ) ;
#10779=CARTESIAN_POINT ( 'NONE',  ( -8.371286044520001468, 1384.927627653609989, 199.7749606464490171 ) ) ;
#10792=CARTESIAN_POINT ( 'NONE',  ( -13.48698396448789971, 1379.694001781489987, 211.4569706220899832 ) ) ;
#10804=CARTESIAN_POINT ( 'NONE',  ( -61.35634870417439402, 1379.727770043109786, 268.3354436782490211 ) ) ;
#10810=CARTESIAN_POINT ( 'NONE',  ( -105.6182501849999937, 1378.913057670360104, 304.5676750416590153 ) ) ;
#10811=CARTESIAN_POINT ( 'NONE',  ( -109.6578465720000111, 1384.929364751169942, 311.3230191942589613 ) ) ;
#10817=CARTESIAN_POINT ( 'NONE',  ( -105.9286161621180042, 1378.913060388629901, 305.0991713824849967 ) ) ;
#10829=ORIENTED_EDGE ( 'NONE', *, *, #32300, .T. ) ;
#10838=CARTESIAN_POINT ( 'NONE',  ( -58.27299464524384121, 1379.718854485406837, 257.4714984816578180 ) ) ;
#10850=CARTESIAN_POINT ( 'NONE',  ( -57.37605527416430817, 1379.717849395646226, 260.5878764870727196 ) ) ;
#10868=CARTESIAN_POINT ( 'NONE',  ( -93.52692659189999347, 1389.453883371680149, 297.6663029733589951 ) ) ;
#10873=EDGE_CURVE ( 'NONE', #66359, #29914, #22974, .T. ) ;
#10881=CARTESIAN_POINT ( 'NONE',  ( -104.8397582023220025, 1379.985347132740117, 306.4823361143110105 ) ) ;
#10906=CARTESIAN_POINT ( 'NONE',  ( -20.11165657711670107, 1384.861962272929986, 220.9937321937230195 ) ) ;
#10928=CARTESIAN_POINT ( 'NONE',  ( -109.5441724309999927, 1377.044192470269991, 306.8927967050020129 ) ) ;
#10953=ORIENTED_EDGE ( 'NONE', *, *, #28360, .T. ) ;
#10962=CARTESIAN_POINT ( 'NONE',  ( -70.57508978779999609, 1375.676061790260064, 279.4267215269589428 ) ) ;
#10966=CARTESIAN_POINT ( 'NONE',  ( -103.7376339979999926, 1385.115701970539931, 296.9235426477590067 ) ) ;
#10978=CARTESIAN_POINT ( 'NONE',  ( -67.40081635460001053, 1379.748791505480085, 277.3949072269590488 ) ) ;
#10986=CARTESIAN_POINT ( 'NONE',  ( -67.04611378480001349, 1384.669946114650202, 292.1828053715589704 ) ) ;
#10988=CARTESIAN_POINT ( 'NONE',  ( -8.888758267720000106, 1385.314821192629779, 218.6605176881890031 ) ) ;
#10990=CARTESIAN_POINT ( 'NONE',  ( -113.4000000000000057, 1378.913060387289988, 304.2218459572590064 ) ) ;
#11037=CARTESIAN_POINT ( 'NONE',  ( -78.11014189374911609, 1383.778372959410262, 302.3262168834259569 ) ) ;
#11044=CARTESIAN_POINT ( 'NONE',  ( -89.13551699850000887, 1383.359784101189916, 292.2933295549590298 ) ) ;
#11049=CARTESIAN_POINT ( 'NONE',  ( -110.0628159060000115, 1384.912455446979948, 296.9513137223589752 ) ) ;
#11081=ADVANCED_FACE ( 'NONE', ( #15691 ), #109781, .T. ) ;
#11092=CARTESIAN_POINT ( 'NONE',  ( -11.66658784013729999, 1391.913060387289988, 209.7120188154370339 ) ) ;
#11126=CARTESIAN_POINT ( 'NONE',  ( -11.32491995773190041, 1391.913060387279984, 206.9750921995710087 ) ) ;
#11136=CARTESIAN_POINT ( 'NONE',  ( -19.72061575229999875, 1388.557148333510213, 219.1405698173590224 ) ) ;
#11144=CARTESIAN_POINT ( 'NONE',  ( -8.129796171130001525, 1383.479577432089854, 218.6364202077689924 ) ) ;
#11163=CARTESIAN_POINT ( 'NONE',  ( -109.1565231619999992, 1385.185641183290045, 297.1420090250589965 ) ) ;
#11166=CARTESIAN_POINT ( 'NONE',  ( -105.5686647185313376, 1391.210135304358346, 305.6570493640687118 ) ) ;
#11176=CARTESIAN_POINT ( 'NONE',  ( -22.08626087506250002, 1383.851343771249958, 221.7312892301039824 ) ) ;
#11185=CARTESIAN_POINT ( 'NONE',  ( -8.201645939166466448, 1386.531733650833758, 199.7449378919872913 ) ) ;
#11190=CARTESIAN_POINT ( 'NONE',  ( -14.39625711568469946, 1380.260135093950112, 209.3432647037969900 ) ) ;
#11191=CARTESIAN_POINT ( 'NONE',  ( -10.03264644813917705, 1391.913060248523607, 214.9446882421459861 ) ) ;
#11198=CARTESIAN_POINT ( 'NONE',  ( -102.6473507896519948, 1385.227429346269901, 296.6858408320929925 ) ) ;
#11205=EDGE_CURVE ( 'NONE', #61557, #98535, #69125, .T. ) ;
#11258=CARTESIAN_POINT ( 'NONE',  ( -109.1645132478509908, 1384.901512804259937, 297.1326343494729940 ) ) ;
#11274=CARTESIAN_POINT ( 'NONE',  ( -30.32475187390000215, 1379.724315040820102, 214.4187306602189835 ) ) ;
#11284=CARTESIAN_POINT ( 'NONE',  ( -64.65699941863819333, 1385.044778570139897, 288.2599696774469749 ) ) ;
#11315=CARTESIAN_POINT ( 'NONE',  ( -7.565574591425869855, 1384.312222434259866, 219.0525576736690141 ) ) ;
#11328=CARTESIAN_POINT ( 'NONE',  ( -85.63289024257620952, 1384.627373604930199, 306.9865616185009571 ) ) ;
#11330=CARTESIAN_POINT ( 'NONE',  ( -33.66923337122079829, 1384.975952570079926, 207.7792561057779892 ) ) ;
#11336=CARTESIAN_POINT ( 'NONE',  ( -8.603957690599999708, 1384.941249256889932, 199.8686546726490008 ) ) ;
#11341=EDGE_CURVE ( 'NONE', #40014, #40412, #35120, .T. ) ;
#11343=CARTESIAN_POINT ( 'NONE',  ( -106.5949931321939914, 1391.913060387289988, 305.5646014930300112 ) ) ;
#11347=CARTESIAN_POINT ( 'NONE',  ( -12.14249633790000082, 1377.794244260820051, 206.8888716493889888 ) ) ;
#11361=CARTESIAN_POINT ( 'NONE',  ( -65.44977854169999887, 1379.747342584589887, 275.4353169223589930 ) ) ;
#11367=CARTESIAN_POINT ( 'NONE',  ( -105.4520934690000047, 1378.947384221549783, 304.5880789179589669 ) ) ;
#11368=CARTESIAN_POINT ( 'NONE',  ( -109.3076610239999980, 1384.932499147180124, 311.2646262372589945 ) ) ;
#11393=CARTESIAN_POINT ( 'NONE',  ( -66.28715543682936584, 1379.742552331314528, 274.9634317763816398 ) ) ;
#11401=B_SPLINE_CURVE_WITH_KNOTS ( 'NONE', 3,
 ( #1491, #18810, #61414, #93863, #69255, #42938 ),
 .UNSPECIFIED., .F., .F.,
 ( 4, 2, 4 ),
 ( 0.000000000000000000, 0.5000000000000000000, 1.000000000000000000 ),
 .UNSPECIFIED. ) ;
#11406=CARTESIAN_POINT ( 'NONE',  ( -51.74412866941842282, 1379.698572072603383, 249.1812003707125882 ) ) ;
#11423=CARTESIAN_POINT ( 'NONE',  ( -103.6582916800000049, 1388.280209741639965, 298.0463838127590748 ) ) ;
#11424=ORIENTED_EDGE ( 'NONE', *, *, #43339, .T. ) ;
#11434=CARTESIAN_POINT ( 'NONE',  ( -106.3487258514710021, 1380.529443125889884, 308.5284918366859870 ) ) ;
#11458=CARTESIAN_POINT ( 'NONE',  ( -28.12733322275310144, 1384.835236073490023, 226.2207532044819800 ) ) ;
#11477=CARTESIAN_POINT ( 'NONE',  ( -109.9873428579799963, 1384.764085902139868, 311.4531231889159812 ) ) ;
#11482=CARTESIAN_POINT ( 'NONE',  ( -56.13014929047670165, 1379.450323875860022, 260.0068040503380189 ) ) ;
#11493=CARTESIAN_POINT ( 'NONE',  ( -7.769784056169999786, 1383.283767220619893, 218.8591793915190067 ) ) ;
#11515=CARTESIAN_POINT ( 'NONE',  ( -63.58938923220000561, 1379.821258372549892, 269.7443356278590159 ) ) ;
#11517=CARTESIAN_POINT ( 'NONE',  ( -107.2050354704289958, 1378.913060387309770, 300.9024058946000082 ) ) ;
#11528=FACE_OUTER_BOUND ( 'NONE', #40312, .T. ) ;
#11532=CARTESIAN_POINT ( 'NONE',  ( -65.92707478070001059, 1379.741696281819941, 274.2307012748590296 ) ) ;
#11538=ORIENTED_EDGE ( 'NONE', *, *, #36740, .F. ) ;
#11543=CARTESIAN_POINT ( 'NONE',  ( -22.15429900546649833, 1385.267682785860188, 221.9372924518760044 ) ) ;
#11586=CARTESIAN_POINT ( 'NONE',  ( -82.66607780726680232, 1383.775112911549968, 305.2794127350090321 ) ) ;
#11587=CARTESIAN_POINT ( 'NONE',  ( -108.7284267277110104, 1383.837174741619947, 311.1014926787349850 ) ) ;
#11592=CARTESIAN_POINT ( 'NONE',  ( -92.36490218759999493, 1379.347538457270048, 300.9928459216590113 ) ) ;
#11603=CARTESIAN_POINT ( 'NONE',  ( -109.8051728760000003, 1384.892702632449982, 297.0523066442589766 ) ) ;
#11630=ORIENTED_EDGE ( 'NONE', *, *, #68499, .T. ) ;
#11670=CARTESIAN_POINT ( 'NONE',  ( -28.25951253750000092, 1389.755799385790169, 221.3495615508589935 ) ) ;
#11671=CARTESIAN_POINT ( 'NONE',  ( -14.28029386204369899, 1390.367275669339961, 209.8449220790990069 ) ) ;
#11708=CARTESIAN_POINT ( 'NONE',  ( -30.09804076777400184, 1383.841955765280090, 227.9062932389740297 ) ) ;
#11718=CARTESIAN_POINT ( 'NONE',  ( -9.039250672204644843, 1388.268641467896032, 200.6155552593253617 ) ) ;
#11726=CARTESIAN_POINT ( 'NONE',  ( -9.612506535307179689, 1386.943031418069950, 218.1121965012910096 ) ) ;
#11735=CARTESIAN_POINT ( 'NONE',  ( -97.02964055224740036, 1385.213118710479876, 295.5936257578139816 ) ) ;
#11739=ORIENTED_EDGE ( 'NONE', *, *, #78509, .F. ) ;
#11751=CARTESIAN_POINT ( 'NONE',  ( 8.013264357029996177, 1375.413060387289988, 209.1218459572589836 ) ) ;
#11752=CARTESIAN_POINT ( 'NONE',  ( -8.295657568419999350, 1385.027123149139925, 218.7016715734189916 ) ) ;
#11775=CARTESIAN_POINT ( 'NONE',  ( -25.91644647850000283, 1384.822840952090019, 203.4460669693289958 ) ) ;
#11786=CIRCLE ( 'NONE', #85066, 0.5000000000000004441 ) ;
#11813=CARTESIAN_POINT ( 'NONE',  ( -68.19307365517850883, 1379.747659725522226, 279.6816280296294508 ) ) ;
#11819=CARTESIAN_POINT ( 'NONE',  ( -71.28004258136559201, 1385.019770350649878, 296.4666894103959862 ) ) ;
#11837=EDGE_CURVE ( 'NONE', #23316, #93351, #82626, .T. ) ;
#11854=CARTESIAN_POINT ( 'NONE',  ( -7.769784805680000517, 1383.283764732429972, 218.8591787099389876 ) ) ;
#11871=CARTESIAN_POINT ( 'NONE',  ( -35.93338201885099892, 1384.980665049489971, 209.4036774743509852 ) ) ;
#11877=AXIS2_PLACEMENT_3D ( 'NONE', #47542, #82229, #12819 ) ;
#11880=CARTESIAN_POINT ( 'NONE',  ( -9.094348614660001218, 1384.950164682069953, 199.9428816977090264 ) ) ;
#11886=CARTESIAN_POINT ( 'NONE',  ( -106.9109750466100053, 1391.913060387289988, 306.4819379310129648 ) ) ;
#11890=CARTESIAN_POINT ( 'NONE',  ( -13.57816499950000022, 1379.569537802170089, 207.8818212896190118 ) ) ;
#11901=CARTESIAN_POINT ( 'NONE',  ( -67.96720087744429861, 1379.746016284620055, 279.4351274535100060 ) ) ;
#11906=CARTESIAN_POINT ( 'NONE',  ( -105.8639003480000014, 1378.913060387289988, 305.0513551771590528 ) ) ;
#11907=CARTESIAN_POINT ( 'NONE',  ( -109.6580479539999970, 1384.932677638599898, 311.3230131862590042 ) ) ;
#11917=ORIENTED_EDGE ( 'NONE', *, *, #50275, .T. ) ;
#11925=ADVANCED_FACE ( 'NONE', ( #23706 ), #22070, .F. ) ;
#11927=CARTESIAN_POINT ( 'NONE',  ( -8.581480553229999586, 1384.925094855179850, 218.6696853789089801 ) ) ;
#11931=CARTESIAN_POINT ( 'NONE',  ( -63.79925921728045779, 1379.736147238250169, 269.7686537772054294 ) ) ;
#11952=CARTESIAN_POINT ( 'NONE',  ( -103.5801209296959939, 1379.883073482990085, 303.9981235976169955 ) ) ;
#11960=CARTESIAN_POINT ( 'NONE',  ( -113.4000000000000057, 1385.251674955540238, 297.2379167808589955 ) ) ;
#11969=ADVANCED_FACE ( 'NONE', ( #25346 ), #56076, .T. ) ;
#11976=CARTESIAN_POINT ( 'NONE',  ( -105.8736429085269890, 1378.613677389549821, 306.5408079283200209 ) ) ;
#11987=CARTESIAN_POINT ( 'NONE',  ( -107.2374608147510031, 1384.994991009320074, 298.2563606770149818 ) ) ;
#12001=CARTESIAN_POINT ( 'NONE',  ( -37.33982031581620475, 1384.799273965830025, 237.6968796437000151 ) ) ;
#12017=CARTESIAN_POINT ( 'NONE',  ( -12.32664273690000023, 1378.996295195989887, 209.7960013046609902 ) ) ;
#12024=CARTESIAN_POINT ( 'NONE',  ( -47.74616927649559983, 1377.617239580540172, 243.6775589761319907 ) ) ;
#12033=CARTESIAN_POINT ( 'NONE',  ( -7.777873728749999493, 1384.438531822959931, 218.8954641931690333 ) ) ;
#12041=FACE_OUTER_BOUND ( 'NONE', #109948, .T. ) ;
#12056=CARTESIAN_POINT ( 'NONE',  ( -94.91986059570000123, 1375.460834337080087, 300.7314404810590531 ) ) ;
#12066=CARTESIAN_POINT ( 'NONE',  ( -19.23736494940000341, 1383.854422637459948, 220.3626903602589948 ) ) ;
#12070=CARTESIAN_POINT ( 'NONE',  ( -66.42105914469999561, 1379.741982406930219, 275.2841866764590009 ) ) ;
#12079=CARTESIAN_POINT ( 'NONE',  ( -109.9987472809999929, 1384.581606379090090, 311.2589846932590376 ) ) ;
#12081=CARTESIAN_POINT ( 'NONE',  ( -25.36236875327359996, 1385.254273797359929, 223.9400902521850014 ) ) ;
#12108=CARTESIAN_POINT ( 'NONE',  ( -105.5826323030000111, 1391.887506638209970, 304.2218459572590064 ) ) ;
#12116=DIRECTION ( 'NONE',  ( -1.000000000000000000, 0.000000000000000000, 0.000000000000000000 ) ) ;
#12127=CARTESIAN_POINT ( 'NONE',  ( -81.60401292589429545, 1383.775847213790030, 304.6599215716950084 ) ) ;
#12128=DIRECTION ( 'NONE',  ( -1.000000000000000000, 0.000000000000000000, 0.000000000000000000 ) ) ;
#12138=CARTESIAN_POINT ( 'NONE',  ( -109.7187112120000023, 1384.936990306269763, 297.0861906625590336 ) ) ;
#12214=CARTESIAN_POINT ( 'NONE',  ( -14.06995080394465525, 1379.599519235348453, 211.7445496221188819 ) ) ;
#12238=CARTESIAN_POINT ( 'NONE',  ( -109.1685115749999966, 1385.071170989440134, 297.1353643137590552 ) ) ;
#12249=CARTESIAN_POINT ( 'NONE',  ( -24.45121130426860034, 1383.848703213860063, 223.1218506052400130 ) ) ;
#12257=CARTESIAN_POINT ( 'NONE',  ( -45.10563462580000049, 1381.548674952109877, 219.7946006703589887 ) ) ;
#12263=CARTESIAN_POINT ( 'NONE',  ( -11.37061168853300153, 1391.632271866039900, 214.0126550961279861 ) ) ;
#12264=CARTESIAN_POINT ( 'NONE',  ( -10.66875363927314169, 1391.196586595016470, 215.3138778947951550 ) ) ;
#12270=CARTESIAN_POINT ( 'NONE',  ( -87.21881660688978855, 1385.183764852800095, 290.6465622116569989 ) ) ;
#12272=CARTESIAN_POINT ( 'NONE',  ( -68.77626911307648072, 1379.747998350314901, 280.2622293725648888 ) ) ;
#12295=CARTESIAN_POINT ( 'NONE',  ( -107.5634112720000104, 1382.701802836779962, 297.7923862875589975 ) ) ;
#12346=CARTESIAN_POINT ( 'NONE',  ( -106.2561851244600035, 1391.913059884029963, 305.4819836422510093 ) ) ;
#12347=CARTESIAN_POINT ( 'NONE',  ( -67.99816612433596674, 1379.747625308294573, 279.4122903084538052 ) ) ;
#12355=CARTESIAN_POINT ( 'NONE',  ( -80.80534708309519942, 1384.991848082589968, 304.3854582852239901 ) ) ;
#12408=CARTESIAN_POINT ( 'NONE',  ( -96.47684263679849437, 1384.607351846010033, 310.3230601989450292 ) ) ;
#12409=CARTESIAN_POINT ( 'NONE',  ( -39.25154068821980502, 1384.988109809909929, 212.1860968133940162 ) ) ;
#12416=CARTESIAN_POINT ( 'NONE',  ( -109.9853374259999867, 1384.903358540060026, 311.4562094292589904 ) ) ;
#12441=CARTESIAN_POINT ( 'NONE',  ( -67.81516288620989030, 1379.745697675489964, 279.2085842206279835 ) ) ;
#12446=CARTESIAN_POINT ( 'NONE',  ( -105.0581302270000066, 1379.236400489019843, 304.0328620110590236 ) ) ;
#12461=DIRECTION ( 'NONE',  ( 1.836970198721029688E-16, 1.000000000000000000, -2.953460612019999929E-19 ) ) ;
#12477=CARTESIAN_POINT ( 'NONE',  ( -68.14071486192135296, 1379.746697161519705, 278.7208864299544189 ) ) ;
#12481=CARTESIAN_POINT ( 'NONE',  ( -61.39005965052979974, 1384.681648932039934, 247.0307441228220000 ) ) ;
#12512=CARTESIAN_POINT ( 'NONE',  ( -106.4826975579999981, 1389.246194448199958, 308.7719952443590046 ) ) ;
#12515=CIRCLE ( 'NONE', #51916, 0.5000000000000004441 ) ;
#12525=CARTESIAN_POINT ( 'NONE',  ( -105.2403994794200059, 1380.288835873570179, 307.4042895074139778 ) ) ;
#12550=CARTESIAN_POINT ( 'NONE',  ( -36.08493826582400033, 1384.804586415280028, 235.7710440410830017 ) ) ;
#12552=CARTESIAN_POINT ( 'NONE',  ( -105.9089176949999995, 1378.913060387289988, 303.0252558878589753 ) ) ;
#12575=CARTESIAN_POINT ( 'NONE',  ( -86.23580615497749591, 1378.226136009930087, 302.2523813644399979 ) ) ;
#12582=EDGE_CURVE ( 'NONE', #85936, #8701, #30738, .T. ) ;
#12585=CARTESIAN_POINT ( 'NONE',  ( -7.683071123930000468, 1383.591828314379882, 218.9382038826490202 ) ) ;
#12595=CARTESIAN_POINT ( 'NONE',  ( -1.836970198721029983E-15, 1374.913060387289988, 209.1218459572589836 ) ) ;
#12607=CARTESIAN_POINT ( 'NONE',  ( -13.18481025451849931, 1379.800827107049827, 208.6184356723600217 ) ) ;
#12611=CARTESIAN_POINT ( 'NONE',  ( -28.76039927569999932, 1380.228231664269970, 215.0392276715589901 ) ) ;
#12624=CARTESIAN_POINT ( 'NONE',  ( -5.960032396909999974, 1384.206784872530079, 218.4667819198089944 ) ) ;
#12628=VECTOR ( 'NONE', #24763, 999.9999999999998863 ) ;
#12630=CARTESIAN_POINT ( 'NONE',  ( -66.55629426049999608, 1379.749035308849898, 275.7365325667589673 ) ) ;
#12640=CARTESIAN_POINT ( 'NONE',  ( -22.89778237906369895, 1385.264640953090066, 222.3446852156519924 ) ) ;
#12641=DIRECTION ( 'NONE',  ( -1.000000000000000000, 0.000000000000000000, 0.000000000000000000 ) ) ;
#12652=ORIENTED_EDGE ( 'NONE', *, *, #67363, .F. ) ;
#12671=CARTESIAN_POINT ( 'NONE',  ( -105.5847408669999936, 1378.244047627129930, 303.6830150497589784 ) ) ;
#12682=CARTESIAN_POINT ( 'NONE',  ( -107.5775718089879973, 1383.759024782929828, 311.0686465984289839 ) ) ;
#12683=CARTESIAN_POINT ( 'NONE',  ( -109.9562721537739947, 1384.319945152750051, 311.4255092121239841 ) ) ;
#12690=ORIENTED_EDGE ( 'NONE', *, *, #9225, .T. ) ;
#12692=CARTESIAN_POINT ( 'NONE',  ( -109.8952007060000113, 1384.926598849860056, 297.0284133136589730 ) ) ;
#12727=EDGE_LOOP ( 'NONE', ( #34556, #10701, #5146, #46401 ) ) ;
#12740=CIRCLE ( 'NONE', #107443, 12.49965726619999984 ) ;
#12742=CARTESIAN_POINT ( 'NONE',  ( -17.59599179729789853, 1384.528033373270091, 201.1169542061229834 ) ) ;
#12791=CARTESIAN_POINT ( 'NONE',  ( -12.31627863005989987, 1378.354374910739807, 209.6655814783919709 ) ) ;
#12802=CARTESIAN_POINT ( 'NONE',  ( -31.40241232791079895, 1383.840297973970110, 229.3250844799549952 ) ) ;
#12811=CARTESIAN_POINT ( 'NONE',  ( -22.93874217539999805, 1382.980169263400057, 202.5862763507190323 ) ) ;
#12817=CARTESIAN_POINT ( 'NONE',  ( -10.24701828192700148, 1387.563789009890115, 217.6416621783679943 ) ) ;
#12819=DIRECTION ( 'NONE',  ( -0.05488031785798359874, -0.01377321100617858243, -0.9983979413892970500 ) ) ;
#12825=CARTESIAN_POINT ( 'NONE',  ( -94.74755207959219661, 1385.206845740749714, 294.8604545563650277 ) ) ;
#12839=CARTESIAN_POINT ( 'NONE',  ( -109.5275565480000068, 1385.603864912959807, 311.2689355842589976 ) ) ;
#12847=CARTESIAN_POINT ( 'NONE',  ( -8.030929497949999885, 1385.277656519309858, 218.7696094612490185 ) ) ;
#12901=CARTESIAN_POINT ( 'NONE',  ( -16.71457808692061420, 1379.711298523256573, 211.9342710108481072 ) ) ;
#12907=CARTESIAN_POINT ( 'NONE',  ( -96.47393723009329847, 1384.954577916420021, 310.3344438142669901 ) ) ;
#12908=CARTESIAN_POINT ( 'NONE',  ( -9.493009264660001278, 1386.944172907939901, 200.5464424274789792 ) ) ;
#12919=FACE_OUTER_BOUND ( 'NONE', #103210, .T. ) ;
#12949=CARTESIAN_POINT ( 'NONE',  ( -87.22487244391929551, 1384.624363658659831, 307.6774912203520671 ) ) ;
#12950=CARTESIAN_POINT ( 'NONE',  ( -41.91864753602830262, 1384.994678410510005, 214.8065739413959818 ) ) ;
#12967=CARTESIAN_POINT ( 'NONE',  ( -13.46522613409999991, 1379.673148676610026, 207.0022512300789685 ) ) ;
#12978=CARTESIAN_POINT ( 'NONE',  ( -68.31931742147419584, 1379.746951998870145, 279.9044409820210149 ) ) ;
#13002=CARTESIAN_POINT ( 'NONE',  ( -14.10694522062919987, 1379.843704623709982, 211.3636899608110014 ) ) ;
#13005=CARTESIAN_POINT ( 'NONE',  ( -64.34879093311614895, 1379.737658639894562, 270.9436941998574184 ) ) ;
#13009=CARTESIAN_POINT ( 'NONE',  ( -57.51057651963380124, 1384.658127080889926, 238.7961619097730193 ) ) ;
#13045=CARTESIAN_POINT ( 'NONE',  ( -12.28855869350000063, 1378.253616442990051, 210.0769077263690008 ) ) ;
#13072=CARTESIAN_POINT ( 'NONE',  ( -39.86052437841249940, 1384.788194491199874, 241.8866321169209925 ) ) ;
#13098=CARTESIAN_POINT ( 'NONE',  ( -67.06482036316408823, 1379.301523365260209, 281.5316999258700434 ) ) ;
#13110=CARTESIAN_POINT ( 'NONE',  ( -7.768842288840000165, 1384.896297089400150, 218.9179251193590119 ) ) ;
#13116=DIRECTION ( 'NONE',  ( -1.836970198721029688E-16, -1.000000000000000000, 0.000000000000000000 ) ) ;
#13129=CARTESIAN_POINT ( 'NONE',  ( -14.31913387383960057, 1380.323794892000024, 209.9058665205810144 ) ) ;
#13133=CARTESIAN_POINT ( 'NONE',  ( -52.67346242910000598, 1377.510081756269983, 241.2642412513589818 ) ) ;
#13144=CARTESIAN_POINT ( 'NONE',  ( -76.21403627649999635, 1383.779720587099746, 301.0850818666589817 ) ) ;
#13149=CARTESIAN_POINT ( 'NONE',  ( -50.64061620630000249, 1379.717051619300037, 241.3114574392589873 ) ) ;
#13155=CARTESIAN_POINT ( 'NONE',  ( -106.9828373484442494, 1391.808999926056458, 300.6260578302935187 ) ) ;
#13159=CARTESIAN_POINT ( 'NONE',  ( -23.62280757684879973, 1385.261635569479949, 222.7744051212729914 ) ) ;
#13188=CARTESIAN_POINT ( 'NONE',  ( -105.3802333100000084, 1391.003270672820008, 303.1242145234589884 ) ) ;
#13214=CARTESIAN_POINT ( 'NONE',  ( -90.27695662370000207, 1381.024254781289983, 306.9587642179589579 ) ) ;
#13219=CARTESIAN_POINT ( 'NONE',  ( -109.7182334529999963, 1384.930883209879994, 297.0861787735589701 ) ) ;
#13220=CARTESIAN_POINT ( 'NONE',  ( -7.989567385690000023, 1384.306347471770096, 199.5291465469090042 ) ) ;
#13225=CARTESIAN_POINT ( 'NONE',  ( -109.2578989990000053, 1384.875540820709830, 297.1358323108589730 ) ) ;
#13226=CARTESIAN_POINT ( 'NONE',  ( -12.28855869350000063, 1378.253616442990051, 210.0769077263690008 ) ) ;
#13237=ORIENTED_EDGE ( 'NONE', *, *, #1601, .F. ) ;
#13269=CARTESIAN_POINT ( 'NONE',  ( -17.14091472579860209, 1384.527013523339974, 201.0257602182319943 ) ) ;
#13275=ORIENTED_EDGE ( 'NONE', *, *, #499, .F. ) ;
#13282=CARTESIAN_POINT ( 'NONE',  ( -68.77190080519999071, 1379.747925807450201, 280.3125203366930123 ) ) ;
#13312=CARTESIAN_POINT ( 'NONE',  ( -107.4477384240240099, 1379.886883745280102, 299.0757736425410371 ) ) ;
#13313=ADVANCED_FACE ( 'NONE', ( #34439 ), #35611, .F. ) ;
#13332=CARTESIAN_POINT ( 'NONE',  ( -49.65267816373729914, 1383.812483723600053, 260.6283176093329530 ) ) ;
#13340=CARTESIAN_POINT ( 'NONE',  ( -23.75690532229999619, 1380.904381710259941, 220.2087197048589928 ) ) ;
#13347=CARTESIAN_POINT ( 'NONE',  ( -12.74756332158530014, 1389.858839731569788, 214.0101211577780020 ) ) ;
#13371=CARTESIAN_POINT ( 'NONE',  ( -109.9979373700000025, 1385.333188379740022, 311.4502719372590036 ) ) ;
#13381=CARTESIAN_POINT ( 'NONE',  ( -7.546363868560000299, 1385.222286201930046, 219.0767476026689735 ) ) ;
#13396=EDGE_LOOP ( 'NONE', ( #56907, #14508, #25513, #8047, #55753 ) ) ;
#13419=ORIENTED_EDGE ( 'NONE', *, *, #50033, .T. ) ;
#13427=CARTESIAN_POINT ( 'NONE',  ( -108.9413858983323280, 1381.821374029668959, 297.6754583912645558 ) ) ;
#13431=CARTESIAN_POINT ( 'NONE',  ( -106.5049786777409935, 1391.913060387289988, 305.4200656224640511 ) ) ;
#13438=CARTESIAN_POINT ( 'NONE',  ( -93.24395053702400560, 1384.962031755649832, 309.6487558849449897 ) ) ;
#13440=CARTESIAN_POINT ( 'NONE',  ( -8.406173068439999341, 1386.862502020539978, 199.9329045535289993 ) ) ;
#13453=CARTESIAN_POINT ( 'NONE',  ( -109.2523138997062802, 1387.517232177382994, 297.4607553404316604 ) ) ;
#13467=DIRECTION ( 'NONE',  ( 0.000000000000000000, 0.000000000000000000, -1.000000000000000000 ) ) ;
#13482=DIRECTION ( 'NONE',  ( -0.02617694830788819954, 0.9996573249755569268, 0.000000000000000000 ) ) ;
#13486=CARTESIAN_POINT ( 'NONE',  ( -101.2260141739269983, 1384.598541685300006, 310.9427063241110432 ) ) ;
#13487=CARTESIAN_POINT ( 'NONE',  ( -63.96209206476559217, 1385.081295340070028, 252.7243603260540112 ) ) ;
#13495=CARTESIAN_POINT ( 'NONE',  ( -109.6584371800000071, 1384.889060004170005, 311.3230551812590079 ) ) ;
#13520=CARTESIAN_POINT ( 'NONE',  ( -67.84113287159999572, 1379.747601269260031, 279.1899061516589882 ) ) ;
#13549=CARTESIAN_POINT ( 'NONE',  ( -12.61160395369999954, 1379.083170920169778, 208.5076010308980017 ) ) ;
#13550=CARTESIAN_POINT ( 'NONE',  ( -64.79513261177929451, 1379.738836812454565, 271.8835555406362801 ) ) ;
#13554=CARTESIAN_POINT ( 'NONE',  ( -86.70839285767250715, 1384.825211293280063, 290.2321663967470613 ) ) ;
#13609=LINE ( 'NONE', #81933, #51901 ) ;
#13619=CARTESIAN_POINT ( 'NONE',  ( -26.96405532890430123, 1384.839336572749971, 225.2101427744029820 ) ) ;
#13642=CARTESIAN_POINT ( 'NONE',  ( -94.10761133452021454, 1379.531657316930023, 303.8031716826509978 ) ) ;
#13653=CARTESIAN_POINT ( 'NONE',  ( -9.027091862569999847, 1384.059351705820063, 218.5832182276589890 ) ) ;
#13675=VERTEX_POINT ( 'NONE', #76720 ) ;
#13678=CARTESIAN_POINT ( 'NONE',  ( -63.58938922729999632, 1374.821258372890043, 269.7443356278590159 ) ) ;
#13694=CARTESIAN_POINT ( 'NONE',  ( -76.15242393239999785, 1384.064636357489917, 301.1578881669589691 ) ) ;
#13698=CARTESIAN_POINT ( 'NONE',  ( -58.05210803569999456, 1379.715589859269812, 257.1931556633589935 ) ) ;
#13709=CARTESIAN_POINT ( 'NONE',  ( -22.69270896030000273, 1385.265743060869909, 222.0224438233589979 ) ) ;
#13711=CARTESIAN_POINT ( 'NONE',  ( -53.96171695904460108, 1385.098550058179853, 269.7692938834680376 ) ) ;
#13729=AXIS2_PLACEMENT_3D ( 'NONE', #39399, #74122, #4161 ) ;
#13739=CARTESIAN_POINT ( 'NONE',  ( -105.6969335659999985, 1391.135062214819982, 302.0247559743589818 ) ) ;
#13741=CARTESIAN_POINT ( 'NONE',  ( -106.2334119559999976, 1391.826625675339983, 302.0221818237590128 ) ) ;
#13754=CARTESIAN_POINT ( 'NONE',  ( -4.237827489471030242E-15, 1374.913060387289988, 209.1218459572589836 ) ) ;
#13762=VERTEX_POINT ( 'NONE', #31 ) ;
#13763=CARTESIAN_POINT ( 'NONE',  ( -103.5772069679999845, 1380.769252584959986, 299.2318157808589945 ) ) ;
#13765=ORIENTED_EDGE ( 'NONE', *, *, #76451, .F. ) ;
#13796=CARTESIAN_POINT ( 'NONE',  ( -8.369546976630001467, 1384.842463915960025, 199.7754933009489946 ) ) ;
#13803=ORIENTED_EDGE ( 'NONE', *, *, #53675, .T. ) ;
#13811=CIRCLE ( 'NONE', #47809, 0.5000000000000004441 ) ;
#13819=CARTESIAN_POINT ( 'NONE',  ( -11.64339741151500007, 1384.514520786359981, 200.1925094546899970 ) ) ;
#13835=CARTESIAN_POINT ( 'NONE',  ( -68.74858467349999103, 1379.747915711970109, 280.1349441135590155 ) ) ;
#13869=CARTESIAN_POINT ( 'NONE',  ( -109.1450416020000063, 1385.242479493820156, 297.1468691531589457 ) ) ;
#13887=CARTESIAN_POINT ( 'NONE',  ( -43.53822014877789570, 1383.822559367279837, 248.2938733222130168 ) ) ;
#13896=CARTESIAN_POINT ( 'NONE',  ( -24.91449396329999999, 1379.865431598030000, 218.2371346374789880 ) ) ;
#13902=CARTESIAN_POINT ( 'NONE',  ( -10.24752963132049999, 1388.126283780050017, 217.1897018944860349 ) ) ;
#13904=CARTESIAN_POINT ( 'NONE',  ( -113.4000000000000057, 1390.913060387289988, 304.2218459572590064 ) ) ;
#13906=CARTESIAN_POINT ( 'NONE',  ( -106.5596784199999973, 1379.201018628780048, 300.2813271376589910 ) ) ;
#13919=CARTESIAN_POINT ( 'NONE',  ( -109.1646150049198809, 1384.938164062486749, 297.1326220263049436 ) ) ;
#13927=CARTESIAN_POINT ( 'NONE',  ( -109.3009594169999872, 1387.251231179749993, 311.0223495752589997 ) ) ;
#13953=CARTESIAN_POINT ( 'NONE',  ( -107.8638321499309995, 1378.913060387349788, 300.1214876574690607 ) ) ;
#13958=EDGE_LOOP ( 'NONE', ( #32359, #16684, #51628, #19888 ) ) ;
#13982=FACE_OUTER_BOUND ( 'NONE', #43509, .T. ) ;
#13992=FACE_OUTER_BOUND ( 'NONE', #98910, .T. ) ;
#14001=CARTESIAN_POINT ( 'NONE',  ( -92.83937824579700759, 1384.962964213820214, 309.5464475911989553 ) ) ;
#14002=CARTESIAN_POINT ( 'NONE',  ( -8.865249977160001293, 1387.451792102280024, 200.3692866900990168 ) ) ;
#14013=CARTESIAN_POINT ( 'NONE',  ( -106.6863336295694040, 1390.802642226108446, 300.1531170756869074 ) ) ;
#14037=CARTESIAN_POINT ( 'NONE',  ( -105.0307287566989061, 1380.923348513794508, 308.4048763095673280 ) ) ;
#14046=CARTESIAN_POINT ( 'NONE',  ( -61.65894565632150659, 1385.069567178810075, 247.6034208562279844 ) ) ;
#14054=CARTESIAN_POINT ( 'NONE',  ( -109.9849080340000000, 1384.910086089010065, 311.4561084402590154 ) ) ;
#14059=CARTESIAN_POINT ( 'NONE',  ( -109.9861441850000006, 1384.675965057090025, 311.4500065002590077 ) ) ;
#14072=CARTESIAN_POINT ( 'NONE',  ( -5.369546485720880113, 1374.928881103789990, 203.3687134724160046 ) ) ;
#14079=CARTESIAN_POINT ( 'NONE',  ( -67.82383404051370235, 1379.746049001880010, 279.2023482137329893 ) ) ;
#14082=CARTESIAN_POINT ( 'NONE',  ( -9.881278461464678031, 1379.739605549548514, 216.5635243919133188 ) ) ;
#14090=CARTESIAN_POINT ( 'NONE',  ( -106.2140063875329901, 1378.913060387799987, 305.8740827694030031 ) ) ;
#14113=CARTESIAN_POINT ( 'NONE',  ( -76.07930854709739776, 1384.773566694879946, 277.2872448374639589 ) ) ;
#14185=CARTESIAN_POINT ( 'NONE',  ( -57.94140768939789865, 1384.704083737000019, 277.3428793058350266 ) ) ;
#14189=CARTESIAN_POINT ( 'NONE',  ( -105.8044893139999942, 1378.913060387289988, 303.5347832593589601 ) ) ;
#14202=CARTESIAN_POINT ( 'NONE',  ( -12.22392939165850123, 1377.774275016259935, 210.6554241722059828 ) ) ;
#14204=AXIS2_PLACEMENT_3D ( 'NONE', #39833, #73996, #6222 ) ;
#14212=CARTESIAN_POINT ( 'NONE',  ( -3.771520276690010220, 1379.037774784969997, 211.6703177581799764 ) ) ;
#14215=CARTESIAN_POINT ( 'NONE',  ( -21.75077721616250059, 1379.626252247850061, 213.4816723946260026 ) ) ;
#14222=FACE_OUTER_BOUND ( 'NONE', #30815, .T. ) ;
#14241=CARTESIAN_POINT ( 'NONE',  ( -109.3216456436046968, 1387.209460202328955, 311.0349939649406110 ) ) ;
#14244=CARTESIAN_POINT ( 'NONE',  ( -13.10979329346079858, 1380.091434411379851, 209.5250314328370109 ) ) ;
#14248=CARTESIAN_POINT ( 'NONE',  ( -30.31557410699999977, 1377.728231664160148, 212.6771353113689713 ) ) ;
#14262=CARTESIAN_POINT ( 'NONE',  ( -27.62594988560000075, 1384.837137189770147, 225.6315537474590371 ) ) ;
#14274=CARTESIAN_POINT ( 'NONE',  ( -39.28171750389999772, 1390.901355467679878, 224.3483216179589874 ) ) ;
#14276=CARTESIAN_POINT ( 'NONE',  ( -44.66018671116690086, 1385.154557438659822, 250.8453420411730406 ) ) ;
#14303=CARTESIAN_POINT ( 'NONE',  ( -106.9455967239999978, 1390.237690493389891, 299.5801972406590039 ) ) ;
#14314=B_SPLINE_SURFACE_WITH_KNOTS ( 'NONE', 5, 5, ( 
 ( #17336, #78387, #76176, #69460, #104133, #52093 ),
 ( #35836, #77293, #8964, #42574, #60499, #85663 ),
 ( #59398, #43135, #9515, #10635, #85114, #27419 ),
 ( #61602, #102461, #95735, #86780, #591, #110325 ),
 ( #18999, #67793, #1695, #34169, #10069, #93509 ),
 ( #61068, #34718, #70019, #53199, #86224, #25195 ),
 ( #51530, #68909, #103011, #8402, #87339, #26307 ),
 ( #33598, #44243, #43683, #16781, #50985, #76725 ),
 ( #94620, #38, #68355, #17896, #35275, #94067 ) ),
 .UNSPECIFIED., .F., .F., .F.,
 ( 6, 3, 6 ),
 ( 6, 6 ),
 ( 1.832321132619999986E-17, 6.516940428549999886, 11.47905148820000143 ),
 ( 0.000000000000000000, 1.000000000000000000 ),
 .UNSPECIFIED. ) ;
#14324=CARTESIAN_POINT ( 'NONE',  ( -113.4000000000000057, 1381.047475678389901, 309.3701288452589893 ) ) ;
#14330=CARTESIAN_POINT ( 'NONE',  ( -8.862265221084019373, 1384.931617321382419, 218.6851228964859502 ) ) ;
#14354=CARTESIAN_POINT ( 'NONE',  ( -8.383874734839999121, 1384.494374329680113, 199.7996924129390095 ) ) ;
#14370=ORIENTED_EDGE ( 'NONE', *, *, #70946, .T. ) ;
#14376=CARTESIAN_POINT ( 'NONE',  ( -22.89435465436789841, 1384.539855335990069, 202.5339165971940076 ) ) ;
#14386=CIRCLE ( 'NONE', #7287, 8.432239102140000497 ) ;
#14431=ORIENTED_EDGE ( 'NONE', *, *, #82837, .T. ) ;
#14441=CARTESIAN_POINT ( 'NONE',  ( -43.78017172700090498, 1383.822166568830198, 248.7628566075970014 ) ) ;
#14448=DIRECTION ( 'NONE',  ( -1.076084536626781954E-17, -1.000000000000000000, -4.313860721084074369E-17 ) ) ;
#14454=CARTESIAN_POINT ( 'NONE',  ( -13.38802240389999909, 1383.860181226410077, 218.7963554078490063 ) ) ;
#14460=CARTESIAN_POINT ( 'NONE',  ( -8.779303069688410233, 1386.002643005009986, 218.5317853082520116 ) ) ;
#14465=CARTESIAN_POINT ( 'NONE',  ( -105.8704711980000042, 1378.498029401629992, 301.8910949082590491 ) ) ;
#14484=CARTESIAN_POINT ( 'NONE',  ( -109.5956166280000019, 1386.715462780010057, 311.2107475812589996 ) ) ;
#14508=ORIENTED_EDGE ( 'NONE', *, *, #94757, .T. ) ;
#14515=CARTESIAN_POINT ( 'NONE',  ( -64.53985313679999081, 1384.829190178189947, 254.0316580881589630 ) ) ;
#14542=CARTESIAN_POINT ( 'NONE',  ( -107.7075879675156358, 1380.190251876901129, 298.7630690546642427 ) ) ;
#14555=CARTESIAN_POINT ( 'NONE',  ( -97.11742683014449540, 1384.953084665809911, 310.4397664338810046 ) ) ;
#14556=CARTESIAN_POINT ( 'NONE',  ( -9.634077209289999999, 1386.855370323769876, 200.5463740245589861 ) ) ;
#14570=CARTESIAN_POINT ( 'NONE',  ( -109.9857364230449974, 1384.899971927750130, 311.4562996732899478 ) ) ;
#14605=CARTESIAN_POINT ( 'NONE',  ( -62.23936251973370304, 1385.072491325380042, 248.8854521166869915 ) ) ;
#14619=CARTESIAN_POINT ( 'NONE',  ( -109.8144715679999877, 1384.521880215379952, 311.3640776482590127 ) ) ;
#14639=CARTESIAN_POINT ( 'NONE',  ( -68.45375916347519762, 1379.747171630710000, 280.0545672679439804 ) ) ;
#14642=CARTESIAN_POINT ( 'NONE',  ( -8.226710716830746506, 1382.151431053786609, 218.4368142409218194 ) ) ;
#14651=CARTESIAN_POINT ( 'NONE',  ( -107.7594617770490117, 1378.913060387289988, 308.1713896475600336 ) ) ;
#14659=ORIENTED_EDGE ( 'NONE', *, *, #37893, .T. ) ;
#14673=CARTESIAN_POINT ( 'NONE',  ( -80.90462325147591116, 1384.798765408159852, 284.2668994243870202 ) ) ;
#14741=CARTESIAN_POINT ( 'NONE',  ( -43.87927512900789395, 1384.769549923549903, 249.3322899781709907 ) ) ;
#14742=CARTESIAN_POINT ( 'NONE',  ( -107.0856175946619970, 1391.913060387289988, 301.5308894922570175 ) ) ;
#14746=CARTESIAN_POINT ( 'NONE',  ( -105.5765342570000058, 1378.949837160079824, 302.9213429863589795 ) ) ;
#14767=CARTESIAN_POINT ( 'NONE',  ( -27.34872825612519875, 1378.876396125770043, 217.1833578772759950 ) ) ;
#14770=CARTESIAN_POINT ( 'NONE',  ( -31.51240728630000376, 1379.723496875969886, 219.1466601182590068 ) ) ;
#14797=CARTESIAN_POINT ( 'NONE',  ( -107.4877904035150067, 1389.702161918033880, 309.4250478887230997 ) ) ;
#14799=CARTESIAN_POINT ( 'NONE',  ( -12.63531666014029931, 1379.388864909599988, 208.8707713015120078 ) ) ;
#14803=CARTESIAN_POINT ( 'NONE',  ( -36.43074434249999172, 1380.172836988449944, 219.9641098163590129 ) ) ;
#14806=ORIENTED_EDGE ( 'NONE', *, *, #50033, .F. ) ;
#14815=CARTESIAN_POINT ( 'NONE',  ( -32.14702491180000266, 1384.162411493540048, 229.9166993473590139 ) ) ;
#14827=CARTESIAN_POINT ( 'NONE',  ( -69.40052021539999316, 1389.408898824169910, 290.4326261031590093 ) ) ;
#14829=CARTESIAN_POINT ( 'NONE',  ( -40.13732683962579983, 1385.181215360810029, 242.3489691607209977 ) ) ;
#14853=CARTESIAN_POINT ( 'NONE',  ( -107.4403222199999988, 1387.882953355429891, 298.2873657394590055 ) ) ;
#14856=CARTESIAN_POINT ( 'NONE',  ( -105.8808422670000056, 1391.420045099660001, 301.8793707204590078 ) ) ;
#14909=ORIENTED_EDGE ( 'NONE', *, *, #7895, .F. ) ;
#14924=CARTESIAN_POINT ( 'NONE',  ( -9.123736379228210680, 1384.508619151900120, 199.9712811155520171 ) ) ;
#14938=CARTESIAN_POINT ( 'NONE',  ( -68.77190080519999071, 1379.747925807450201, 280.3125203366930123 ) ) ;
#14961=ORIENTED_EDGE ( 'NONE', *, *, #20045, .F. ) ;
#14973=CARTESIAN_POINT ( 'NONE',  ( -106.7897227899999990, 1379.694571751269905, 299.8550812676590454 ) ) ;
#14989=CARTESIAN_POINT ( 'NONE',  ( -41.04806346289370111, 1383.826527834990202, 243.6424592814190078 ) ) ;
#14997=CARTESIAN_POINT ( 'NONE',  ( -55.58991683120000005, 1380.431293333419944, 241.3934034463590024 ) ) ;
#15007=CARTESIAN_POINT ( 'NONE',  ( -103.6765714240000023, 1379.937512265609939, 302.8207899414589974 ) ) ;
#15009=DIRECTION ( 'NONE',  ( -1.000000000000000000, 0.000000000000000000, 0.000000000000000000 ) ) ;
#15025=CARTESIAN_POINT ( 'NONE',  ( -109.8667940760000050, 1385.713658988820043, 311.3767387042589689 ) ) ;
#15055=VERTEX_POINT ( 'NONE', #109051 ) ;
#15056=CARTESIAN_POINT ( 'NONE',  ( -75.49415276370000072, 1384.770980541030212, 276.6885382114589902 ) ) ;
#15060=CARTESIAN_POINT ( 'NONE',  ( -106.9474174639999973, 1379.784802923450115, 308.7531441963589600 ) ) ;
#15090=CARTESIAN_POINT ( 'NONE',  ( -11.81825512610000040, 1379.647206402889879, 214.1905352636190116 ) ) ;
#15098=CARTESIAN_POINT ( 'NONE',  ( -8.162781193059998941, 1386.079686460999937, 199.6931303246190055 ) ) ;
#15111=CARTESIAN_POINT ( 'NONE',  ( -108.1042440287333193, 1389.151938345616145, 298.3733779900309173 ) ) ;
#15128=FACE_OUTER_BOUND ( 'NONE', #24934, .T. ) ;
#15131=CARTESIAN_POINT ( 'NONE',  ( -11.15738487964140013, 1390.939238811560017, 203.8452351040699853 ) ) ;
#15135=CARTESIAN_POINT ( 'NONE',  ( -104.5385623544569285, 1380.577965172966742, 307.6528342442834969 ) ) ;
#15141=CARTESIAN_POINT ( 'NONE',  ( -12.95282315900000114, 1379.746587813670203, 210.9367672650590180 ) ) ;
#15143=CARTESIAN_POINT ( 'NONE',  ( -53.74734980331459866, 1385.033272470989914, 231.5355373840500022 ) ) ;
#15144=CARTESIAN_POINT ( 'NONE',  ( -11.08783833967420129, 1391.913060387289988, 212.3049891749950291 ) ) ;
#15151=CARTESIAN_POINT ( 'NONE',  ( -109.3074459189999885, 1384.922471985850279, 311.2646699492589732 ) ) ;
#15154=CARTESIAN_POINT ( 'NONE',  ( -109.1345257920000051, 1384.812366243020051, 311.2635679502590165 ) ) ;
#15173=CARTESIAN_POINT ( 'NONE',  ( -68.75556014300001095, 1379.747888069970031, 280.3281857314590297 ) ) ;
#15175=CARTESIAN_POINT ( 'NONE',  ( -9.268081120116850258, 1380.504154720858878, 217.3372005545678292 ) ) ;
#15196=CARTESIAN_POINT ( 'NONE',  ( -14.08142637225379978, 1379.709117121690042, 211.5303641152310092 ) ) ;
#15206=CARTESIAN_POINT ( 'NONE',  ( -10.57866586919999996, 1391.913060534260012, 214.0410642522289777 ) ) ;
#15207=CARTESIAN_POINT ( 'NONE',  ( -70.27615847020030060, 1384.739003949510106, 266.4825429262279499 ) ) ;
#15232=B_SPLINE_CURVE_WITH_KNOTS ( 'NONE', 3,
 ( #103412, #26717, #24771, #92545, #50017, #39402, #84149, #99285, #15813, #66832, #66290, #30995, #48372, #100939, #32103, #82515, #75767, #7450, #48931, #67386, #90903, #40499, #74125, #41613, #24235, #32655, #100407, #22561, #58967, #83593, #14742, #6892, #74676, #108255, #49472, #108810, #109915 ),
 .UNSPECIFIED., .F., .F.,
 ( 4, 3, 3, 3, 3, 3, 3, 3, 3, 3, 3, 3, 4 ),
 ( -8.626417477929999578, -8.230297350330690875, -7.288362325489999627, -6.788184810323580010, -5.950307173050000564, -5.270875643514309594, -4.379860848525059858, -3.500078386716319656, -3.080773698474470024, -2.517080355727370211, -1.669614525887570089, -0.8307986329775687295, 0.000000000000000000 ),
 .UNSPECIFIED. ) ;
#15246=CARTESIAN_POINT ( 'NONE',  ( -67.65174119259999941, 1379.761245408810282, 278.4852794438589854 ) ) ;
#15270=CARTESIAN_POINT ( 'NONE',  ( -12.31752010984839885, 1377.944433743309901, 209.1218459601290078 ) ) ;
#15278=CARTESIAN_POINT ( 'NONE',  ( -56.94594514817760000, 1384.708275839130010, 275.5160223163470050 ) ) ;
#15285=CARTESIAN_POINT ( 'NONE',  ( -4.237827489471030242E-15, 1374.913060387289988, 209.1218459572589836 ) ) ;
#15286=CARTESIAN_POINT ( 'NONE',  ( -9.906269641306360896, 1380.355646941639407, 201.6945993121081528 ) ) ;
#15297=CARTESIAN_POINT ( 'NONE',  ( -12.35647260227639954, 1378.853423139930101, 211.4877825593519844 ) ) ;
#15307=CARTESIAN_POINT ( 'NONE',  ( -39.30087362371570237, 1378.765606774250045, 229.0543489963469881 ) ) ;
#15309=CARTESIAN_POINT ( 'NONE',  ( -29.90839080569999808, 1379.722162691039784, 217.8816187629589933 ) ) ;
#15342=CARTESIAN_POINT ( 'NONE',  ( -3.771520293490000064, 1379.460406650380037, 206.9293833799489732 ) ) ;
#15349=EDGE_CURVE ( 'NONE', #27006, #101083, #36803, .T. ) ;
#15357=CARTESIAN_POINT ( 'NONE',  ( -47.37590574939999755, 1384.752751010099928, 256.2773158601589785 ) ) ;
#15374=CARTESIAN_POINT ( 'NONE',  ( -73.11479823269999656, 1385.127942832860072, 272.3424178700590232 ) ) ;
#15375=ORIENTED_EDGE ( 'NONE', *, *, #78509, .T. ) ;
#15376=CARTESIAN_POINT ( 'NONE',  ( -43.63441986346529688, 1385.160729704950199, 248.8361117960110107 ) ) ;
#15385=CARTESIAN_POINT ( 'NONE',  ( -7.544898869409998987, 1384.902875507950057, 219.0876726552290279 ) ) ;
#15387=ORIENTED_EDGE ( 'NONE', *, *, #46251, .T. ) ;
#15402=CARTESIAN_POINT ( 'NONE',  ( -106.2112533720000016, 1391.321897446320236, 300.8491284572590416 ) ) ;
#15422=CARTESIAN_POINT ( 'NONE',  ( -12.02612939183720009, 1377.659857216290220, 211.7505375168460091 ) ) ;
#15442=ORIENTED_EDGE ( 'NONE', *, *, #67205, .F. ) ;
#15463=CARTESIAN_POINT ( 'NONE',  ( -5.153093391039999638, 1380.759461119849902, 203.4632808174290233 ) ) ;
#15474=CARTESIAN_POINT ( 'NONE',  ( -30.25652781387339729, 1384.556785492720110, 205.7254385433210189 ) ) ;
#15482=CARTESIAN_POINT ( 'NONE',  ( -12.96458870010000020, 1380.564911143250129, 203.9320203105589826 ) ) ;
#15486=CARTESIAN_POINT ( 'NONE',  ( -68.76593665590000626, 1379.747941725510145, 280.1891108434590478 ) ) ;
#15494=CARTESIAN_POINT ( 'NONE',  ( -1.512515161746819920E-15, 1385.198152793140025, 218.6122691739390120 ) ) ;
#15509=DIRECTION ( 'NONE',  ( 1.000000000000000000, 0.000000000000000000, 0.000000000000000000 ) ) ;
#15528=ORIENTED_EDGE ( 'NONE', *, *, #31835, .F. ) ;
#15537=CARTESIAN_POINT ( 'NONE',  ( -65.17440126354809138, 1383.790278610199948, 288.6850384825009996 ) ) ;
#15542=ORIENTED_EDGE ( 'NONE', *, *, #103236, .T. ) ;
#15544=CARTESIAN_POINT ( 'NONE',  ( -57.73766270559999469, 1379.143380400379783, 257.1610347018590232 ) ) ;
#15553=CARTESIAN_POINT ( 'NONE',  ( -107.1873477440000073, 1379.571931949629970, 299.3438537678590023 ) ) ;
#15570=CARTESIAN_POINT ( 'NONE',  ( -106.7983762909999967, 1389.555420353100089, 308.8839675026590044 ) ) ;
#15598=CARTESIAN_POINT ( 'NONE',  ( -73.12043787219998592, 1384.880583958779880, 272.3393879815590140 ) ) ;
#15606=EDGE_LOOP ( 'NONE', ( #103627, #50737, #93540, #5336, #99801 ) ) ;
#15609=CARTESIAN_POINT ( 'NONE',  ( -10.92223504695139980, 1391.913060387089899, 205.7923380047099897 ) ) ;
#15629=CARTESIAN_POINT ( 'NONE',  ( -10.60340555500000015, 1379.609174620120029, 215.5963861307990044 ) ) ;
#15636=CARTESIAN_POINT ( 'NONE',  ( -13.72218023960000011, 1389.845687919130114, 205.4181164005090068 ) ) ;
#15641=CARTESIAN_POINT ( 'NONE',  ( -9.129309581573130217, 1383.864686136899991, 218.5281989956060045 ) ) ;
#15646=CARTESIAN_POINT ( 'NONE',  ( -106.8244771589985049, 1390.652608569862423, 299.9266001010461764 ) ) ;
#15657=( BOUNDED_CURVE ( )  B_SPLINE_CURVE ( 3, ( #78733, #44588, #87699, #3707 ),
 .UNSPECIFIED., .F., .T. ) 
 B_SPLINE_CURVE_WITH_KNOTS ( ( 4, 4 ),
 ( 3.320448054550920070, 3.390722914990644821 ),
 .UNSPECIFIED. ) 
 CURVE ( )  GEOMETRIC_REPRESENTATION_ITEM ( )  RATIONAL_B_SPLINE_CURVE ( ( 1.000000000000000000, 0.9995884960067018543, 0.9995884960067018543, 1.000000000000000000 ) ) 
 REPRESENTATION_ITEM ( '' )  );
#15672=CARTESIAN_POINT ( 'NONE',  ( -105.6076294414992418, 1381.326326253046773, 309.0868219927184555 ) ) ;
#15678=CARTESIAN_POINT ( 'NONE',  ( -14.13509333269999857, 1379.975727635469866, 211.1783289813689919 ) ) ;
#15680=CARTESIAN_POINT ( 'NONE',  ( -58.69938589393059658, 1385.055105096270154, 241.2266681709880061 ) ) ;
#15691=FACE_OUTER_BOUND ( 'NONE', #92258, .T. ) ;
#15710=CARTESIAN_POINT ( 'NONE',  ( -68.52665777820699589, 1379.747389946890053, 280.1435722370280246 ) ) ;
#15713=ORIENTED_EDGE ( 'NONE', *, *, #35715, .T. ) ;
#15737=CARTESIAN_POINT ( 'NONE',  ( -12.61779677260000021, 1379.111305426719809, 208.5419189764980104 ) ) ;
#15741=CARTESIAN_POINT ( 'NONE',  ( -11.28091541760000105, 1391.913060106340026, 212.5574219731489620 ) ) ;
#15742=CARTESIAN_POINT ( 'NONE',  ( -78.28135749134220589, 1384.785472859150104, 280.7109069974439990 ) ) ;
#15750=CARTESIAN_POINT ( 'NONE',  ( 12.48860275614654824, 1384.926148861439970, 208.5962672545927603 ) ) ;
#15759=CARTESIAN_POINT ( 'NONE',  ( -47.60661184359999254, 1379.710340994259923, 235.3636715871589900 ) ) ;
#15794=CARTESIAN_POINT ( 'NONE',  ( -10.17157269315458556, 1390.403795797951034, 216.1384918992431494 ) ) ;
#15812=CARTESIAN_POINT ( 'NONE',  ( -53.13680734357709667, 1384.725240562959925, 268.1326697647110109 ) ) ;
#15813=CARTESIAN_POINT ( 'NONE',  ( -106.4392312446289992, 1391.913060387289988, 303.5569487479260147 ) ) ;
#15815=CARTESIAN_POINT ( 'NONE',  ( -106.8359495019999912, 1379.429462365020072, 299.8958288151589500 ) ) ;
#15821=CARTESIAN_POINT ( 'NONE',  ( -12.18433968541703116, 1377.735202854164072, 207.2844700481445841 ) ) ;
#15844=CARTESIAN_POINT ( 'NONE',  ( -7.459448365662689540, 1377.973318082249989, 211.7927975196730017 ) ) ;
#15846=CARTESIAN_POINT ( 'NONE',  ( -29.87190587263160069, 1379.676854917029914, 217.9309857436469997 ) ) ;
#15853=CARTESIAN_POINT ( 'NONE',  ( -106.3126565290000087, 1379.599899938080171, 307.8895711306589646 ) ) ;
#15857=DIRECTION ( 'NONE',  ( -1.836970198721029688E-16, -1.000000000000000000, 0.000000000000000000 ) ) ;
#15877=CARTESIAN_POINT ( 'NONE',  ( -106.6554729947317526, 1390.652008648487936, 308.2807419479074724 ) ) ;
#15882=EDGE_CURVE ( 'NONE', #99683, #26950, #94087, .T. ) ;
#15886=CARTESIAN_POINT ( 'NONE',  ( -19.31603552179999994, 1379.367063215299822, 208.2524156231729933 ) ) ;
#15900=CARTESIAN_POINT ( 'NONE',  ( -109.9987472819999965, 1384.028067710840105, 311.1749645552590096 ) ) ;
#15915=CARTESIAN_POINT ( 'NONE',  ( -61.45349693709999883, 1390.736557064060207, 266.8826925622589670 ) ) ;
#15917=CARTESIAN_POINT ( 'NONE',  ( -40.39009907441349867, 1385.179773408669917, 242.7937635241629835 ) ) ;
#15926=CARTESIAN_POINT ( 'NONE',  ( -7.769235965580000070, 1384.905329033560065, 218.9178834839189847 ) ) ;
#15939=B_SPLINE_CURVE_WITH_KNOTS ( 'NONE', 3,
 ( #30769, #64948, #99062, #22341, #56541, #6115, #13953, #5579, #39729, #73895, #108021, #31318, #65501, #22894, #48699, #74456, #11517, #94962, #26639, #2586, #36710, #27206, #61389, #45692, #43465, #103908, #96623, #28869, #79277, #95508, #18779, #77611, #52977, #922, #28313, #79831, #78151, #18230, #35045, #104459, #105020, #27752, #9300, #10398, #70903, #105582, #3137, #9847, #37271, #62504, #19334, #61945 ),
 .UNSPECIFIED., .F., .F.,
 ( 4, 3, 3, 3, 3, 3, 3, 3, 3, 3, 3, 3, 3, 3, 3, 3, 3, 4 ),
 ( -13.54897587289999983, -13.17531786724759968, -12.47907539720000081, -12.15554221928960033, -11.39789929992029904, -10.56585940365520138, -9.637960392618930783, -8.269156193220000617, -7.517475011647490213, -6.592826046528001527, -5.699782786179998340, -5.491406205670669394, -4.662291499253420568, -3.881037718147339888, -3.127721678440000375, -2.865801632923298925, -2.150110822952852274, -1.461586381269999180 ),
 .UNSPECIFIED. ) ;
#15945=CARTESIAN_POINT ( 'NONE',  ( -108.6385992050000056, 1386.360677242800193, 297.3882613995589850 ) ) ;
#15979=CARTESIAN_POINT ( 'NONE',  ( -16.14609365299999766, 1380.312263807889849, 210.2238755387789979 ) ) ;
#15998=CARTESIAN_POINT ( 'NONE',  ( -8.164317912589998727, 1384.513847593510036, 199.6670242607489740 ) ) ;
#16018=CARTESIAN_POINT ( 'NONE',  ( -113.4000000000000057, 1379.105522877179965, 302.6503168488589495 ) ) ;
#16024=CARTESIAN_POINT ( 'NONE',  ( -37.07348200565930085, 1384.574303191529907, 210.3284201765650039 ) ) ;
#16025=CARTESIAN_POINT ( 'NONE',  ( -14.52363634152899863, 1379.696035566400042, 208.2603442536380101 ) ) ;
#16038=CARTESIAN_POINT ( 'NONE',  ( -68.45900093969999034, 1379.747219870859908, 279.4339011000590176 ) ) ;
#16059=CARTESIAN_POINT ( 'NONE',  ( -8.873656775930450991, 1385.220332894750072, 218.6703658329330153 ) ) ;
#16088=CARTESIAN_POINT ( 'NONE',  ( -62.13084746230200039, 1383.793921180840016, 284.1282107610300045 ) ) ;
#16098=CARTESIAN_POINT ( 'NONE',  ( -37.85704848470000172, 1380.929536399250082, 234.3704980780590006 ) ) ;
#16105=CARTESIAN_POINT ( 'NONE',  ( -109.1112710710209939, 1384.400207420500237, 313.2414003153020303 ) ) ;
#16109=CARTESIAN_POINT ( 'NONE',  ( -108.0400389039999851, 1380.595742417440078, 298.4240030958590069 ) ) ;
#16121=ORIENTED_EDGE ( 'NONE', *, *, #85697, .F. ) ;
#16130=CARTESIAN_POINT ( 'NONE',  ( -108.2565521540000049, 1386.661487099380111, 310.8214570342590264 ) ) ;
#16138=CARTESIAN_POINT ( 'NONE',  ( -13.72218023960000011, 1389.845687919130114, 205.4181164005090068 ) ) ;
#16168=CARTESIAN_POINT ( 'NONE',  ( -11.22869580998730044, 1391.913060387200176, 206.6514090535289938 ) ) ;
#16189=CARTESIAN_POINT ( 'NONE',  ( -12.29441139609999922, 1379.981535577770046, 214.2870256391589976 ) ) ;
#16196=CARTESIAN_POINT ( 'NONE',  ( -12.44451260820000016, 1390.433100873249941, 205.6563933776689908 ) ) ;
#16217=CARTESIAN_POINT ( 'NONE',  ( -15.70334894381019986, 1383.857901626470039, 219.4107432652749878 ) ) ;
#16229=DIRECTION ( 'NONE',  ( -1.000000000000000000, 1.836970198721029688E-16, 0.000000000000000000 ) ) ;
#16233=CARTESIAN_POINT ( 'NONE',  ( -104.5039857551601443, 1380.553604562968530, 307.5917977560359873 ) ) ;
#16240=CARTESIAN_POINT ( 'NONE',  ( -80.12029132004148835, 1385.158018703190010, 283.2668441326100037 ) ) ;
#16241=CARTESIAN_POINT ( 'NONE',  ( -11.22781813603899792, 1391.913060387289988, 211.9257311578400049 ) ) ;
#16268=CARTESIAN_POINT ( 'NONE',  ( -68.47067291010000645, 1379.747730938300265, 280.0399411558590259 ) ) ;
#16299=CARTESIAN_POINT ( 'NONE',  ( -11.38303023819999993, 1391.412213333949921, 213.8762289909089986 ) ) ;
#16300=CARTESIAN_POINT ( 'NONE',  ( -97.56323068563240497, 1384.866207655270046, 295.7272966331869952 ) ) ;
#16319=CARTESIAN_POINT ( 'NONE',  ( -60.03859995180000197, 1379.727664477899907, 261.7965084652589667 ) ) ;
#16334=ORIENTED_EDGE ( 'NONE', *, *, #31174, .F. ) ;
#16335=CARTESIAN_POINT ( 'NONE',  ( -8.848352085069999262, 1384.928008052449968, 199.9247643512989896 ) ) ;
#16350=MECHANICAL_DESIGN_GEOMETRIC_PRESENTATION_REPRESENTATION('',(#27106),#86153);
#16354=CARTESIAN_POINT ( 'NONE',  ( -8.297485596343202374, 1387.805263089111804, 218.3696328644297751 ) ) ;
#16371=CARTESIAN_POINT ( 'NONE',  ( -55.35023455054019337, 1384.715211743480040, 272.4935865345279922 ) ) ;
#16372=CARTESIAN_POINT ( 'NONE',  ( -22.90005503110699792, 1384.955863742640076, 202.5115359936190202 ) ) ;
#16374=CARTESIAN_POINT ( 'NONE',  ( -106.9496064929999903, 1379.185917738360104, 299.9942942488589779 ) ) ;
#16378=CARTESIAN_POINT ( 'NONE',  ( -9.449812779362575910, 1380.957496575889991, 201.0964360788809131 ) ) ;
#16387=CARTESIAN_POINT ( 'NONE',  ( -12.10275407134929893, 1377.603811883519938, 211.3932643068179971 ) ) ;
#16398=CARTESIAN_POINT ( 'NONE',  ( -24.48072446064930219, 1378.898509916240073, 215.5032166125519950 ) ) ;
#16401=CARTESIAN_POINT ( 'NONE',  ( -52.38592625916200518, 1379.720821623890060, 249.9316393081959973 ) ) ;
#16403=VERTEX_POINT ( 'NONE', #106314 ) ;
#16408=CARTESIAN_POINT ( 'NONE',  ( -109.3074459329999968, 1384.922460900670103, 311.2646700692590116 ) ) ;
#16434=CARTESIAN_POINT ( 'NONE',  ( -3.771520293490000064, 1376.318813996809922, 206.9293833799489732 ) ) ;
#16435=ORIENTED_EDGE ( 'NONE', *, *, #10873, .F. ) ;
#16438=CARTESIAN_POINT ( 'NONE',  ( 1.715743480078970019E-15, 1374.913060387289988, 209.1218459572589836 ) ) ;
#16460=CARTESIAN_POINT ( 'NONE',  ( -58.30163007960000243, 1385.052442321870103, 240.0694839391589994 ) ) ;
#16462=CARTESIAN_POINT ( 'NONE',  ( -77.48449076556670434, 1385.000788814369798, 302.0789985806010236 ) ) ;
#16472=CARTESIAN_POINT ( 'NONE',  ( -7.768842288750000158, 1384.896297089410155, 218.9179251193689879 ) ) ;
#16474=CARTESIAN_POINT ( 'NONE',  ( -107.3898476250000016, 1380.885722407379944, 309.4972360872590116 ) ) ;
#16486=CARTESIAN_POINT ( 'NONE',  ( -105.4593524538789211, 1391.263055996386356, 303.4133149664163511 ) ) ;
#16511=CARTESIAN_POINT ( 'NONE',  ( -13.71394807775421754, 1379.587227311490551, 211.8543316273178334 ) ) ;
#16520=CARTESIAN_POINT ( 'NONE',  ( -12.30145601893210028, 1378.350113758880070, 209.9325833000719967 ) ) ;
#16555=CARTESIAN_POINT ( 'NONE',  ( -113.4000000000000057, 1376.913060387289988, 301.4143084471589873 ) ) ;
#16560=CARTESIAN_POINT ( 'NONE',  ( -32.90424402952790217, 1384.563281534569796, 207.2982514105669907 ) ) ;
#16562=CARTESIAN_POINT ( 'NONE',  ( -108.9389063659999977, 1385.729741725900112, 311.1830050262590248 ) ) ;
#16567=CARTESIAN_POINT ( 'NONE',  ( -57.28255472204047294, 1379.717548595288235, 260.3994659975323884 ) ) ;
#16571=CARTESIAN_POINT ( 'NONE',  ( -68.55439833990000409, 1379.747438846910200, 279.6432152850590001 ) ) ;
#16580=CARTESIAN_POINT ( 'NONE',  ( -5.958828918510000072, 1385.041501276899908, 218.5259373746190192 ) ) ;
#16587=CARTESIAN_POINT ( 'NONE',  ( -113.4000000000000057, 1384.899971913130003, 304.2218459572590064 ) ) ;
#16628=CARTESIAN_POINT ( 'NONE',  ( -70.66573123358719499, 1383.784603572710239, 295.5469044946160011 ) ) ;
#16634=ORIENTED_EDGE ( 'NONE', *, *, #20132, .F. ) ;
#16637=CARTESIAN_POINT ( 'NONE',  ( -59.79588189159999700, 1380.471087561269997, 250.5313864223589917 ) ) ;
#16642=CARTESIAN_POINT ( 'NONE',  ( -8.925728462962421617, 1385.954551176779887, 218.5383989427139966 ) ) ;
#16648=CARTESIAN_POINT ( 'NONE',  ( -109.7649665430000141, 1383.250791452569956, 297.1361542659589645 ) ) ;
#16670=CARTESIAN_POINT ( 'NONE',  ( -105.6600088659999983, 1389.882499440619995, 307.5167961107590031 ) ) ;
#16684=ORIENTED_EDGE ( 'NONE', *, *, #20788, .T. ) ;
#16702=CARTESIAN_POINT ( 'NONE',  ( -109.9849858529770046, 1384.909542710179949, 311.4561255368179786 ) ) ;
#16719=CARTESIAN_POINT ( 'NONE',  ( -13.60512064039999913, 1388.590188594380152, 217.4599908286989773 ) ) ;
#16728=CARTESIAN_POINT ( 'NONE',  ( -12.53694325390000053, 1380.612673806029761, 215.4769779826689842 ) ) ;
#16735=CARTESIAN_POINT ( 'NONE',  ( -13.72145621289999973, 1390.430903341090016, 208.3849667214680039 ) ) ;
#16745=CARTESIAN_POINT ( 'NONE',  ( -12.28855869350000063, 1378.253616442990051, 210.0769077263690008 ) ) ;
#16757=CARTESIAN_POINT ( 'NONE',  ( -12.66789338582930036, 1383.860718371299981, 218.8636147899300113 ) ) ;
#16770=CARTESIAN_POINT ( 'NONE',  ( -109.7185680580000025, 1384.890266421910155, 297.0862365493590005 ) ) ;
#16781=CARTESIAN_POINT ( 'NONE',  ( -12.11669130219999957, 1391.856317166560075, 209.2336078948329998 ) ) ;
#16782=CARTESIAN_POINT ( 'NONE',  ( -85.14792482515179017, 1385.176708844659743, 288.8829841967900052 ) ) ;
#16808=CARTESIAN_POINT ( 'NONE',  ( -68.53362818316249161, 1379.747368904349969, 280.1371498460779321 ) ) ;
#16810=B_SPLINE_CURVE_WITH_KNOTS ( 'NONE', 5,
 ( #13312, #106836, #14973, #5492, #22258, #56457, #72713, #48620, #90592 ),
 .UNSPECIFIED., .F., .F.,
 ( 6, 3, 6 ),
 ( 0.000000000000000000, 0.4368039669223903743, 1.000000000000000000 ),
 .UNSPECIFIED. ) ;
#16831=ORIENTED_EDGE ( 'NONE', *, *, #65048, .F. ) ;
#16845=CARTESIAN_POINT ( 'NONE',  ( -100.7279122188340068, 1384.876502697709839, 296.3975145639699349 ) ) ;
#16863=CARTESIAN_POINT ( 'NONE',  ( -62.89799739219998997, 1379.732086956869807, 267.9971866538590461 ) ) ;
#16885=CARTESIAN_POINT ( 'NONE',  ( 3.555115653736739510E-15, 1384.926148861439970, 209.1218459572589836 ) ) ;
#16910=CARTESIAN_POINT ( 'NONE',  ( -12.05837087505603833, 1377.636358387990413, 211.6001473997702362 ) ) ;
#16913=CARTESIAN_POINT ( 'NONE',  ( -12.54019733330000008, 1391.397793261360221, 209.7548870936209937 ) ) ;
#16916=CARTESIAN_POINT ( 'NONE',  ( -70.90293112098160577, 1384.660040799420130, 296.0611682970840093 ) ) ;
#16917=CARTESIAN_POINT ( 'NONE',  ( -25.74505365984370187, 1384.960943526260053, 203.5578757433129908 ) ) ;
#16921=CARTESIAN_POINT ( 'NONE',  ( -106.4005663920000018, 1378.913060486199811, 301.5683367484589894 ) ) ;
#16925=CARTESIAN_POINT ( 'NONE',  ( -11.77674179528174569, 1378.208832213107371, 205.4865746833227718 ) ) ;
#16934=CARTESIAN_POINT ( 'NONE',  ( -10.30967637289999850, 1381.062970967459705, 201.9668772049490144 ) ) ;
#16945=CARTESIAN_POINT ( 'NONE',  ( -25.90124155867470179, 1379.608127361219886, 215.5185761863660048 ) ) ;
#16961=PRESENTATION_STYLE_ASSIGNMENT (( #85858 ) ) ;
#16969=EDGE_LOOP ( 'NONE', ( #18221, #87671, #34909, #13237 ) ) ;
#16978=CARTESIAN_POINT ( 'NONE',  ( 8.233576870951500105E-14, 1375.413060387289988, 209.1218459572589836 ) ) ;
#16983=CARTESIAN_POINT ( 'NONE',  ( -105.5730645133519943, 1377.937125738340228, 304.5637690312989889 ) ) ;
#16991=CARTESIAN_POINT ( 'NONE',  ( -96.25814220559999512, 1384.042779414059851, 310.4933417822589377 ) ) ;
#17003=CARTESIAN_POINT ( 'NONE',  ( -62.39649109850000031, 1386.686758807429896, 249.3285297428589899 ) ) ;
#17005=CARTESIAN_POINT ( 'NONE',  ( -62.96821258457789838, 1385.052146392690247, 285.7569334418829499 ) ) ;
#17016=CARTESIAN_POINT ( 'NONE',  ( -108.1487418590059946, 1381.161261816019760, 310.1575172367179789 ) ) ;
#17055=ORIENTED_EDGE ( 'NONE', *, *, #45337, .T. ) ;
#17063=CARTESIAN_POINT ( 'NONE',  ( -35.85007572059999603, 1380.172836988449944, 220.5090016197590046 ) ) ;
#17068=CARTESIAN_POINT ( 'NONE',  ( -113.4000000000000057, 1378.061224848670008, 306.7703178455799957 ) ) ;
#17084=CARTESIAN_POINT ( 'NONE',  ( -8.623386125339999708, 1384.482357225949954, 199.8976969836290039 ) ) ;
#17097=CARTESIAN_POINT ( 'NONE',  ( -5.292751683389999684, 1386.092796132500098, 203.4019327673190105 ) ) ;
#17109=CARTESIAN_POINT ( 'NONE',  ( -28.43185375333949949, 1384.552470293700026, 204.7838833589590024 ) ) ;
#17118=CARTESIAN_POINT ( 'NONE',  ( -68.77278092737650184, 1379.747928288920093, 280.3133413970129482 ) ) ;
#17122=CARTESIAN_POINT ( 'NONE',  ( -68.72163677839999707, 1379.747817063369894, 280.0443424388590188 ) ) ;
#17129=CARTESIAN_POINT ( 'NONE',  ( -3.078458293560000225, 1384.906579013939790, 218.5736861911289850 ) ) ;
#17143=CARTESIAN_POINT ( 'NONE',  ( -8.869114759610731369, 1385.182896069670051, 218.6736307222820130 ) ) ;
#17173=CARTESIAN_POINT ( 'NONE',  ( -5.932239102140000497, 1391.913060387289988, 209.1218459572589836 ) ) ;
#17177=CARTESIAN_POINT ( 'NONE',  ( -72.21359640208430619, 1383.783188034720069, 297.1805363241429632 ) ) ;
#17184=CARTESIAN_POINT ( 'NONE',  ( -47.98273391449999536, 1382.329346158459884, 255.9965235912589492 ) ) ;
#17194=CARTESIAN_POINT ( 'NONE',  ( -108.6438184989999911, 1382.182729019579938, 297.8040021080590236 ) ) ;
#17219=CARTESIAN_POINT ( 'NONE',  ( -108.2870185569999961, 1387.477179604599996, 310.5036998792590452 ) ) ;
#17282=CARTESIAN_POINT ( 'NONE',  ( -12.70027339480000173, 1379.689331990199889, 213.2914259217290009 ) ) ;
#17288=CARTESIAN_POINT ( 'NONE',  ( -12.91227934189999971, 1390.899010879880052, 208.3938681258139809 ) ) ;
#17294=CARTESIAN_POINT ( 'NONE',  ( -8.934489778684168826, 1384.314414410530162, 218.6338716263649928 ) ) ;
#17302=EDGE_CURVE ( 'NONE', #68662, #1545, #2923, .T. ) ;
#17327=FACE_OUTER_BOUND ( 'NONE', #92989, .T. ) ;
#17336=CARTESIAN_POINT ( 'NONE',  ( -11.15738186299999946, 1390.939237837450037, 203.8452286657090156 ) ) ;
#17337=CARTESIAN_POINT ( 'NONE',  ( -83.83445332652270565, 1385.172051411020220, 287.6040778670190434 ) ) ;
#17338=CARTESIAN_POINT ( 'NONE',  ( -11.66658784013729999, 1391.913060387289988, 209.7120188154370339 ) ) ;
#17342=CARTESIAN_POINT ( 'NONE',  ( -107.4477384240240099, 1379.886883745280102, 299.0757736425410371 ) ) ;
#17366=ADVANCED_FACE ( 'NONE', ( #21543 ), #55755, .T. ) ;
#17400=CARTESIAN_POINT ( 'NONE',  ( -10.34436050340000079, 1391.793768386910187, 215.1256036177990154 ) ) ;
#17401=CARTESIAN_POINT ( 'NONE',  ( -105.5483579447400047, 1384.891159839150077, 296.9529443240709838 ) ) ;
#17417=CARTESIAN_POINT ( 'NONE',  ( -37.65558013879999777, 1379.730903953030065, 220.7433301062589805 ) ) ;
#17432=CARTESIAN_POINT ( 'NONE',  ( -8.371636071799999357, 1384.910415699319856, 199.7750054352590041 ) ) ;
#17445=ORIENTED_EDGE ( 'NONE', *, *, #96295, .F. ) ;
#17470=CARTESIAN_POINT ( 'NONE',  ( -75.79932541657819911, 1384.647805970779928, 300.7287927689640128 ) ) ;
#17471=CARTESIAN_POINT ( 'NONE',  ( -26.14076515983080284, 1384.961658909369817, 203.7233559922780159 ) ) ;
#17490=CARTESIAN_POINT ( 'NONE',  ( -8.872398163489998879, 1383.598668384430084, 200.1252679808089852 ) ) ;
#17504=CARTESIAN_POINT ( 'NONE',  ( -65.39490631584679647, 1379.739707105699836, 275.4685780489909916 ) ) ;
#17511=FACE_OUTER_BOUND ( 'NONE', #101726, .T. ) ;
#17513=CARTESIAN_POINT ( 'NONE',  ( -7.561556810379999938, 1385.457612210709840, 219.0574708042989869 ) ) ;
#17538=CARTESIAN_POINT ( 'NONE',  ( -59.08254685325682232, 1379.721614939749088, 259.3076159164612591 ) ) ;
#17539=CARTESIAN_POINT ( 'NONE',  ( -18.96272001720000233, 1380.296266888389937, 209.6316668868479951 ) ) ;
#17554=CARTESIAN_POINT ( 'NONE',  ( -106.4203974090000031, 1384.309678820099862, 311.2870763412590236 ) ) ;
#17567=CARTESIAN_POINT ( 'NONE',  ( -79.40695482969999830, 1386.732498983730011, 283.0119451973590117 ) ) ;
#17569=CARTESIAN_POINT ( 'NONE',  ( -69.45076499915620616, 1385.026108280010021, 294.4474613690360343 ) ) ;
#17578=CARTESIAN_POINT ( 'NONE',  ( -107.1059704325560062, 1382.194773922719833, 310.1619100124009947 ) ) ;
#17593=CARTESIAN_POINT ( 'NONE',  ( -109.5445191200000039, 1385.771176860549986, 297.1603890872589773 ) ) ;
#17607=CARTESIAN_POINT ( 'NONE',  ( -11.58291379525149978, 1384.886121621980010, 218.9039716644460043 ) ) ;
#17652=ORIENTED_EDGE ( 'NONE', *, *, #63323, .T. ) ;
#17669=CARTESIAN_POINT ( 'NONE',  ( -31.92467753469999892, 1384.972130813700005, 206.3032401593790155 ) ) ;
#17670=CARTESIAN_POINT ( 'NONE',  ( -37.44610523480289999, 1384.575341795339909, 210.6318899809130016 ) ) ;
#17680=CARTESIAN_POINT ( 'NONE',  ( -68.57300709150000273, 1379.748249346600005, 279.7358748726589965 ) ) ;
#17685=CARTESIAN_POINT ( 'NONE',  ( -67.03907699609999327, 1384.912355060409936, 292.1878509945590281 ) ) ;
#17687=CARTESIAN_POINT ( 'NONE',  ( -10.02788795287149881, 1385.311267560810165, 218.7355560477120093 ) ) ;
#17707=VECTOR ( 'NONE', #23069, 999.9999999999998863 ) ;
#17734=CARTESIAN_POINT ( 'NONE',  ( -68.62142813640339511, 1383.786590555389921, 293.1919703512040201 ) ) ;
#17735=CARTESIAN_POINT ( 'NONE',  ( -107.7365696369350019, 1379.032352522303881, 299.3254846779751119 ) ) ;
#17742=CARTESIAN_POINT ( 'NONE',  ( -74.89462252569998668, 1381.007359432420117, 297.5740919175589738 ) ) ;
#17752=CARTESIAN_POINT ( 'NONE',  ( -110.0797703000000070, 1384.336996500939904, 296.9599543076590180 ) ) ;
#17775=CARTESIAN_POINT ( 'NONE',  ( -107.8448688559999908, 1387.924802880550033, 310.1598078892590138 ) ) ;
#17796=CARTESIAN_POINT ( 'NONE',  ( -12.23669307423070052, 1377.661331666050273, 207.7794331870949804 ) ) ;
#17816=CARTESIAN_POINT ( 'NONE',  ( -11.63765358216780221, 1391.913060387119913, 208.5693770010209960 ) ) ;
#17827=CARTESIAN_POINT ( 'NONE',  ( -8.744990863649999113, 1385.315572773260101, 218.5566709142290165 ) ) ;
#17838=CARTESIAN_POINT ( 'NONE',  ( -9.292238542100001553, 1381.405190552079830, 217.5286081215490128 ) ) ;
#17845=CARTESIAN_POINT ( 'NONE',  ( -13.27879787639999876, 1390.397743956920067, 206.9666494769190024 ) ) ;
#17871=CARTESIAN_POINT ( 'NONE',  ( -9.506144258141100423, 1383.863471983120007, 218.5502817718870006 ) ) ;
#17887=CARTESIAN_POINT ( 'NONE',  ( -14.28042675339239942, 1390.367274744259930, 209.8448731692960223 ) ) ;
#17896=CARTESIAN_POINT ( 'NONE',  ( -12.09196955530000039, 1391.856377031290094, 209.7328924207210150 ) ) ;
#17897=CARTESIAN_POINT ( 'NONE',  ( -80.63838622464560046, 1385.160061434930185, 283.9401284501640248 ) ) ;
#17899=CARTESIAN_POINT ( 'NONE',  ( -51.76145802239999938, 1379.744278086280019, 243.7243931585590246 ) ) ;
#17910=AXIS2_PLACEMENT_3D ( 'NONE', #85417, #26626, #18764 ) ;
#17923=CARTESIAN_POINT ( 'NONE',  ( -68.77190087506669158, 1379.747925807530009, 280.3125204381590265 ) ) ;
#17938=CARTESIAN_POINT ( 'NONE',  ( -13.72550927608089921, 1379.647794360040052, 208.3261796023589909 ) ) ;
#17950=EDGE_CURVE ( 'NONE', #29914, #91726, #7026, .T. ) ;
#17951=VERTEX_POINT ( 'NONE', #37000 ) ;
#17952=CARTESIAN_POINT ( 'NONE',  ( -14.18795909183540083, 1380.146470109049915, 210.8218107588240002 ) ) ;
#17961=CARTESIAN_POINT ( 'NONE',  ( -94.11669641235350525, 1384.854232109579698, 294.6094501371869683 ) ) ;
#17981=CARTESIAN_POINT ( 'NONE',  ( -14.11459548090000027, 1379.710415317729939, 208.2104247299010069 ) ) ;
#17998=CARTESIAN_POINT ( 'NONE',  ( -9.094910632070000389, 1384.931050598290085, 199.9427863282390092 ) ) ;
#18030=EDGE_LOOP ( 'NONE', ( #98688, #14431, #55245, #47364 ) ) ;
#18039=CARTESIAN_POINT ( 'NONE',  ( -61.29572242790209913, 1384.690799301989955, 283.1176806947750038 ) ) ;
#18040=CARTESIAN_POINT ( 'NONE',  ( -17.14540223173099776, 1384.945687311829943, 201.0017889155920159 ) ) ;
#18042=CARTESIAN_POINT ( 'NONE',  ( -5.238827773017599831, 1374.990239134210015, 214.8178773404370077 ) ) ;
#18046=CARTESIAN_POINT ( 'NONE',  ( -9.094129269030000629, 1384.954944735329946, 199.9429221374590213 ) ) ;
#18059=CARTESIAN_POINT ( 'NONE',  ( -9.393822458599998981, 1383.815214525520105, 200.1452963205690025 ) ) ;
#18073=CARTESIAN_POINT ( 'NONE',  ( -64.26953522495749382, 1379.737737548759924, 273.6740357258199765 ) ) ;
#18079=CARTESIAN_POINT ( 'NONE',  ( -106.5010113160000174, 1379.147773116859980, 307.7477130958589555 ) ) ;
#18135=CARTESIAN_POINT ( 'NONE',  ( -79.49029774420000649, 1385.156174356060092, 282.9512253370589860 ) ) ;
#18149=CARTESIAN_POINT ( 'NONE',  ( -108.3715397873749993, 1382.864756451370113, 310.7319415575520338 ) ) ;
#18163=CARTESIAN_POINT ( 'NONE',  ( -109.6343409440000016, 1386.390526388930084, 297.1907160496590450 ) ) ;
#18177=CARTESIAN_POINT ( 'NONE',  ( -16.85280213986460041, 1384.871734412140086, 219.8759916889669910 ) ) ;
#18199=CARTESIAN_POINT ( 'NONE',  ( -113.4000000000000057, 1378.967725634990074, 306.1169302589129870 ) ) ;
#18203=ORIENTED_EDGE ( 'NONE', *, *, #58995, .T. ) ;
#18221=ORIENTED_EDGE ( 'NONE', *, *, #9979, .T. ) ;
#18230=CARTESIAN_POINT ( 'NONE',  ( -105.9862693054190004, 1378.913060387289988, 302.9553208434759881 ) ) ;
#18235=CARTESIAN_POINT ( 'NONE',  ( -85.86390051840001547, 1385.060281227220003, 289.6783794304589605 ) ) ;
#18236=CARTESIAN_POINT ( 'NONE',  ( -62.23286792741850348, 1384.686997364249919, 248.8895857189220067 ) ) ;
#18247=CARTESIAN_POINT ( 'NONE',  ( -68.43569653030000666, 1379.748342192099926, 279.4446506693590209 ) ) ;
#18255=CARTESIAN_POINT ( 'NONE',  ( -22.68102785909999852, 1384.991329335610089, 222.0421655005590367 ) ) ;
#18257=CARTESIAN_POINT ( 'NONE',  ( -17.87379895800760110, 1385.284389312859957, 220.1513191895170394 ) ) ;
#18302=CARTESIAN_POINT ( 'NONE',  ( -95.87000543284069920, 1383.766626252310061, 310.0354134814519966 ) ) ;
#18311=CARTESIAN_POINT ( 'NONE',  ( -81.27653993580000247, 1383.775959360260003, 304.8043613862590746 ) ) ;
#18321=CARTESIAN_POINT ( 'NONE',  ( -109.8221033779999942, 1384.392514930950028, 297.0589093852589713 ) ) ;
#18389=DIRECTION ( 'NONE',  ( 0.000000000000000000, -1.000000000000000000, 0.000000000000000000 ) ) ;
#18394=CARTESIAN_POINT ( 'NONE',  ( -14.01707770341873527, 1379.589456901253470, 211.9120362016159049 ) ) ;
#18397=CARTESIAN_POINT ( 'NONE',  ( -10.49767883750000053, 1382.256743515189783, 217.7001910593189677 ) ) ;
#18429=CARTESIAN_POINT ( 'NONE',  ( -6.169242136949999455, 1378.878171907740125, 208.5195113185000082 ) ) ;
#18436=CARTESIAN_POINT ( 'NONE',  ( -12.10181609356209975, 1392.233360485750154, 211.6594669569279858 ) ) ;
#18438=EDGE_CURVE ( 'NONE', #73589, #43960, #60330, .T. ) ;
#18445=CARTESIAN_POINT ( 'NONE',  ( -68.28143006493819200, 1385.103599963460056, 262.2692984668489657 ) ) ;
#18447=CARTESIAN_POINT ( 'NONE',  ( -62.03809624990000060, 1379.749343316239901, 266.3689138319589915 ) ) ;
#18473=CARTESIAN_POINT ( 'NONE',  ( -68.75448126042309127, 1379.747879528159956, 280.3343026105569606 ) ) ;
#18487=CARTESIAN_POINT ( 'NONE',  ( -12.54333794360629817, 1378.892795628550175, 208.9638137175840029 ) ) ;
#18508=CARTESIAN_POINT ( 'NONE',  ( -12.50784581649999971, 1391.398398855719961, 210.4070514663689835 ) ) ;
#18510=CARTESIAN_POINT ( 'NONE',  ( -87.98792674194200458, 1384.830566764610012, 291.2189899076259394 ) ) ;
#18528=CARTESIAN_POINT ( 'NONE',  ( -41.90725927229999570, 1379.698394009460117, 226.1262471626590127 ) ) ;
#18563=CARTESIAN_POINT ( 'NONE',  ( -12.29793863238220020, 1378.259112548620124, 208.2596361589930041 ) ) ;
#18583=CARTESIAN_POINT ( 'NONE',  ( -70.16143979324509417, 1384.662073857830137, 295.2445469226630053 ) ) ;
#18584=CARTESIAN_POINT ( 'NONE',  ( -23.72885132301209765, 1384.957336300120005, 202.7962431987409957 ) ) ;
#18601=CARTESIAN_POINT ( 'NONE',  ( -8.179930635319999865, 1384.351711335470100, 199.6861503408189833 ) ) ;
#18614=CARTESIAN_POINT ( 'NONE',  ( -63.27222210238460320, 1379.733933836859933, 271.8034403823299954 ) ) ;
#18623=CARTESIAN_POINT ( 'NONE',  ( -7.552662639750000295, 1385.340273189239952, 219.0680905273789847 ) ) ;
#18652=CARTESIAN_POINT ( 'NONE',  ( -14.17772861730700207, 1379.591530685439920, 207.8208986668599891 ) ) ;
#18671=B_SPLINE_CURVE_WITH_KNOTS ( 'NONE', 3,
 ( #27412, #78379, #87332, #10628, #95180, #10062, #70011, #11190, #60490, #96282, #44235, #94611, #8954, #43127, #69451, #86216, #26300, #104125, #53765, #95728, #1687, #18992 ),
 .UNSPECIFIED., .F., .F.,
 ( 4, 3, 3, 3, 3, 3, 3, 4 ),
 ( -136.9024435287539916, -136.6634106196869993, -136.4076183642550006, -136.1480203043660140, -135.8861880622630167, -135.6207110178370101, -135.3532902909820166, -135.0843706930000110 ),
 .UNSPECIFIED. ) ;
#18681=CARTESIAN_POINT ( 'NONE',  ( -87.30316128990000379, 1388.086780051900178, 306.8656371684590454 ) ) ;
#18682=ORIENTED_EDGE ( 'NONE', *, *, #108224, .F. ) ;
#18693=CARTESIAN_POINT ( 'NONE',  ( -109.1074149406630056, 1382.912272179509955, 310.9584811440479939 ) ) ;
#18714=ADVANCED_FACE ( 'NONE', ( #82476 ), #1450, .F. ) ;
#18721=CARTESIAN_POINT ( 'NONE',  ( -20.98450557191650034, 1384.859229475929851, 221.3795081009360217 ) ) ;
#18745=CARTESIAN_POINT ( 'NONE',  ( -101.7780583737760054, 1379.485289778789820, 304.0159838458559989 ) ) ;
#18764=DIRECTION ( 'NONE',  ( -0.9997613315435491810, 0.000000000000000000, 0.02184673774890954004 ) ) ;
#18766=CARTESIAN_POINT ( 'NONE',  ( -113.4000000000000057, 1384.926148861439970, 304.2218459572590064 ) ) ;
#18768=ORIENTED_EDGE ( 'NONE', *, *, #35246, .F. ) ;
#18769=ORIENTED_EDGE ( 'NONE', *, *, #76182, .T. ) ;
#18778=CARTESIAN_POINT ( 'NONE',  ( -94.55573068399999670, 1374.531630663889928, 302.1084921616590009 ) ) ;
#18779=CARTESIAN_POINT ( 'NONE',  ( -106.1739094701860040, 1378.913060387289988, 302.4879143702450506 ) ) ;
#18785=CARTESIAN_POINT ( 'NONE',  ( -62.89508772654340873, 1384.691239647969724, 250.3595330377160337 ) ) ;
#18798=CARTESIAN_POINT ( 'NONE',  ( -66.95646680580000520, 1379.743567625210062, 276.4036447723590300 ) ) ;
#18808=CARTESIAN_POINT ( 'NONE',  ( -59.23393169420000248, 1385.069165163979960, 279.9259648821590645 ) ) ;
#18810=CARTESIAN_POINT ( 'NONE',  ( -105.6563836332091597, 1378.913058981198219, 304.0447272458403631 ) ) ;
#18851=CARTESIAN_POINT ( 'NONE',  ( -100.5687700116990015, 1383.763643007270048, 310.7088986134360198 ) ) ;
#18859=CARTESIAN_POINT ( 'NONE',  ( -76.21403627649999635, 1383.779720587099746, 301.0850818666589817 ) ) ;
#18869=CARTESIAN_POINT ( 'NONE',  ( -108.2394657659999950, 1382.219629552339939, 297.9605983755590159 ) ) ;
#18888=CARTESIAN_POINT ( 'NONE',  ( -110.0634901748029932, 1384.899971912700039, 296.9512050915229793 ) ) ;
#18899=DIRECTION ( 'NONE',  ( 1.000000000000000000, 0.000000000000000000, 0.000000000000000000 ) ) ;
#18945=CARTESIAN_POINT ( 'NONE',  ( -13.85129689699811451, 1390.139984326732701, 212.7740231941627655 ) ) ;
#18956=ORIENTED_EDGE ( 'NONE', *, *, #75470, .F. ) ;
#18966=CARTESIAN_POINT ( 'NONE',  ( -12.31816045095820122, 1378.322797730630100, 209.5997611854560034 ) ) ;
#18978=CARTESIAN_POINT ( 'NONE',  ( -33.18021480408270207, 1383.837964353870120, 231.4654556182339888 ) ) ;
#18986=CARTESIAN_POINT ( 'NONE',  ( -3.078458355069999985, 1384.494027187519805, 199.6978503428690033 ) ) ;
#18992=CARTESIAN_POINT ( 'NONE',  ( -14.53473304376390018, 1379.710786975620067, 208.2794084638009906 ) ) ;
#18999=CARTESIAN_POINT ( 'NONE',  ( -12.32169104970000006, 1391.303891397440111, 206.9552536725390155 ) ) ;
#19000=CARTESIAN_POINT ( 'NONE',  ( -89.80898548959270045, 1385.192144560830002, 292.4574326567000639 ) ) ;
#19002=CARTESIAN_POINT ( 'NONE',  ( -66.55629426049999608, 1379.749035308849898, 275.7365325667589673 ) ) ;
#19039=CARTESIAN_POINT ( 'NONE',  ( -12.79475420062619939, 1379.177177335730221, 208.7218844242719911 ) ) ;
#19078=CARTESIAN_POINT ( 'NONE',  ( -32.57298063980000080, 1379.681802635260055, 216.0596865545890068 ) ) ;
#19082=CARTESIAN_POINT ( 'NONE',  ( -68.47067290995560995, 1379.747730938292307, 280.0399411559841951 ) ) ;
#19091=CARTESIAN_POINT ( 'NONE',  ( -7.965680540240001051, 1384.926148861439970, 199.4891222871690104 ) ) ;
#19114=CARTESIAN_POINT ( 'NONE',  ( -12.31752474539220010, 1377.944612774040024, 209.1221336184720201 ) ) ;
#19133=CARTESIAN_POINT ( 'NONE',  ( -72.07271172023830275, 1384.656943536320114, 297.2850582096680228 ) ) ;
#19134=CARTESIAN_POINT ( 'NONE',  ( -44.54400286966450295, 1385.001782504770063, 217.7620875069719943 ) ) ;
#19140=CARTESIAN_POINT ( 'NONE',  ( -8.604576571519999106, 1384.925122429579915, 199.8686409562490098 ) ) ;
#19146=CARTESIAN_POINT ( 'NONE',  ( -106.9772147180469943, 1391.913060387289988, 306.6383769938329920 ) ) ;
#19150=CARTESIAN_POINT ( 'NONE',  ( -8.395462917950000659, 1384.396045361419965, 199.8129348554689955 ) ) ;
#19163=CARTESIAN_POINT ( 'NONE',  ( -62.71435643260001314, 1379.746901600850151, 270.6043089134589650 ) ) ;
#19171=DIRECTION ( 'NONE',  ( -0.9991156138703695122, 0.000000000000000000, 0.04204747460234692369 ) ) ;
#19197=CARTESIAN_POINT ( 'NONE',  ( -41.28229943905566302, 1379.658502791898627, 225.0653720194143546 ) ) ;
#19208=CARTESIAN_POINT ( 'NONE',  ( -29.09816620510556362, 1379.626347181600977, 217.7851320636372918 ) ) ;
#19226=CARTESIAN_POINT ( 'NONE',  ( -81.17886098919998972, 1384.990453609069846, 304.9592558327589700 ) ) ;
#19238=CARTESIAN_POINT ( 'NONE',  ( -104.3125648498219817, 1379.920782886319785, 305.5271631452329757 ) ) ;
#19247=EDGE_CURVE ( 'NONE', #46346, #74400, #37446, .T. ) ;
#19271=CARTESIAN_POINT ( 'NONE',  ( -15.94115646620460147, 1384.874344242760117, 219.6433026291970236 ) ) ;
#19289=ADVANCED_FACE ( 'NONE', ( #7688 ), #74646, .T. ) ;
#19292=CARTESIAN_POINT ( 'NONE',  ( -109.9872068205719984, 1384.854720727420045, 311.4556833561759390 ) ) ;
#19320=ORIENTED_EDGE ( 'NONE', *, *, #100767, .T. ) ;
#19331=CARTESIAN_POINT ( 'NONE',  ( -69.36674278830000162, 1379.746858117810007, 280.1513224085589968 ) ) ;
#19334=CARTESIAN_POINT ( 'NONE',  ( -105.7960290519230000, 1378.913060387289988, 303.9610383217989806 ) ) ;
#19337=CARTESIAN_POINT ( 'NONE',  ( -92.78435512849998190, 1384.849527344140142, 294.1459074807589786 ) ) ;
#19345=CARTESIAN_POINT ( 'NONE',  ( -3.078458294050000266, 1383.868666969369770, 218.4015365393190109 ) ) ;
#19351=CARTESIAN_POINT ( 'NONE',  ( -66.36498982899999532, 1379.745690266980091, 275.3119164116589559 ) ) ;
#19359=CARTESIAN_POINT ( 'NONE',  ( -47.37130750840000104, 1384.881166745699829, 256.2794477600589858 ) ) ;
#19361=CARTESIAN_POINT ( 'NONE',  ( -10.35521326297049960, 1385.310235430599960, 218.7605991785599997 ) ) ;
#19411=CARTESIAN_POINT ( 'NONE',  ( -94.12119808786221142, 1383.767725327359813, 309.6675098620430049 ) ) ;
#19413=CARTESIAN_POINT ( 'NONE',  ( -108.7912213487909980, 1383.917108116560030, 311.1258975414110068 ) ) ;
#19419=CARTESIAN_POINT ( 'NONE',  ( -85.29011547940000071, 1381.870680097800005, 290.3579090523590480 ) ) ;
#19442=ORIENTED_EDGE ( 'NONE', *, *, #49792, .T. ) ;
#19495=CARTESIAN_POINT ( 'NONE',  ( -11.55918612708340021, 1391.913060387249971, 207.9911993583930325 ) ) ;
#19505=CARTESIAN_POINT ( 'NONE',  ( -27.45731751820000355, 1390.955273319920252, 213.9131165264389836 ) ) ;
#19511=CARTESIAN_POINT ( 'NONE',  ( -14.02252553536541235, 1379.587897852161632, 211.9004556758163460 ) ) ;
#19513=AXIS2_PLACEMENT_3D ( 'NONE', #100065, #32850, #83815 ) ;
#19514=CARTESIAN_POINT ( 'NONE',  ( -11.18262514070000080, 1381.429409390050068, 216.8219888905990160 ) ) ;
#19521=DIRECTION ( 'NONE',  ( -1.836970198721029688E-16, -1.000000000000000000, 0.000000000000000000 ) ) ;
#19526=CARTESIAN_POINT ( 'NONE',  ( -12.31337600513549901, 1378.372828873670187, 209.7376539469879901 ) ) ;
#19544=CARTESIAN_POINT ( 'NONE',  ( -20.48566081668520056, 1383.853069179059958, 220.9684220193649935 ) ) ;
#19553=CARTESIAN_POINT ( 'NONE',  ( -3.078458325710000221, 1378.867273990040076, 208.5251302500439863 ) ) ;
#19567=CARTESIAN_POINT ( 'NONE',  ( -95.92464888116629140, 1385.210119995399964, 295.2644287896150104 ) ) ;
#19571=CARTESIAN_POINT ( 'NONE',  ( -54.25698729759999850, 1379.746222734200046, 249.0120014888590276 ) ) ;
#19595=CARTESIAN_POINT ( 'NONE',  ( -109.1655177890000061, 1384.872414444939977, 297.1329087538589420 ) ) ;
#19643=CARTESIAN_POINT ( 'NONE',  ( -107.7923298369999969, 1386.973993580999831, 297.6574877858589616 ) ) ;
#19646=CARTESIAN_POINT ( 'NONE',  ( -37.91547825339999633, 1379.647889607849947, 220.5156237355589894 ) ) ;
#19650=CARTESIAN_POINT ( 'NONE',  ( -19.29595629980909877, 1379.713387097429404, 212.5268654157613355 ) ) ;
#19657=CARTESIAN_POINT ( 'NONE',  ( -55.97777492769100149, 1385.087189547780099, 273.6896789270770114 ) ) ;
#19684=CARTESIAN_POINT ( 'NONE',  ( -14.31803753242949817, 1379.584910753419990, 207.9694682050350139 ) ) ;
#19706=CARTESIAN_POINT ( 'NONE',  ( -89.21435300837349303, 1384.620659748430171, 308.4344151408140533 ) ) ;
#19707=CARTESIAN_POINT ( 'NONE',  ( -40.27720933358730093, 1384.990567941889822, 213.1516827062340269 ) ) ;
#19713=CARTESIAN_POINT ( 'NONE',  ( -8.156587067910001210, 1384.920246153470089, 199.6468409925089986 ) ) ;
#19726=CARTESIAN_POINT ( 'NONE',  ( -11.39873841100000007, 1380.703654181990032, 203.1461614638990056 ) ) ;
#19739=CARTESIAN_POINT ( 'NONE',  ( -65.79241599563980003, 1379.740566815069997, 276.1610046520289643 ) ) ;
#19741=VERTEX_POINT ( 'NONE', #108733 ) ;
#19744=CARTESIAN_POINT ( 'NONE',  ( -105.5263324250000068, 1378.950045411100064, 305.1391035067590565 ) ) ;
#19750=CARTESIAN_POINT ( 'NONE',  ( -106.1387134729239961, 1378.913060388289978, 305.7024349280350179 ) ) ;
#19767=CARTESIAN_POINT ( 'NONE',  ( -8.297791668369999485, 1384.930381111709949, 218.7035399147090118 ) ) ;
#19777=TOROIDAL_SURFACE ( 'NONE', #9066, 11.99982860380000105, 0.5000000000000000000 ) ;
#19782=CARTESIAN_POINT ( 'NONE',  ( -27.47436269071217296, 1379.622196554404354, 216.6943055741242006 ) ) ;
#19799=CARTESIAN_POINT ( 'NONE',  ( -80.90466521880000528, 1390.617052934750063, 295.5380644611589673 ) ) ;
#19810=CARTESIAN_POINT ( 'NONE',  ( -105.2550079177960072, 1380.603825893849944, 307.9159414798160697 ) ) ;
#19836=CARTESIAN_POINT ( 'NONE',  ( -12.16775715655800028, 1384.884604198070065, 218.9723175489479843 ) ) ;
#19860=CARTESIAN_POINT ( 'NONE',  ( -62.02946302165940295, 1379.821285026140004, 270.5012637983109585 ) ) ;
#19869=CARTESIAN_POINT ( 'NONE',  ( -8.835564857580001430, 1383.775455445409989, 218.4808771233589937 ) ) ;
#19888=ORIENTED_EDGE ( 'NONE', *, *, #42848, .F. ) ;
#19890=CARTESIAN_POINT ( 'NONE',  ( -85.19634273949999681, 1374.907833766890008, 296.7812697200590151 ) ) ;
#19906=CARTESIAN_POINT ( 'NONE',  ( -19.17386968219999943, 1384.864972699589771, 220.5237385319589976 ) ) ;
#19911=CARTESIAN_POINT ( 'NONE',  ( -65.90645751559999610, 1379.740571517399758, 274.2408093113589871 ) ) ;
#19920=CARTESIAN_POINT ( 'NONE',  ( -62.07136965400000150, 1384.687060561920134, 284.7656473558590164 ) ) ;
#19922=CARTESIAN_POINT ( 'NONE',  ( -25.89380455557000005, 1385.251986020480217, 224.3320981585399920 ) ) ;
#19949=DIRECTION ( 'NONE',  ( 0.9991156149436395406, 0.000000000000000000, -0.04204744909971582650 ) ) ;
#19953=CARTESIAN_POINT ( 'NONE',  ( -105.5745406720000119, 1391.578499750080027, 304.2150149938590289 ) ) ;
#19972=CARTESIAN_POINT ( 'NONE',  ( -84.55035757104050731, 1383.773842207470125, 306.2764245462699932 ) ) ;
#19978=CARTESIAN_POINT ( 'NONE',  ( -77.39008541779999462, 1380.628426168399983, 284.5123695392589980 ) ) ;
#20027=EDGE_CURVE ( 'NONE', #82812, #6492, #62185, .T. ) ;
#20032=ORIENTED_EDGE ( 'NONE', *, *, #1601, .T. ) ;
#20045=EDGE_CURVE ( 'NONE', #108404, #6840, #110434, .T. ) ;
#20060=CARTESIAN_POINT ( 'NONE',  ( -34.95273570850000056, 1389.711644948749836, 227.7285918695590112 ) ) ;
#20061=CARTESIAN_POINT ( 'NONE',  ( -10.82432768028174053, 1387.838219566829594, 217.4113394113601316 ) ) ;
#20065=CARTESIAN_POINT ( 'NONE',  ( -14.05089909369253753, 1379.587328361107211, 211.8228618032813699 ) ) ;
#20099=CARTESIAN_POINT ( 'NONE',  ( -26.82051671160990125, 1383.845951110550004, 224.8659914338689703 ) ) ;
#20107=CARTESIAN_POINT ( 'NONE',  ( -7.985077194497058883, 1385.602515846550887, 199.5277730303256192 ) ) ;
#20114=CARTESIAN_POINT ( 'NONE',  ( -13.02325698038220025, 1389.786154039980147, 214.1047924551970141 ) ) ;
#20124=CARTESIAN_POINT ( 'NONE',  ( -93.46554775850030694, 1385.203179652859944, 294.3505717766860244 ) ) ;
#20125=CARTESIAN_POINT ( 'NONE',  ( -10.21500170628049986, 1391.913060387289988, 214.1061961160360170 ) ) ;
#20126=CARTESIAN_POINT ( 'NONE',  ( -47.55875411400000274, 1379.740588162619815, 235.3895649973590025 ) ) ;
#20132=EDGE_CURVE ( 'NONE', #60994, #23316, #67535, .T. ) ;
#20145=CARTESIAN_POINT ( 'NONE',  ( -103.6765714240000023, 1379.937512265609939, 302.8207899414589974 ) ) ;
#20176=CARTESIAN_POINT ( 'NONE',  ( -108.4621596517139892, 1384.899542035220065, 297.1088480531129790 ) ) ;
#20204=CARTESIAN_POINT ( 'NONE',  ( -70.52515152282619226, 1385.022333344260005, 295.6573805310360399 ) ) ;
#20229=CARTESIAN_POINT ( 'NONE',  ( -12.57424790809989901, 1378.934406982339851, 208.2958865634099936 ) ) ;
#20236=CARTESIAN_POINT ( 'NONE',  ( -7.543411004532610598, 1384.832500331219762, 219.0864943133630049 ) ) ;
#20250=CARTESIAN_POINT ( 'NONE',  ( -106.4523221262569876, 1384.588530624839905, 311.2244654649010158 ) ) ;
#20252=CARTESIAN_POINT ( 'NONE',  ( -35.56235328268290630, 1384.979870847169877, 209.1200667756079952 ) ) ;
#20253=CARTESIAN_POINT ( 'NONE',  ( -5.186175634954670599, 1375.029200368459897, 214.7946987418769993 ) ) ;
#20269=CARTESIAN_POINT ( 'NONE',  ( -11.97041545340000113, 1377.998423774769890, 206.0180012850990181 ) ) ;
#20280=CARTESIAN_POINT ( 'NONE',  ( -68.38416025601300419, 1379.747023923529923, 279.9629332694450454 ) ) ;
#20291=B_SPLINE_CURVE_WITH_KNOTS ( 'NONE', 3,
 ( #35974, #37067, #71263, #105384, #28672, #62878, #96989, #20253, #18042, #46044, #80176, #3492, #37620, #94764, #40361, #29222 ),
 .UNSPECIFIED., .F., .F.,
 ( 4, 2, 2, 2, 2, 2, 2, 4 ),
 ( 0.08222331860531204017, 0.08289724164938169770, 0.1008996809443339915, 0.1197691111161940103, 0.1404166416624439973, 0.1523778974832539768, 0.1644143184452410145, 0.1647592702822719968 ),
 .UNSPECIFIED. ) ;
#20312=CARTESIAN_POINT ( 'NONE',  ( -12.31997106290000055, 1378.116150593050179, 209.3647868251559885 ) ) ;
#20313=CARTESIAN_POINT ( 'NONE',  ( -68.21293751808869388, 1379.746846629274842, 278.8708533149582536 ) ) ;
#20326=CARTESIAN_POINT ( 'NONE',  ( -42.58097080400749235, 1379.666281498085482, 232.7225854015026698 ) ) ;
#20336=FACE_OUTER_BOUND ( 'NONE', #47403, .T. ) ;
#20345=CARTESIAN_POINT ( 'NONE',  ( -106.7016412910000014, 1389.434639682969873, 300.0422109230589740 ) ) ;
#20356=CARTESIAN_POINT ( 'NONE',  ( -106.0127463409999962, 1379.506663669829777, 307.3641268108590339 ) ) ;
#20379=CARTESIAN_POINT ( 'NONE',  ( -23.85220579467060276, 1384.849935670340074, 222.9428685578329805 ) ) ;
#20398=CARTESIAN_POINT ( 'NONE',  ( -109.9764103964939892, 1384.522409963689825, 311.4409506053760310 ) ) ;
#20403=CARTESIAN_POINT ( 'NONE',  ( -66.65550921930001493, 1376.456288702509937, 281.7771486387589448 ) ) ;
#20412=CARTESIAN_POINT ( 'NONE',  ( -8.489398380670001742, 1383.783001120280005, 218.5304454457089776 ) ) ;
#20420=DIRECTION ( 'NONE',  ( 1.000000000000000000, 0.000000000000000000, 0.000000000000000000 ) ) ;
#20426=ORIENTED_EDGE ( 'NONE', *, *, #81578, .F. ) ;
#20434=CARTESIAN_POINT ( 'NONE',  ( -85.19634273949999681, 1379.292758746510117, 296.7812697164590077 ) ) ;
#20440=CARTESIAN_POINT ( 'NONE',  ( -103.7379217180000097, 1384.886069803950022, 296.9203887490589864 ) ) ;
#20447=CARTESIAN_POINT ( 'NONE',  ( -8.743385264969999682, 1384.893486076239924, 218.5827849380889916 ) ) ;
#20451=CARTESIAN_POINT ( 'NONE',  ( -66.97296676889999389, 1379.743459854440061, 276.3954181864590396 ) ) ;
#20462=CARTESIAN_POINT ( 'NONE',  ( -37.65727875451359807, 1385.195046747119932, 238.1789081722270112 ) ) ;
#20465=CARTESIAN_POINT ( 'NONE',  ( -106.3976693117229928, 1390.939243848519936, 307.7527733253859878 ) ) ;
#20469=CARTESIAN_POINT ( 'NONE',  ( -7.960775697985232213, 1384.702683515537956, 199.4917424227981826 ) ) ;
#20476=EDGE_LOOP ( 'NONE', ( #99427, #23857, #20032, #54371 ) ) ;
#20492=CARTESIAN_POINT ( 'NONE',  ( -104.4989196679999992, 1379.706513807679812, 303.6605283612590256 ) ) ;
#20506=CARTESIAN_POINT ( 'NONE',  ( -76.37423058801520881, 1383.779709834140021, 300.9739160671820173 ) ) ;
#20508=CARTESIAN_POINT ( 'NONE',  ( -109.0618172498179916, 1383.544782690639977, 311.0389996180940102 ) ) ;
#20512=CARTESIAN_POINT ( 'NONE',  ( -98.86909676750001097, 1384.870948519250078, 296.2469157437590184 ) ) ;
#20618=CARTESIAN_POINT ( 'NONE',  ( -109.8982923870000121, 1385.096845541700077, 297.0319097604589729 ) ) ;
#20629=CARTESIAN_POINT ( 'NONE',  ( -20.76923605841339793, 1383.852768131139783, 221.0916664262549887 ) ) ;
#20630=CIRCLE ( 'NONE', #29599, 2.000034594847158065 ) ;
#20640=CARTESIAN_POINT ( 'NONE',  ( -8.125464938096873979, 1386.278383885165113, 199.6698962121421914 ) ) ;
#20647=CARTESIAN_POINT ( 'NONE',  ( -9.882261837502390733, 1388.398873433800190, 217.1410497004710010 ) ) ;
#20656=CARTESIAN_POINT ( 'NONE',  ( -107.2083758124640127, 1385.238133497090075, 297.0681113654679848 ) ) ;
#20662=ORIENTED_EDGE ( 'NONE', *, *, #4271, .F. ) ;
#20679=CARTESIAN_POINT ( 'NONE',  ( -8.860265397230000062, 1385.060179297459854, 218.6816725719889973 ) ) ;
#20710=ADVANCED_FACE ( 'NONE', ( #27282, #53622 ), #79907, .T. ) ;
#20733=CARTESIAN_POINT ( 'NONE',  ( -109.7725577738988108, 1383.360694053928455, 297.1371496055471653 ) ) ;
#20738=CARTESIAN_POINT ( 'NONE',  ( -68.34593600991827600, 1379.747695174417913, 279.8829065417061202 ) ) ;
#20745=CARTESIAN_POINT ( 'NONE',  ( -105.8331820287869931, 1384.932354072029966, 311.2232221701380581 ) ) ;
#20747=CARTESIAN_POINT ( 'NONE',  ( -8.268835750490000081, 1384.932997505379944, 199.7028512843090198 ) ) ;
#20779=CARTESIAN_POINT ( 'NONE',  ( -7.597325770185070049, 1384.051822739160116, 219.0196936294289856 ) ) ;
#20788=EDGE_CURVE ( 'NONE', #96593, #81708, #70915, .T. ) ;
#20794=CARTESIAN_POINT ( 'NONE',  ( -83.70238417473080972, 1384.631100110490024, 306.0393046053840180 ) ) ;
#20795=CARTESIAN_POINT ( 'NONE',  ( -35.18605615840250067, 1384.979076970040069, 208.8412567272559954 ) ) ;
#20817=CARTESIAN_POINT ( 'NONE',  ( -9.448886036450000248, 1383.288095429739997, 218.3547579606889997 ) ) ;
#20831=CARTESIAN_POINT ( 'NONE',  ( -67.58960521306219960, 1379.745587075000003, 278.8661543758199741 ) ) ;
#20837=CARTESIAN_POINT ( 'NONE',  ( -109.4845004149999994, 1384.937458541380011, 311.2840473662590171 ) ) ;
#20847=DIRECTION ( 'NONE',  ( 0.8090169943747140824, -7.703825410061002683E-33, 0.5877852522927943246 ) ) ;
#20854=EDGE_LOOP ( 'NONE', ( #94608, #17055, #37669, #80401 ) ) ;
#20862=CARTESIAN_POINT ( 'NONE',  ( -67.56224301914092223, 1379.745465240531303, 277.5421263419358411 ) ) ;
#20866=CARTESIAN_POINT ( 'NONE',  ( -51.61765082585089459, 1384.627073787560221, 227.8738222896710113 ) ) ;
#20873=DIRECTION ( 'NONE',  ( 1.836970198721029688E-16, 1.000000000000000000, -1.262177448353620010E-31 ) ) ;
#20884=CARTESIAN_POINT ( 'NONE',  ( -104.1336782687082234, 1379.826409842592739, 304.0106197004701585 ) ) ;
#20892=CARTESIAN_POINT ( 'NONE',  ( -106.7752590979999923, 1385.237353006989906, 297.1314966531590471 ) ) ;
#20899=DIRECTION ( 'NONE',  ( -0.009310542140203791062, -0.9999463363072063071, 0.004542940771242790637 ) ) ;
#20903=CARTESIAN_POINT ( 'NONE',  ( -12.26982153759260008, 1378.706398924530049, 210.4710096042489909 ) ) ;
#20904=CARTESIAN_POINT ( 'NONE',  ( -106.5015102169999892, 1378.995521017789997, 308.0072629902589938 ) ) ;
#20928=CARTESIAN_POINT ( 'NONE',  ( -28.73531012334500190, 1384.833055677890115, 226.7915508562620062 ) ) ;
#20945=CARTESIAN_POINT ( 'NONE',  ( -12.31045119098629925, 1378.376187953739873, 209.7947064970520046 ) ) ;
#20952=CARTESIAN_POINT ( 'NONE',  ( -42.70274084799289938, 1379.638451954410129, 233.1566849246620166 ) ) ;
#20955=CARTESIAN_POINT ( 'NONE',  ( -19.25299971689319989, 1379.621289133459868, 212.6578715478160007 ) ) ;
#20962=CARTESIAN_POINT ( 'NONE',  ( -8.784226513880000198, 1383.880421208059943, 218.5159863009489811 ) ) ;
#20982=FACE_OUTER_BOUND ( 'NONE', #71323, .T. ) ;
#20985=CARTESIAN_POINT ( 'NONE',  ( -35.85007572059999603, 1375.172836988449944, 220.5090016197590046 ) ) ;
#20986=B_SPLINE_CURVE_WITH_KNOTS ( 'NONE', 3,
 ( #92886, #25671, #109699, #59864, #16702, #68827, #76101, #102389, #26229, #85033 ),
 .UNSPECIFIED., .F., .F.,
 ( 4, 3, 3, 4 ),
 ( 0.9035847615492319518, 0.9657249562039529334, 1.011896175524879871, 1.040557828610000124 ),
 .UNSPECIFIED. ) ;
#21001=CARTESIAN_POINT ( 'NONE',  ( -66.57398076899998784, 1379.745927938969999, 275.7277585373589659 ) ) ;
#21011=CARTESIAN_POINT ( 'NONE',  ( -89.65053622680001411, 1384.736506983960226, 308.7475415573589999 ) ) ;
#21013=CARTESIAN_POINT ( 'NONE',  ( -30.62646649957819989, 1385.230650423509815, 228.7000830702139922 ) ) ;
#21016=CARTESIAN_POINT ( 'NONE',  ( -106.7386147527374902, 1391.793769404327804, 307.5809084578692705 ) ) ;
#21022=CARTESIAN_POINT ( 'NONE',  ( -113.3410085367727334, 1379.913060387289988, 301.7225420527167898 ) ) ;
#21027=ORIENTED_EDGE ( 'NONE', *, *, #8891, .T. ) ;
#21037=CARTESIAN_POINT ( 'NONE',  ( -105.0196130309999916, 1390.463866858269739, 304.1900705858589617 ) ) ;
#21058=CARTESIAN_POINT ( 'NONE',  ( -109.1218884720000091, 1383.638097810560112, 311.0730448896949838 ) ) ;
#21067=CARTESIAN_POINT ( 'NONE',  ( -110.0636332773229924, 1384.926148836659877, 296.9511394268049571 ) ) ;
#21077=FACE_OUTER_BOUND ( 'NONE', #35262, .T. ) ;
#21081=CARTESIAN_POINT ( 'NONE',  ( -108.0661742336610018, 1378.913060387289988, 308.5496305239910271 ) ) ;
#21114=ORIENTED_EDGE ( 'NONE', *, *, #36740, .T. ) ;
#21138=CARTESIAN_POINT ( 'NONE',  ( -9.109477210328888575, 1384.590310583010250, 199.9607628076590231 ) ) ;
#21153=CIRCLE ( 'NONE', #98072, 2.000012941106792841 ) ;
#21159=CARTESIAN_POINT ( 'NONE',  ( -12.31544236599309983, 1378.361828460810102, 209.6885106622719945 ) ) ;
#21172=CARTESIAN_POINT ( 'NONE',  ( -19.11991078017920032, 1383.854501207500107, 220.4169213401859793 ) ) ;
#21179=CARTESIAN_POINT ( 'NONE',  ( -24.66946762459999931, 1380.257393238360009, 206.6025861486290012 ) ) ;
#21186=CARTESIAN_POINT ( 'NONE',  ( -9.095095392940001133, 1388.475365584439942, 217.6269457225290012 ) ) ;
#21194=CARTESIAN_POINT ( 'NONE',  ( -91.93155929093219925, 1385.198662290420089, 293.6444189235990052 ) ) ;
#21195=DIRECTION ( 'NONE',  ( -1.000000000000000000, 0.000000000000000000, 0.000000000000000000 ) ) ;
#21207=CARTESIAN_POINT ( 'NONE',  ( -109.2202009529999884, 1384.950645967480114, 311.2644681782590510 ) ) ;
#21217=DIRECTION ( 'NONE',  ( 1.000000000000000000, 0.000000000000000000, 0.000000000000000000 ) ) ;
#21269=CARTESIAN_POINT ( 'NONE',  ( -108.3767226235554375, 1381.034261239543866, 298.1262863712069020 ) ) ;
#21274=CARTESIAN_POINT ( 'NONE',  ( -106.4020727818770098, 1391.913060387289988, 304.2008118092670088 ) ) ;
#21282=CARTESIAN_POINT ( 'NONE',  ( -91.22333267815579916, 1384.966695060079928, 309.0954049842840163 ) ) ;
#21284=CARTESIAN_POINT ( 'NONE',  ( -9.398774730970000491, 1388.838992215879898, 201.0120684272889946 ) ) ;
#21333=CARTESIAN_POINT ( 'NONE',  ( -101.9108661632280075, 1384.597254715800091, 311.0043636481769909 ) ) ;
#21334=CARTESIAN_POINT ( 'NONE',  ( -36.32278535918399598, 1384.981498583400025, 209.7013335389069937 ) ) ;
#21341=CARTESIAN_POINT ( 'NONE',  ( -109.6573945330000157, 1384.913341287360026, 311.3230419672590301 ) ) ;
#21353=CARTESIAN_POINT ( 'NONE',  ( -12.42424857989999865, 1378.957147359669989, 207.0567700494690087 ) ) ;
#21365=CARTESIAN_POINT ( 'NONE',  ( -67.68653639069999883, 1379.747580689210054, 278.9655481578590184 ) ) ;
#21367=ORIENTED_EDGE ( 'NONE', *, *, #86710, .F. ) ;
#21384=CARTESIAN_POINT ( 'NONE',  ( 3.552713678799999608E-15, 1384.913060387289988, 209.1218459572589836 ) ) ;
#21393=CARTESIAN_POINT ( 'NONE',  ( -14.09820228469869896, 1379.801286730300035, 211.4211468150479902 ) ) ;
#21397=CARTESIAN_POINT ( 'NONE',  ( -68.30823798306452943, 1379.747042357273358, 279.0703650132669509 ) ) ;
#21402=CARTESIAN_POINT ( 'NONE',  ( -61.12661706479850210, 1384.679990717839928, 246.4532168033390178 ) ) ;
#21421=CIRCLE ( 'NONE', #28555, 2.000048411567817652 ) ;
#21470=CARTESIAN_POINT ( 'NONE',  ( -25.87963768509780138, 1384.843092929030036, 224.3457638931510019 ) ) ;
#21472=CARTESIAN_POINT ( 'NONE',  ( -105.9306909619999999, 1379.241374661100053, 301.2498419558590399 ) ) ;
#21493=CARTESIAN_POINT ( 'NONE',  ( -66.50370960850830215, 1378.395022579190027, 281.8681772372950149 ) ) ;
#21504=CARTESIAN_POINT ( 'NONE',  ( -8.343937223730000241, 1384.261598685969830, 218.6501499107789925 ) ) ;
#21526=CARTESIAN_POINT ( 'NONE',  ( -12.58290190409640097, 1379.610136253339988, 209.8104529657169905 ) ) ;
#21530=CARTESIAN_POINT ( 'NONE',  ( -59.84652512769999788, 1378.966454954579831, 258.3077303883590048 ) ) ;
#21543=FACE_OUTER_BOUND ( 'NONE', #96224, .T. ) ;
#21551=CARTESIAN_POINT ( 'NONE',  ( -63.94472642409999708, 1379.737898519059854, 270.3073122244590536 ) ) ;
#21562=CARTESIAN_POINT ( 'NONE',  ( -89.64944567690000099, 1384.853425860309926, 308.7505802988590062 ) ) ;
#21564=CARTESIAN_POINT ( 'NONE',  ( -23.38007145301870082, 1385.262645945500026, 222.6269832384300003 ) ) ;
#21566=CARTESIAN_POINT ( 'NONE',  ( -9.094494643104590992, 1384.946982382309898, 199.9428547751310248 ) ) ;
#21593=CARTESIAN_POINT ( 'NONE',  ( -104.1991395359999899, 1389.999248167110181, 304.1793320542590209 ) ) ;
#21595=CARTESIAN_POINT ( 'NONE',  ( -106.1577607520000015, 1391.913060387289988, 304.2026179676590232 ) ) ;
#21599=CARTESIAN_POINT ( 'NONE',  ( -105.0207718979999925, 1379.360663349339802, 304.0316769014589795 ) ) ;
#21614=CARTESIAN_POINT ( 'NONE',  ( -106.5131656470000081, 1380.118154394319845, 307.6054082156589971 ) ) ;
#21619=CARTESIAN_POINT ( 'NONE',  ( -110.0632502760000051, 1384.922727919980161, 296.9512166178590178 ) ) ;
#21620=CARTESIAN_POINT ( 'NONE',  ( -8.999250544063707835, 1381.632011801812951, 200.5706445290884972 ) ) ;
#21632=AXIS2_PLACEMENT_3D ( 'NONE', #110085, #42890, #42328 ) ;
#21713=CARTESIAN_POINT ( 'NONE',  ( -109.1677958815039915, 1385.012782240220076, 297.1338810903739613 ) ) ;
#21727=CARTESIAN_POINT ( 'NONE',  ( -44.28647047321589980, 1383.821342991460142, 249.7482539287410077 ) ) ;
#21736=CARTESIAN_POINT ( 'NONE',  ( -34.14316623799999917, 1378.983883636150040, 218.5549180040089823 ) ) ;
#21742=CARTESIAN_POINT ( 'NONE',  ( -10.78513347949999890, 1390.743336494430196, 215.1699270643190118 ) ) ;
#21753=AXIS2_PLACEMENT_3D ( 'NONE', #101710, #6022, #23364 ) ;
#21755=ORIENTED_EDGE ( 'NONE', *, *, #66480, .F. ) ;
#21764=CARTESIAN_POINT ( 'NONE',  ( -109.9471644529999992, 1385.741605226209913, 311.4145034772590179 ) ) ;
#21773=CARTESIAN_POINT ( 'NONE',  ( -8.021176654290000485, 1385.031491206999817, 218.7854548825889935 ) ) ;
#21793=ORIENTED_EDGE ( 'NONE', *, *, #25438, .T. ) ;
#21795=CARTESIAN_POINT ( 'NONE',  ( -9.852560507769998921, 1384.650985176700033, 199.8802037849889928 ) ) ;
#21810=VECTOR ( 'NONE', #35670, 1000.000000000000000 ) ;
#21833=CARTESIAN_POINT ( 'NONE',  ( -78.73038605992259420, 1384.997356039029910, 302.9955482565979992 ) ) ;
#21834=CARTESIAN_POINT ( 'NONE',  ( -9.090173430379998365, 1385.732952333820094, 200.0315116276589720 ) ) ;
#21846=CARTESIAN_POINT ( 'NONE',  ( -107.3576381908248862, 1390.051752611091615, 299.1848643298906723 ) ) ;
#21872=FACE_OUTER_BOUND ( 'NONE', #361, .T. ) ;
#21875=CARTESIAN_POINT ( 'NONE',  ( -12.58289157959999827, 1379.610106932609824, 209.8104170840169900 ) ) ;
#21876=CARTESIAN_POINT ( 'NONE',  ( -88.41516169894879340, 1384.622141336479899, 308.1440992471430036 ) ) ;
#21877=CARTESIAN_POINT ( 'NONE',  ( -63.64159431314190840, 1385.079648997679897, 252.0084059150040048 ) ) ;
#21884=CARTESIAN_POINT ( 'NONE',  ( -109.3072984829999967, 1384.913227208139915, 311.2647025462590022 ) ) ;
#21900=CARTESIAN_POINT ( 'NONE',  ( -12.22846866959999979, 1380.845870869829923, 215.9110647297389960 ) ) ;
#21910=CARTESIAN_POINT ( 'NONE',  ( -67.35605454205490616, 1379.745124473419992, 278.5250339855529660 ) ) ;
#21922=CARTESIAN_POINT ( 'NONE',  ( -107.6824634920189965, 1378.913060387289988, 308.0758627141039483 ) ) ;
#21936=CARTESIAN_POINT ( 'NONE',  ( -14.08968533280249957, 1379.756368969990035, 211.4767688306389744 ) ) ;
#21941=B_SPLINE_CURVE_WITH_KNOTS ( 'NONE', 5,
 ( #4782, #47902, #21016, #107249, #46822, #20465 ),
 .UNSPECIFIED., .F., .F.,
 ( 6, 6 ),
 ( 0.000000000000000000, 1.000000000000000000 ),
 .UNSPECIFIED. ) ;
#21944=CARTESIAN_POINT ( 'NONE',  ( -81.42396034917169345, 1384.801295219920121, 284.9086290667029857 ) ) ;
#21973=CARTESIAN_POINT ( 'NONE',  ( -113.4000000000000057, 1387.988142337750105, 310.3973246102589769 ) ) ;
#21975=CARTESIAN_POINT ( 'NONE',  ( -8.604091250959998050, 1384.887133344300082, 199.8687245402490191 ) ) ;
#22002=CARTESIAN_POINT ( 'NONE',  ( -12.31967538714310173, 1378.053937847460020, 209.2867312577349992 ) ) ;
#22011=CARTESIAN_POINT ( 'NONE',  ( -25.34879943620689957, 1384.844904870469918, 223.9545694878910069 ) ) ;
#22012=DIRECTION ( 'NONE',  ( 6.360620485575798415E-17, 1.000000000000000000, -8.754643039332639448E-17 ) ) ;
#22017=ADVANCED_FACE ( 'NONE', ( #64105 ), #52422, .F. ) ;
#22037=CARTESIAN_POINT ( 'NONE',  ( -75.28129077213660025, 1378.304634124660197, 294.2128303316549705 ) ) ;
#22049=CARTESIAN_POINT ( 'NONE',  ( -105.5067510789999972, 1391.271045334170140, 304.2081904284589768 ) ) ;
#22054=( LENGTH_UNIT ( ) NAMED_UNIT ( * ) SI_UNIT ( .MILLI., .METRE. ) );
#22066=CARTESIAN_POINT ( 'NONE',  ( -109.9353129566706002, 1385.616331449368545, 311.4122602311213655 ) ) ;
#22070=B_SPLINE_SURFACE_WITH_KNOTS ( 'NONE', 5, 5, ( 
 ( #84165, #41627, #7465, #32120, #67401, #31559 ),
 ( #16387, #8012, #15297, #42179, #48944, #74692 ),
 ( #6368, #48388, #49489, #99301, #22575, #56779 ),
 ( #14202, #82531, #23150, #5827, #75244, #57353 ),
 ( #91478, #40514, #108824, #87502, #43837, #69060 ),
 ( #70182, #34323, #93652, #68502, #10792, #1857 ) ),
 .UNSPECIFIED., .F., .F., .F.,
 ( 6, 6 ),
 ( 6, 6 ),
 ( -0.001190444914978719881, 1.957152629518910114 ),
 ( 0.000000000000000000, 2.001190444958909964 ),
 .UNSPECIFIED. ) ;
#22075=CARTESIAN_POINT ( 'NONE',  ( -41.40570855549999862, 1375.117442312619914, 227.6002677670589947 ) ) ;
#22087=CARTESIAN_POINT ( 'NONE',  ( -67.06144730649998564, 1384.373230830070042, 292.1716250880589882 ) ) ;
#22091=CARTESIAN_POINT ( 'NONE',  ( -65.04611674080000228, 1379.740440402699960, 272.5882088742590099 ) ) ;
#22101=CARTESIAN_POINT ( 'NONE',  ( -25.94961989419999782, 1385.251886777470190, 224.2307850120589876 ) ) ;
#22103=CARTESIAN_POINT ( 'NONE',  ( -23.13586480360919850, 1385.263656115849926, 222.4840418823009998 ) ) ;
#22131=CARTESIAN_POINT ( 'NONE',  ( -103.8898683500000004, 1389.939938586880089, 304.1778429387589995 ) ) ;
#22150=CARTESIAN_POINT ( 'NONE',  ( -108.1212971963999934, 1383.758655145139983, 311.0734215935020188 ) ) ;
#22155=CARTESIAN_POINT ( 'NONE',  ( -109.9987473180000137, 1381.991098133720016, 297.9223374245589753 ) ) ;
#22200=ORIENTED_EDGE ( 'NONE', *, *, #84290, .T. ) ;
#22222=CARTESIAN_POINT ( 'NONE',  ( -12.26760366359999921, 1381.106678608419998, 202.8726028786589950 ) ) ;
#22235=CONICAL_SURFACE ( 'NONE', #99382, 12.50000000000000000, 0.02617993877989872875 ) ;
#22244=CARTESIAN_POINT ( 'NONE',  ( -14.05847445561479958, 1379.589564867563695, 211.7968567430240228 ) ) ;
#22258=CARTESIAN_POINT ( 'NONE',  ( -105.8429516820000060, 1379.429574992919925, 301.1876983431590133 ) ) ;
#22275=CARTESIAN_POINT ( 'NONE',  ( -48.77857038591120187, 1383.813927605060144, 258.8276066785749663 ) ) ;
#22283=CARTESIAN_POINT ( 'NONE',  ( -37.54707235840000124, 1380.310470099769873, 214.8595787094589866 ) ) ;
#22291=CARTESIAN_POINT ( 'NONE',  ( -13.85142996899100076, 1390.139986880880087, 212.7740396815260056 ) ) ;
#22295=CARTESIAN_POINT ( 'NONE',  ( -104.8261132509999953, 1380.717247260959994, 300.0167969450589567 ) ) ;
#22314=CARTESIAN_POINT ( 'NONE',  ( -109.6996574960000004, 1385.658284643630168, 311.3154365352589821 ) ) ;
#22324=CARTESIAN_POINT ( 'NONE',  ( -7.543563443440000071, 1384.985423750119935, 219.0866481152289964 ) ) ;
#22329=ORIENTED_EDGE ( 'NONE', *, *, #55979, .T. ) ;
#22341=CARTESIAN_POINT ( 'NONE',  ( -108.0838200535449971, 1378.913060387289988, 299.8681954501259952 ) ) ;
#22371=CARTESIAN_POINT ( 'NONE',  ( -109.1922049499590486, 1382.216944093681832, 297.5007580629779227 ) ) ;
#22375=CARTESIAN_POINT ( 'NONE',  ( -106.7031369453130054, 1391.913060387289988, 306.7753017128669626 ) ) ;
#22382=CARTESIAN_POINT ( 'NONE',  ( -92.43541484565200506, 1384.963896024199812, 309.4382857164679876 ) ) ;
#22384=CARTESIAN_POINT ( 'NONE',  ( -8.312690972840000470, 1386.943181267609816, 199.8519208937690053 ) ) ;
#22396=CARTESIAN_POINT ( 'NONE',  ( -107.2768973518786311, 1390.144646088828495, 299.2871404242311542 ) ) ;
#22419=CARTESIAN_POINT ( 'NONE',  ( -103.6308070735486524, 1379.927247807891035, 304.9220808158690375 ) ) ;
#22428=CARTESIAN_POINT ( 'NONE',  ( -65.13748019436710024, 1385.087367150850014, 255.3513583967259706 ) ) ;
#22436=CARTESIAN_POINT ( 'NONE',  ( -109.8252913419999999, 1384.913429218860074, 311.3807689642590049 ) ) ;
#22440=CARTESIAN_POINT ( 'NONE',  ( -109.8284014480000081, 1384.811872824480133, 311.3795260262589863 ) ) ;
#22461=CARTESIAN_POINT ( 'NONE',  ( -67.99044070674879947, 1379.746877581120089, 279.4179884241240188 ) ) ;
#22464=CARTESIAN_POINT ( 'NONE',  ( -11.84045693795016874, 1377.795153884136198, 212.6165618655485900 ) ) ;
#22489=CARTESIAN_POINT ( 'NONE',  ( -62.06363869513148046, 1379.731149298604578, 265.9958807297100520 ) ) ;
#22493=CARTESIAN_POINT ( 'NONE',  ( -77.18480047366641372, 1384.779630308949891, 279.0553653738320463 ) ) ;
#22503=CARTESIAN_POINT ( 'NONE',  ( -109.0351219020656828, 1384.329096908686552, 311.2187149847616752 ) ) ;
#22530=CARTESIAN_POINT ( 'NONE',  ( -109.9268356472339860, 1384.151773320029861, 311.4065111799300212 ) ) ;
#22560=CARTESIAN_POINT ( 'NONE',  ( -32.13574913744070471, 1384.820411185770126, 230.4565343730859865 ) ) ;
#22561=CARTESIAN_POINT ( 'NONE',  ( -106.9331110549079966, 1391.913060387289988, 301.8577884849000270 ) ) ;
#22575=CARTESIAN_POINT ( 'NONE',  ( -13.46738151552789908, 1379.591386266799873, 211.6550698743690191 ) ) ;
#22584=CARTESIAN_POINT ( 'NONE',  ( -7.483730530865719821, 1379.920825505379980, 211.0169310811999708 ) ) ;
#22590=EDGE_LOOP ( 'NONE', ( #79011, #93267, #66650 ) ) ;
#22614=CARTESIAN_POINT ( 'NONE',  ( -109.8119358823353338, 1386.120803211467546, 311.3368505780957207 ) ) ;
#22617=CARTESIAN_POINT ( 'NONE',  ( -12.62128053491670165, 1379.543530202440252, 209.2104001695750242 ) ) ;
#22622=CARTESIAN_POINT ( 'NONE',  ( -45.66666430340000460, 1375.391324216819839, 231.3493056147590039 ) ) ;
#22636=CARTESIAN_POINT ( 'NONE',  ( -36.25797752260000095, 1383.833857111379984, 235.3800711337590030 ) ) ;
#22651=CARTESIAN_POINT ( 'NONE',  ( -36.12389091449999512, 1385.203813137380166, 235.4649545851590062 ) ) ;
#22653=CARTESIAN_POINT ( 'NONE',  ( -42.09313388289950097, 1385.169883172800155, 245.8983665241910046 ) ) ;
#22666=CARTESIAN_POINT ( 'NONE',  ( -8.862056540259999338, 1384.892951007150259, 218.6851137892589918 ) ) ;
#22684=CARTESIAN_POINT ( 'NONE',  ( -105.5763038039999913, 1391.607272681279710, 303.0949483744590225 ) ) ;
#22691=EDGE_CURVE ( 'NONE', #49944, #81708, #70488, .T. ) ;
#22693=FACE_OUTER_BOUND ( 'NONE', #47817, .T. ) ;
#22706=CARTESIAN_POINT ( 'NONE',  ( -106.7568774629999950, 1381.977856463960052, 297.8845616112589596 ) ) ;
#22738=CARTESIAN_POINT ( 'NONE',  ( -7.964207469239999782, 1384.720725717920004, 199.4939945441389852 ) ) ;
#22787=ORIENTED_EDGE ( 'NONE', *, *, #4553, .F. ) ;
#22834=CARTESIAN_POINT ( 'NONE',  ( -38.67527654348140231, 1383.830167042470066, 239.5321249052780104 ) ) ;
#22843=CARTESIAN_POINT ( 'NONE',  ( -30.22254988470000114, 1380.278343034279942, 209.1988840933390179 ) ) ;
#22853=CARTESIAN_POINT ( 'NONE',  ( -105.6667097630000001, 1379.864153498549967, 301.0124091048589889 ) ) ;
#22870=CARTESIAN_POINT ( 'NONE',  ( -108.6463189709999995, 1386.108622646309868, 311.0727272582590217 ) ) ;
#22875=DIRECTION ( 'NONE',  ( -1.000000000000000000, 0.000000000000000000, 0.000000000000000000 ) ) ;
#22880=CARTESIAN_POINT ( 'NONE',  ( -14.22857088754179955, 1379.587268947920165, 207.8738992505469980 ) ) ;
#22894=CARTESIAN_POINT ( 'NONE',  ( -107.4518942052619934, 1378.913060387349788, 300.6024564064820197 ) ) ;
#22898=VERTEX_POINT ( 'NONE', #35303 ) ;
#22901=CARTESIAN_POINT ( 'NONE',  ( -37.21779252409999827, 1384.846743917189997, 210.1685376368189964 ) ) ;
#22905=CARTESIAN_POINT ( 'NONE',  ( -106.6183162539999927, 1379.688366450070134, 308.3260602744589960 ) ) ;
#22935=CARTESIAN_POINT ( 'NONE',  ( -105.7922123186220063, 1391.671139054730020, 305.5979281096929867 ) ) ;
#22944=CARTESIAN_POINT ( 'NONE',  ( -99.83489338526950974, 1384.946744245190075, 310.8186357852670199 ) ) ;
#22945=EDGE_CURVE ( 'NONE', #82950, #103478, #4993, .T. ) ;
#22946=CARTESIAN_POINT ( 'NONE',  ( -8.515298204750001432, 1385.582038790579873, 199.8542761591889985 ) ) ;
#22958=CARTESIAN_POINT ( 'NONE',  ( -109.4214834242509795, 1387.219425580758980, 297.3509835002536761 ) ) ;
#22974=B_SPLINE_CURVE_WITH_KNOTS ( 'NONE', 5,
 ( #930, #78159, #84354, #16562, #67578, #25531, #34505, #60274, #41799, #86559, #93300, #94392, #68681, #1471, #85438 ),
 .UNSPECIFIED., .F., .F.,
 ( 6, 3, 3, 3, 6 ),
 ( 0.000000000000000000, 0.1618001797507035155, 0.2522523987000994117, 0.4661970989643994812, 1.000000000000000000 ),
 .UNSPECIFIED. ) ;
#22985=CARTESIAN_POINT ( 'NONE',  ( -103.5801209296959939, 1379.883073482990085, 303.9981235976169955 ) ) ;
#22992=CARTESIAN_POINT ( 'NONE',  ( -12.49429521540000110, 1379.282925338159885, 210.7339652385390139 ) ) ;
#22994=CARTESIAN_POINT ( 'NONE',  ( -58.93529294637219351, 1385.056221149589874, 241.7207647726530126 ) ) ;
#23007=CARTESIAN_POINT ( 'NONE',  ( -109.3027203169999950, 1384.654548469560041, 311.2558226302590469 ) ) ;
#23016=CARTESIAN_POINT ( 'NONE',  ( -12.53694325390000053, 1380.612673806029761, 215.4769779826689842 ) ) ;
#23025=CARTESIAN_POINT ( 'NONE',  ( -109.1147032029209925, 1384.600588565270073, 311.2513737746320430 ) ) ;
#23027=CARTESIAN_POINT ( 'NONE',  ( -68.71407884372058561, 1379.747795434490172, 280.3090442124819788 ) ) ;
#23030=CARTESIAN_POINT ( 'NONE',  ( -11.56858258461559963, 1378.020591857488171, 213.4395426976007002 ) ) ;
#23031=ORIENTED_EDGE ( 'NONE', *, *, #2886, .F. ) ;
#23038=CARTESIAN_POINT ( 'NONE',  ( -106.3515999725659924, 1378.913060387349788, 306.1522039670650202 ) ) ;
#23059=CARTESIAN_POINT ( 'NONE',  ( -72.68496013324840987, 1384.753871603139942, 271.2572098337690250 ) ) ;
#23069=DIRECTION ( 'NONE',  ( -0.01668530547203104716, 0.7071067811868645414, 0.7069098956591685079 ) ) ;
#23101=CARTESIAN_POINT ( 'NONE',  ( -109.9627613373179997, 1384.389859246369952, 311.4306166055309859 ) ) ;
#23132=CARTESIAN_POINT ( 'NONE',  ( -54.44353615944859826, 1384.719267686110015, 270.7278933346339613 ) ) ;
#23150=CARTESIAN_POINT ( 'NONE',  ( -12.42270385469250016, 1378.931396367140223, 211.1644544291300178 ) ) ;
#23153=CONICAL_SURFACE ( 'NONE', #14204, 0.9999999999999857891, 0.7853981633970000820 ) ;
#23165=CARTESIAN_POINT ( 'NONE',  ( -52.34085353736339385, 1379.705649852349779, 249.9538312876250075 ) ) ;
#23188=ORIENTED_EDGE ( 'NONE', *, *, #15349, .T. ) ;
#23192=CARTESIAN_POINT ( 'NONE',  ( -107.8944167935766956, 1389.215957491298241, 309.8698152422039698 ) ) ;
#23194=CARTESIAN_POINT ( 'NONE',  ( -12.34597593048379949, 1378.750903717820165, 209.0838442145889928 ) ) ;
#23198=CARTESIAN_POINT ( 'NONE',  ( -50.14839348009999753, 1375.010081756269983, 242.5009839091590038 ) ) ;
#23212=CARTESIAN_POINT ( 'NONE',  ( -73.68066259569999943, 1383.781794063629832, 298.8244620241590042 ) ) ;
#23225=CARTESIAN_POINT ( 'NONE',  ( -19.25455816879999915, 1386.939098950560037, 220.3202894305590007 ) ) ;
#23227=CARTESIAN_POINT ( 'NONE',  ( -44.39234662709849744, 1385.156173160149820, 250.3178217652419733 ) ) ;
#23238=CARTESIAN_POINT ( 'NONE',  ( -8.297571581699999754, 1384.891077973469919, 218.7035731870690256 ) ) ;
#23254=CARTESIAN_POINT ( 'NONE',  ( -108.0517768189999970, 1387.143456978330050, 297.7515165377590165 ) ) ;
#23256=CARTESIAN_POINT ( 'NONE',  ( -106.6767654209999847, 1391.553749469950162, 300.4545537148590029 ) ) ;
#23276=AXIS2_PLACEMENT_3D ( 'NONE', #63292, #104158, #97407 ) ;
#23316=VERTEX_POINT ( 'NONE', #38341 ) ;
#23334=CARTESIAN_POINT ( 'NONE',  ( -19.84796779067900019, 1384.533059183989963, 201.6437377799259991 ) ) ;
#23364=DIRECTION ( 'NONE',  ( -1.000000000000000000, 0.000000000000000000, 0.000000000000000000 ) ) ;
#23379=CARTESIAN_POINT ( 'NONE',  ( -7.545163887449800377, 1384.911772596620040, 219.0875992466739888 ) ) ;
#23395=B_SPLINE_CURVE_WITH_KNOTS ( 'NONE', 3,
 ( #22985, #48228, #91860, #50437, #108105, #22419, #23549, #24088, #7311, #32519, #82910, #33052, #75636, #84010, #99142, #57741, #6201, #56622, #39252, #40353, #6746, #74534, #90757, #67240, #83452, #31954, #101335, #66147, #107562, #16233, #73427, #15135, #57190, #58276, #31401, #24625, #14037, #91314, #48786, #82368, #58822, #108665, #92960, #65581, #49325, #84562, #5667, #15672, #66690, #75085, #30848, #100270, #39814, #40905, #73974, #109235 ),
 .UNSPECIFIED., .F., .F.,
 ( 4, 2, 2, 2, 1, 1, 2, 2, 2, 2, 1, 1, 2, 2, 2, 2, 1, 1, 2, 2, 2, 1, 1, 1, 1, 1, 1, 2, 2, 2, 2, 2, 2, 4 ),
 ( 0.000000000000000000, 0.06250000003649344715, 0.09375000005474017073, 0.1093750000638571834, 0.1171875000684189649, 0.1210937500707053305, 0.1230468750718511778, 0.1250000000729970251, 0.1875000001098633684, 0.2187500001282965401, 0.2343750001375136671, 0.2421875001421222584, 0.2460937501444259434, 0.2500000001467296284, 0.3125000001831972352, 0.3437500002014302058, 0.3593750002105552399, 0.3671875002151185896, 0.3710937502173994318, 0.3750000002196802740, 0.4375000002557568601, 0.4687500002737773341, 0.4843750002828046131, 0.4921875002873182803, 0.4960937502895878537, 0.4980468752907154517, 0.4990234377912663999, 0.4995117190415430120, 0.5000000002918195685, 0.6250000002188711434, 0.7500000001459228294, 0.8750000000729744043, 0.9375000000364872577, 1.000000000000000000 ),
 .UNSPECIFIED. ) ;
#23400=AXIS2_PLACEMENT_3D ( 'NONE', #89598, #99635, #38642 ) ;
#23403=CARTESIAN_POINT ( 'NONE',  ( -51.69639516817590419, 1383.809142186679992, 264.8244201884630229 ) ) ;
#23412=CARTESIAN_POINT ( 'NONE',  ( -8.783909226360000488, 1382.320486701790060, 217.8959194107489736 ) ) ;
#23423=CARTESIAN_POINT ( 'NONE',  ( -107.1079164160000090, 1379.789533456470053, 299.4362131821590083 ) ) ;
#23441=CARTESIAN_POINT ( 'NONE',  ( -109.5835204229999960, 1385.270838993090138, 311.3045831672590111 ) ) ;
#23473=CARTESIAN_POINT ( 'NONE',  ( -75.49940225679999628, 1385.016445804960085, 276.6852814938590086 ) ) ;
#23505=CARTESIAN_POINT ( 'NONE',  ( -14.01399965579999929, 1379.590355683860025, 211.9184156875489862 ) ) ;
#23510=CARTESIAN_POINT ( 'NONE',  ( -108.8990485207509948, 1384.924713768860101, 311.2645749510550104 ) ) ;
#23511=CARTESIAN_POINT ( 'NONE',  ( -8.964263409860000920, 1385.771258260049763, 200.0191890160589878 ) ) ;
#23515=VECTOR ( 'NONE', #87325, 999.9999999999998863 ) ;
#23522=CARTESIAN_POINT ( 'NONE',  ( -108.8108081923106596, 1388.207833152419198, 297.7714192390470771 ) ) ;
#23545=CARTESIAN_POINT ( 'NONE',  ( -109.3495745150000005, 1384.893444084359999, 297.1386071063589611 ) ) ;
#23549=CARTESIAN_POINT ( 'NONE',  ( -103.6396175609407351, 1379.933997479830168, 304.9922815699929970 ) ) ;
#23555=CARTESIAN_POINT ( 'NONE',  ( -13.02112344040000025, 1380.010336238359969, 210.3784953617490032 ) ) ;
#23557=CARTESIAN_POINT ( 'NONE',  ( -61.13392802363229350, 1385.066938601299853, 246.4491151330799994 ) ) ;
#23558=CARTESIAN_POINT ( 'NONE',  ( -11.65231821165970061, 1391.913060387289988, 209.9483455405510028 ) ) ;
#23568=CARTESIAN_POINT ( 'NONE',  ( -109.9878148690000046, 1384.765614765949977, 311.4533902662590208 ) ) ;
#23587=CARTESIAN_POINT ( 'NONE',  ( -68.66102733441179851, 1379.747688256459924, 280.2626083829800336 ) ) ;
#23591=CARTESIAN_POINT ( 'NONE',  ( -10.49976491246964017, 1379.056602952379990, 215.6293701293769800 ) ) ;
#23600=CARTESIAN_POINT ( 'NONE',  ( -107.3791820827839985, 1378.913060387289988, 307.6919078974059971 ) ) ;
#23625=CARTESIAN_POINT ( 'NONE',  ( -10.79387578689999927, 1391.590462314130036, 214.7676431958390140 ) ) ;
#23626=CARTESIAN_POINT ( 'NONE',  ( -69.45604853682949908, 1384.733805731689927, 264.7784157945660013 ) ) ;
#23648=VERTEX_POINT ( 'NONE', #59862 ) ;
#23657=CARTESIAN_POINT ( 'NONE',  ( -8.156254201879999499, 1384.896657262430153, 199.6468321548190090 ) ) ;
#23674=CARTESIAN_POINT ( 'NONE',  ( -7.794443285332278037, 1386.710985943309879, 218.8404340897528186 ) ) ;
#23689=CARTESIAN_POINT ( 'NONE',  ( -50.03546363177220968, 1384.739880094399950, 261.8130513971230471 ) ) ;
#23697=CARTESIAN_POINT ( 'NONE',  ( -11.14745452005457871, 1378.905166874835913, 203.8219142046758634 ) ) ;
#23706=FACE_OUTER_BOUND ( 'NONE', #60217, .T. ) ;
#23717=CARTESIAN_POINT ( 'NONE',  ( -36.47250856561959864, 1379.658678557460007, 223.7669085669769800 ) ) ;
#23719=ORIENTED_EDGE ( 'NONE', *, *, #24991, .T. ) ;
#23743=CARTESIAN_POINT ( 'NONE',  ( -108.4309645088232088, 1388.536554251156758, 310.3699996483296104 ) ) ;
#23750=CARTESIAN_POINT ( 'NONE',  ( -19.16011842089999817, 1379.988729378269909, 208.8610751811399950 ) ) ;
#23763=CARTESIAN_POINT ( 'NONE',  ( -49.59998741779999420, 1384.429563225830179, 260.9046511607589878 ) ) ;
#23775=CARTESIAN_POINT ( 'NONE',  ( -74.54124110130000247, 1388.281602540309905, 277.2607202525589969 ) ) ;
#23777=CARTESIAN_POINT ( 'NONE',  ( -38.52179989938650095, 1385.190298941179890, 239.5872078768659890 ) ) ;
#23785=CARTESIAN_POINT ( 'NONE',  ( -8.861530393209999801, 1384.875119385939797, 218.6849572728390285 ) ) ;
#23801=CARTESIAN_POINT ( 'NONE',  ( -106.8356828860000007, 1390.011699867550078, 299.6508205978589672 ) ) ;
#23803=CARTESIAN_POINT ( 'NONE',  ( -106.1967435559999871, 1391.345933298020100, 301.1341274642589951 ) ) ;
#23821=B_SPLINE_CURVE_WITH_KNOTS ( 'NONE', 3,
 ( #27794, #71502, #97197, #27244, #87151, #70384, #61425, #3175, #104501, #61981, #53575, #96096 ),
 .UNSPECIFIED., .F., .F.,
 ( 4, 2, 2, 2, 2, 4 ),
 ( -0.08068999410833509189, -0.06416485085002331112, -0.04444643289188129898, -0.02282564341193510371, 0.000000000000000000, 0.0003431288226209555647 ),
 .UNSPECIFIED. ) ;
#23857=ORIENTED_EDGE ( 'NONE', *, *, #11837, .T. ) ;
#23860=ORIENTED_EDGE ( 'NONE', *, *, #37130, .T. ) ;
#23868=ORIENTED_EDGE ( 'NONE', *, *, #37704, .T. ) ;
#23873=CARTESIAN_POINT ( 'NONE',  ( -40.26705673720950074, 1384.583644506999917, 213.1675334149419996 ) ) ;
#23878=ORIENTED_EDGE ( 'NONE', *, *, #96295, .T. ) ;
#23887=CARTESIAN_POINT ( 'NONE',  ( -68.76290618570000390, 1379.747985224000104, 280.1898727115589622 ) ) ;
#23910=VERTEX_POINT ( 'NONE', #107357 ) ;
#23918=CARTESIAN_POINT ( 'NONE',  ( -7.545177104707559756, 1384.914515597359923, 219.0875873435799974 ) ) ;
#23939=CARTESIAN_POINT ( 'NONE',  ( -42.01758979030880425, 1383.824999389499908, 245.4151092701270045 ) ) ;
#23947=CARTESIAN_POINT ( 'NONE',  ( -46.58469234310000218, 1379.055167030529901, 234.6844865969590046 ) ) ;
#23952=CARTESIAN_POINT ( 'NONE',  ( -7.679213435265119791, 1385.492375165610156, 218.9666595514219978 ) ) ;
#23958=CARTESIAN_POINT ( 'NONE',  ( -107.4881158890000137, 1380.862912516779943, 298.8296354258590100 ) ) ;
#23977=CARTESIAN_POINT ( 'NONE',  ( -108.1428528709999881, 1386.591709523359896, 310.8553624892590506 ) ) ;
#23991=DIRECTION ( 'NONE',  ( -1.000000000000000000, 0.000000000000000000, 0.000000000000000000 ) ) ;
#24003=CARTESIAN_POINT ( 'NONE',  ( -46.09372478569999743, 1384.870670475119823, 219.0248111663489965 ) ) ;
#24009=EDGE_CURVE ( 'NONE', #82014, #96593, #38271, .T. ) ;
#24014=CARTESIAN_POINT ( 'NONE',  ( -10.56579291990400016, 1391.913060387269979, 204.9477986745440319 ) ) ;
#24035=CARTESIAN_POINT ( 'NONE',  ( -11.70763562119999968, 1378.584671346379992, 213.2295515425790029 ) ) ;
#24046=CARTESIAN_POINT ( 'NONE',  ( -11.98665338999999896, 1391.172375739130075, 205.5831304284690191 ) ) ;
#24049=EDGE_CURVE ( 'NONE', #96085, #50916, #52974, .T. ) ;
#24083=CARTESIAN_POINT ( 'NONE',  ( -110.0629570050000012, 1384.907242112629774, 296.9512948280589626 ) ) ;
#24086=EDGE_CURVE ( 'NONE', #19741, #16403, #82456, .T. ) ;
#24088=CARTESIAN_POINT ( 'NONE',  ( -103.6552259873821100, 1379.945806083001571, 305.1021558360112635 ) ) ;
#24091=CARTESIAN_POINT ( 'NONE',  ( -108.3926162938884801, 1381.231319549018281, 310.3369704220332892 ) ) ;
#24094=CARTESIAN_POINT ( 'NONE',  ( -57.85475636940380184, 1385.051150463449858, 239.4744903710780193 ) ) ;
#24095=CARTESIAN_POINT ( 'NONE',  ( -11.57078835683859985, 1391.913060387289988, 210.5928294217469841 ) ) ;
#24104=CARTESIAN_POINT ( 'NONE',  ( -109.9744337340000016, 1384.497115240790208, 311.4392815102590362 ) ) ;
#24119=CARTESIAN_POINT ( 'NONE',  ( -109.1329681763050132, 1384.757089681630077, 311.2614977992300282 ) ) ;
#24122=CARTESIAN_POINT ( 'NONE',  ( -68.53711315337859844, 1379.747442305619870, 280.1339386914270335 ) ) ;
#24124=CARTESIAN_POINT ( 'NONE',  ( -8.564985822174367769, 1381.538787820967173, 218.1048692684619539 ) ) ;
#24133=B_SPLINE_SURFACE_WITH_KNOTS ( 'NONE', 5, 5, ( 
 ( #72942, #45008, #46109, #80240, #71330, #107080 ),
 ( #55056, #28732, #61813, #53971, #45562, #97049 ),
 ( #20312, #3559, #71886, #108175, #108734, #65648 ),
 ( #66760, #92466, #40972, #99764, #57262, #74046 ),
 ( #100333, #109299, #15737, #74598, #98677, #30918 ),
 ( #32025, #49938, #13549, #73501, #32584, #91390 ) ),
 .UNSPECIFIED., .F., .F., .F.,
 ( 6, 6 ),
 ( 6, 6 ),
 ( 0.000000000000000000, 0.5294136330519999545 ),
 ( 0.000000000000000000, 2.000000000000000000 ),
 .UNSPECIFIED. ) ;
#24156=CARTESIAN_POINT ( 'NONE',  ( -11.50315952000000053, 1391.841514381249908, 212.6496336906789963 ) ) ;
#24157=CARTESIAN_POINT ( 'NONE',  ( -85.15111601059649615, 1384.818475995900144, 288.8775456395259766 ) ) ;
#24176=CARTESIAN_POINT ( 'NONE',  ( -60.00250937820000274, 1379.736434133900048, 261.8124847885590043 ) ) ;
#24181=B_SPLINE_SURFACE_WITH_KNOTS ( 'NONE', 5, 5, ( 
 ( #45560, #88650, #3556, #61810, #70226, #38220 ),
 ( #27624, #53396, #36576, #19767, #95932, #62362 ),
 ( #97047, #87545, #37128, #29275, #11927, #45005 ),
 ( #79149, #80236, #4095, #3006, #29820, #2460 ),
 ( #46657, #78583, #105999, #72402, #46107, #64009 ),
 ( #79701, #97586, #70774, #104885, #89181, #98120 ) ),
 .UNSPECIFIED., .F., .F., .F.,
 ( 6, 6 ),
 ( 6, 6 ),
 ( 0.9325643087039999779, 1.051317469700000062 ),
 ( 0.000000000000000000, 2.000000000000000000 ),
 .UNSPECIFIED. ) ;
#24199=CARTESIAN_POINT ( 'NONE',  ( -109.7733655239769917, 1383.592504427309905, 311.3137736610110551 ) ) ;
#24203=EDGE_CURVE ( 'NONE', #8701, #15055, #6356, .T. ) ;
#24214=VECTOR ( 'NONE', #8813, 1000.000000000000000 ) ;
#24234=CARTESIAN_POINT ( 'NONE',  ( -51.53422708892170334, 1384.732738490049996, 264.8871901791150094 ) ) ;
#24235=CARTESIAN_POINT ( 'NONE',  ( -106.8411176217500014, 1391.913060387289988, 302.0741137023289298 ) ) ;
#24243=CARTESIAN_POINT ( 'NONE',  ( -8.536583043757159928, 1382.467666485138807, 200.0783688444290362 ) ) ;
#24265=CARTESIAN_POINT ( 'NONE',  ( -7.468813707570000737, 1377.075590846060095, 211.4935550762889989 ) ) ;
#24267=CARTESIAN_POINT ( 'NONE',  ( -52.29426375968220242, 1379.697094711749969, 249.9767541960729886 ) ) ;
#24273=CARTESIAN_POINT ( 'NONE',  ( -105.5253899740000065, 1379.039621664339847, 305.7477329845589793 ) ) ;
#24294=CARTESIAN_POINT ( 'NONE',  ( -107.6660152849997587, 1389.491633112957743, 309.6288604638345419 ) ) ;
#24301=CARTESIAN_POINT ( 'NONE',  ( -7.543040680839999901, 1380.366160257679894, 209.1218465795010104 ) ) ;
#24315=CARTESIAN_POINT ( 'NONE',  ( -76.10119759110000359, 1384.646775243249976, 301.2182732922589707 ) ) ;
#24328=CARTESIAN_POINT ( 'NONE',  ( -55.00753619759999680, 1390.789904819489948, 252.7470035923590217 ) ) ;
#24330=CARTESIAN_POINT ( 'NONE',  ( -49.49710368664120352, 1385.125075197469869, 260.6903207721879312 ) ) ;
#24341=CARTESIAN_POINT ( 'NONE',  ( -7.545020166129999595, 1384.905783835959937, 219.0876432053290159 ) ) ;
#24356=CARTESIAN_POINT ( 'NONE',  ( -109.0713608260000029, 1386.631206999619735, 297.4104235875589666 ) ) ;
#24389=CARTESIAN_POINT ( 'NONE',  ( -12.30975638026900043, 1378.376095226579992, 209.8073264528339905 ) ) ;
#24406=CARTESIAN_POINT ( 'NONE',  ( -8.157610789389998729, 1384.622758710029984, 199.6574702203289746 ) ) ;
#24412=CIRCLE ( 'NONE', #87013, 0.9999999999999955591 ) ;
#24428=CARTESIAN_POINT ( 'NONE',  ( -32.14450299649809750, 1384.561384632279896, 206.8209701602499990 ) ) ;
#24442=CIRCLE ( 'NONE', #58447, 7.513264357030008611 ) ;
#24470=CARTESIAN_POINT ( 'NONE',  ( -105.0631825244292372, 1390.534411153809060, 304.1916690124131719 ) ) ;
#24494=CARTESIAN_POINT ( 'NONE',  ( -73.02464777688889797, 1383.782474506479957, 297.9868448762199478 ) ) ;
#24501=CARTESIAN_POINT ( 'NONE',  ( -72.24957631569999705, 1381.775758148160094, 272.8158467630589712 ) ) ;
#24505=CARTESIAN_POINT ( 'NONE',  ( -8.508204430222377823, 1386.516060600280071, 218.4508996449510221 ) ) ;
#24511=CARTESIAN_POINT ( 'NONE',  ( -105.6757023109999949, 1378.000557810240025, 302.9257663873589763 ) ) ;
#24531=CARTESIAN_POINT ( 'NONE',  ( -107.1491673510000027, 1387.396471041590075, 310.3410155632590204 ) ) ;
#24539=CARTESIAN_POINT ( 'NONE',  ( -14.34470072367650140, 1379.595425982329971, 208.0071153785060005 ) ) ;
#24565=CARTESIAN_POINT ( 'NONE',  ( -11.01364452973389874, 1391.913060387030100, 206.0332053900289964 ) ) ;
#24586=CARTESIAN_POINT ( 'NONE',  ( -11.92968414179999925, 1378.045929578360074, 212.2475929956690095 ) ) ;
#24592=CARTESIAN_POINT ( 'NONE',  ( -12.22845464540000116, 1392.111545638959797, 206.8354075410990163 ) ) ;
#24597=CARTESIAN_POINT ( 'NONE',  ( -8.860260194638639675, 1384.841874547059888, 218.6844059295819989 ) ) ;
#24611=CARTESIAN_POINT ( 'NONE',  ( -14.58219550427210010, 1383.858962634210002, 219.1768149639169962 ) ) ;
#24621=PLANE ( 'NONE',  #31800 ) ;
#24625=CARTESIAN_POINT ( 'NONE',  ( -104.9411529111025487, 1380.860630878966958, 308.2816869617895463 ) ) ;
#24634=CARTESIAN_POINT ( 'NONE',  ( -67.47041654031760061, 1385.099433479379968, 260.5101198769480106 ) ) ;
#24635=CARTESIAN_POINT ( 'NONE',  ( -11.64091994802049790, 1391.913060387289988, 210.0754932155269898 ) ) ;
#24659=CARTESIAN_POINT ( 'NONE',  ( -109.1646618499602397, 1384.891810334096363, 297.1326802748606610 ) ) ;
#24661=CARTESIAN_POINT ( 'NONE',  ( -68.44952925478749250, 1379.747226849109893, 280.0582246923240177 ) ) ;
#24663=CARTESIAN_POINT ( 'NONE',  ( -9.668563137246193762, 1379.991352563589089, 216.8468033706864730 ) ) ;
#24698=CARTESIAN_POINT ( 'NONE',  ( -11.40910167059999836, 1391.913060387289988, 211.4454899872289957 ) ) ;
#24700=CARTESIAN_POINT ( 'NONE',  ( -103.0456467999559891, 1384.883686176350011, 296.7218882600220127 ) ) ;
#24701=ORIENTED_EDGE ( 'NONE', *, *, #92741, .F. ) ;
#24718=CARTESIAN_POINT ( 'NONE',  ( -63.91816553489999819, 1379.742600501299876, 270.3198227003589977 ) ) ;
#24733=CARTESIAN_POINT ( 'NONE',  ( -8.604799066060000001, 1384.909923716469848, 199.8686514356990074 ) ) ;
#24752=CARTESIAN_POINT ( 'NONE',  ( -8.062121734079813251, 1387.317230855839398, 218.5919200099478701 ) ) ;
#24762=EDGE_CURVE ( 'NONE', #7882, #7907, #58122, .T. ) ;
#24763=DIRECTION ( 'NONE',  ( -0.01668530547203130737, -0.7071067811868645414, 0.7069098956591685079 ) ) ;
#24770=CARTESIAN_POINT ( 'NONE',  ( -47.91296898077749944, 1384.750118820870057, 257.4434400084929848 ) ) ;
#24771=CARTESIAN_POINT ( 'NONE',  ( -106.4020803887899973, 1391.913060387289988, 304.0987531970990290 ) ) ;
#24773=CARTESIAN_POINT ( 'NONE',  ( -107.4477388159999975, 1379.886884385820167, 299.0757729400589824 ) ) ;
#24778=CARTESIAN_POINT ( 'NONE',  ( -11.93976775657317013, 1378.024740770806602, 206.0762735010970061 ) ) ;
#24798=CARTESIAN_POINT ( 'NONE',  ( -24.42450952024000088, 1377.857503279539969, 215.6133220620030215 ) ) ;
#24801=CARTESIAN_POINT ( 'NONE',  ( -48.15636025208650040, 1379.711680487519970, 241.4636575790609925 ) ) ;
#24807=CARTESIAN_POINT ( 'NONE',  ( -105.9298767669999961, 1379.081211923699811, 306.7609391451590000 ) ) ;
#24839=CARTESIAN_POINT ( 'NONE',  ( -3.771520291289999882, 1375.697147833719782, 207.5503167614189977 ) ) ;
#24853=CARTESIAN_POINT ( 'NONE',  ( -106.4241660069999966, 1383.759861017009825, 311.1380007012590454 ) ) ;
#24865=CARTESIAN_POINT ( 'NONE',  ( -59.30951814779999864, 1386.658176173940092, 279.8843003692589946 ) ) ;
#24867=CARTESIAN_POINT ( 'NONE',  ( -52.91940571912499536, 1385.104601948549998, 267.6864206406419839 ) ) ;
#24876=CARTESIAN_POINT ( 'NONE',  ( -106.2815139762350043, 1381.801306631560010, 309.7257556431679859 ) ) ;
#24890=CARTESIAN_POINT ( 'NONE',  ( -109.2614022059999996, 1385.672371935979982, 297.1866512157590705 ) ) ;
#24905=AXIS2_PLACEMENT_3D ( 'NONE', #94177, #10183, #44357 ) ;
#24923=CARTESIAN_POINT ( 'NONE',  ( -12.29749543468789952, 1378.326909674530043, 209.9820058553110016 ) ) ;
#24934=EDGE_LOOP ( 'NONE', ( #98640, #82453, #35888, #110222, #37312 ) ) ;
#24942=CARTESIAN_POINT ( 'NONE',  ( -8.862552377930001057, 1384.556343050050145, 199.9458714445790122 ) ) ;
#24965=CARTESIAN_POINT ( 'NONE',  ( -113.4000000000000057, 1378.483856714079820, 302.0293834673589686 ) ) ;
#24971=CARTESIAN_POINT ( 'NONE',  ( -42.50641556133220433, 1384.590798579960165, 215.4612014908259710 ) ) ;
#24980=CARTESIAN_POINT ( 'NONE',  ( -67.28024477550941640, 1379.744889785224586, 278.5190817744257856 ) ) ;
#24987=CARTESIAN_POINT ( 'NONE',  ( -68.74238773750001030, 1379.747863086420011, 280.1036906554590473 ) ) ;
#24991=EDGE_CURVE ( 'NONE', #96085, #83875, #20630, .T. ) ;
#25006=DIRECTION ( 'NONE',  ( -1.836970198721029688E-16, -1.000000000000000000, 0.000000000000000000 ) ) ;
#25042=CARTESIAN_POINT ( 'NONE',  ( -68.92988442230469559, 1383.786281746080022, 293.5620293669300054 ) ) ;
#25044=DIRECTION ( 'NONE',  ( -0.05481995565582255259, -0.1266070825601602612, -0.9904369839154324451 ) ) ;
#25050=CARTESIAN_POINT ( 'NONE',  ( -51.40360984529999655, 1380.961789557690054, 260.0749407918589782 ) ) ;
#25061=CARTESIAN_POINT ( 'NONE',  ( -109.1959892269999983, 1382.683563420089968, 297.4542923961590191 ) ) ;
#25084=CARTESIAN_POINT ( 'NONE',  ( -106.9425809150000077, 1387.746739512440172, 310.0310650472589487 ) ) ;
#25109=ORIENTED_EDGE ( 'NONE', *, *, #100767, .F. ) ;
#25123=CARTESIAN_POINT ( 'NONE',  ( -10.37958022962100024, 1391.913060387289988, 204.5402316943800258 ) ) ;
#25136=CARTESIAN_POINT ( 'NONE',  ( -9.852819229099999632, 1386.608977785310117, 199.8799424390689978 ) ) ;
#25144=CARTESIAN_POINT ( 'NONE',  ( -12.97372998250000009, 1379.811305717160167, 213.3571419713289856 ) ) ;
#25148=CONICAL_SURFACE ( 'NONE', #23400, 12.49999999999999467, 0.02617993877989872875 ) ;
#25151=CARTESIAN_POINT ( 'NONE',  ( -11.20689792730000001, 1390.718236914620093, 203.7291915516989889 ) ) ;
#25157=CARTESIAN_POINT ( 'NONE',  ( -9.025258063816389509, 1384.071087798369945, 218.5842451692199973 ) ) ;
#25185=FACE_OUTER_BOUND ( 'NONE', #85757, .T. ) ;
#25195=CARTESIAN_POINT ( 'NONE',  ( -11.62395736679999914, 1391.913060387289988, 208.2888796421599977 ) ) ;
#25196=CARTESIAN_POINT ( 'NONE',  ( -68.09493305640410199, 1385.102643623660015, 261.8663954522849622 ) ) ;
#25197=CARTESIAN_POINT ( 'NONE',  ( -10.76416396095310013, 1391.913060387289988, 213.0502257285290284 ) ) ;
#25221=CARTESIAN_POINT ( 'NONE',  ( -68.55949274003370419, 1379.747596899770087, 280.1521097459560110 ) ) ;
#25224=ORIENTED_EDGE ( 'NONE', *, *, #78940, .T. ) ;
#25235=CARTESIAN_POINT ( 'NONE',  ( -12.45166823054470129, 1378.738365027170175, 209.0955970008419911 ) ) ;
#25243=DIRECTION ( 'NONE',  ( 0.9998780035959986545, 0.000000000000000000, -0.01561979272846077127 ) ) ;
#25249=CARTESIAN_POINT ( 'NONE',  ( -14.19917317546740065, 1380.177169543179843, 210.7455613943569972 ) ) ;
#25257=CARTESIAN_POINT ( 'NONE',  ( -87.73050061784429943, 1384.829504049740081, 291.0308553036180115 ) ) ;
#25275=CARTESIAN_POINT ( 'NONE',  ( -52.00740111290000556, 1379.696047019589969, 243.6069664339590020 ) ) ;
#25326=CARTESIAN_POINT ( 'NONE',  ( -11.44054303565944686, 1391.153937848091800, 213.9067438120043221 ) ) ;
#25328=CARTESIAN_POINT ( 'NONE',  ( -57.60540916714719373, 1384.705479994730013, 276.7345517628079961 ) ) ;
#25329=CARTESIAN_POINT ( 'NONE',  ( -19.85270156754270232, 1384.950477623580127, 201.6204297621999899 ) ) ;
#25331=CARTESIAN_POINT ( 'NONE',  ( -107.8626300280000123, 1378.913060387289988, 300.1243669462589878 ) ) ;
#25336=CARTESIAN_POINT ( 'NONE',  ( -9.211456433762755580, 1381.302692241149771, 200.8120824927987087 ) ) ;
#25346=FACE_OUTER_BOUND ( 'NONE', #75485, .T. ) ;
#25360=CARTESIAN_POINT ( 'NONE',  ( -56.97967810409669909, 1379.730140100299877, 259.4601704726770208 ) ) ;
#25362=ORIENTED_EDGE ( 'NONE', *, *, #30897, .F. ) ;
#25366=CARTESIAN_POINT ( 'NONE',  ( -105.1200804420000026, 1379.260731124600170, 305.2465900763589843 ) ) ;
#25393=CARTESIAN_POINT ( 'NONE',  ( 1.079600664838949807E-13, 1377.913060387289988, 206.3143084471490170 ) ) ;
#25408=EDGE_CURVE ( 'NONE', #43960, #23910, #9866, .T. ) ;
#25417=CARTESIAN_POINT ( 'NONE',  ( -55.17517041340000361, 1388.273123790759882, 269.8705547383589760 ) ) ;
#25419=CARTESIAN_POINT ( 'NONE',  ( -70.15791120722559526, 1385.023615900659934, 295.2473282410489901 ) ) ;
#25420=VECTOR ( 'NONE', #9915, 999.9999999999998863 ) ;
#25431=CARTESIAN_POINT ( 'NONE',  ( -107.4010429502839941, 1381.980278631019701, 310.0687908842899674 ) ) ;
#25438=EDGE_CURVE ( 'NONE', #76524, #90041, #11786, .T. ) ;
#25446=CARTESIAN_POINT ( 'NONE',  ( -105.8185367562990251, 1391.163754585894822, 301.8502271879565910 ) ) ;
#25448=CARTESIAN_POINT ( 'NONE',  ( -109.3474494770000121, 1386.224464844990280, 297.2624775481590405 ) ) ;
#25474=CARTESIAN_POINT ( 'NONE',  ( -12.24671249752945812, 1378.552623650818987, 211.6779590916783036 ) ) ;
#25485=CARTESIAN_POINT ( 'NONE',  ( -12.29128949743470045, 1378.278888474700125, 210.0499278134209931 ) ) ;
#25512=ORIENTED_EDGE ( 'NONE', *, *, #174, .F. ) ;
#25513=ORIENTED_EDGE ( 'NONE', *, *, #58995, .F. ) ;
#25529=CARTESIAN_POINT ( 'NONE',  ( -43.36595167702599696, 1384.593702623199988, 216.4150399315160200 ) ) ;
#25531=CARTESIAN_POINT ( 'NONE',  ( -108.2808028870000072, 1386.465776205880047, 310.9170304772590043 ) ) ;
#25536=CARTESIAN_POINT ( 'NONE',  ( -39.57835122609379397, 1379.656430289635182, 228.3944668109967040 ) ) ;
#25541=CARTESIAN_POINT ( 'NONE',  ( -68.68489780340000550, 1379.748151576980035, 279.9908545622590168 ) ) ;
#25578=ADVANCED_FACE ( 'NONE', ( #68210 ), #77972, .T. ) ;
#25598=CARTESIAN_POINT ( 'NONE',  ( -64.48517748775938685, 1383.791068212090067, 287.7044658124170269 ) ) ;
#25605=CARTESIAN_POINT ( 'NONE',  ( -35.50363208510000135, 1379.896902233160063, 227.2934423945590083 ) ) ;
#25616=CARTESIAN_POINT ( 'NONE',  ( -107.0843635519999992, 1382.329134876569924, 298.0462323021590691 ) ) ;
#25639=CARTESIAN_POINT ( 'NONE',  ( -104.4869036590000064, 1389.270867165570053, 307.8650956148590012 ) ) ;
#25671=CARTESIAN_POINT ( 'NONE',  ( -109.9854347995050006, 1384.902532624669902, 311.4562314680339910 ) ) ;
#25677=CARTESIAN_POINT ( 'NONE',  ( -11.60429320023880173, 1391.913060387170162, 208.2952356049119658 ) ) ;
#25696=CARTESIAN_POINT ( 'NONE',  ( -12.00298711920000017, 1378.730876743509953, 212.7098913336589874 ) ) ;
#25702=CARTESIAN_POINT ( 'NONE',  ( -10.22564300610000032, 1389.880884843570129, 202.1309545629490003 ) ) ;
#25741=CARTESIAN_POINT ( 'NONE',  ( -11.97102458384909873, 1391.459503355940114, 212.4918544850630155 ) ) ;
#25745=CARTESIAN_POINT ( 'NONE',  ( -109.2894791384494653, 1382.540884933779353, 311.0173327546005453 ) ) ;
#25750=CARTESIAN_POINT ( 'NONE',  ( -77.54836707579930533, 1385.147474671279952, 279.6196463459559709 ) ) ;
#25770=DIRECTION ( 'NONE',  ( 0.000000000000000000, 0.000000000000000000, -1.000000000000000000 ) ) ;
#25775=B_SPLINE_SURFACE_WITH_KNOTS ( 'NONE', 5, 5, ( 
 ( #26604, #103874, #17068, #18199, #44534, #36677 ),
 ( #94926, #10928, #104429, #61359, #1421, #27721 ),
 ( #53497, #52396, #86519, #9812, #45104, #51265 ),
 ( #77033, #85398, #95478, #34466, #43978, #18745 ),
 ( #30470, #106623, #38861, #54608, #13642, #72494 ),
 ( #89826, #55705, #12575, #5271, #89278, #64656 ),
 ( #46204, #98775, #96588, #28273, #37232, #62466 ),
 ( #47832, #98223, #22037, #4717, #3103, #55157 ),
 ( #37784, #29910, #64102, #38315, #80338, #71428 ),
 ( #20403, #71973, #21493, #13098, #81965, #54063 ),
 ( #80886, #88190, #46755, #81405, #19860, #3655 ),
 ( #56234, #88739, #105544, #11482, #4182, #73039 ),
 ( #90364, #47282, #28831, #107178, #104983, #70870 ),
 ( #45658, #12024, #79797, #63029, #97134, #106085 ),
 ( #29363, #63564, #97679, #20952, #92573, #65198 ),
 ( #75793, #33223, #15307, #31018, #109945, #6921 ),
 ( #57900, #83085, #59003, #92035, #67412, #101512 ),
 ( #41077, #50049, #14767, #49499, #84724, #74153 ),
 ( #75255, #24798, #16398, #57363, #83624, #39977 ),
 ( #109404, #99864, #91487, #6378, #73603, #48398 ),
 ( #100968, #107733, #5837, #108283, #58445, #108833 ),
 ( #24265, #15844, #50593, #22584, #56789, #32680 ),
 ( #48954, #7476, #14212, #40524, #74702, #66859 ),
 ( #90926, #99310, #93131, #84178, #82541, #31570 ) ),
 .UNSPECIFIED., .F., .F., .F.,
 ( 6, 3, 3, 3, 3, 3, 3, 6 ),
 ( 6, 6 ),
 ( 0.000000000000000000, 19.27951045849999900, 37.56883265599999788, 64.75259520960000259, 97.48063803579999842, 123.9428332119999965, 141.7919792689999952, 160.6499452009999800 ),
 ( 3.122614431000000135, 7.854052422239930387 ),
 .UNSPECIFIED. ) ;
#25790=CARTESIAN_POINT ( 'NONE',  ( -13.06508296313580075, 1379.379227062329846, 208.5508266283169689 ) ) ;
#25811=CARTESIAN_POINT ( 'NONE',  ( -104.7048071253149999, 1384.888671349390052, 296.8869291217460500 ) ) ;
#25827=CARTESIAN_POINT ( 'NONE',  ( -26.01816549270000323, 1379.613343931319832, 211.4995553492590261 ) ) ;
#25842=CARTESIAN_POINT ( 'NONE',  ( -8.156721943249999995, 1384.915541804160057, 199.6468728678090088 ) ) ;
#25883=CARTESIAN_POINT ( 'NONE',  ( -80.81157604502008951, 1384.636890264109979, 304.3801429775080578 ) ) ;
#25888=CARTESIAN_POINT ( 'NONE',  ( -107.5501839869999969, 1379.272371748259957, 299.1643429852589975 ) ) ;
#25901=CARTESIAN_POINT ( 'NONE',  ( -8.875403779870000065, 1384.475744450559887, 199.9572675252190095 ) ) ;
#25914=CARTESIAN_POINT ( 'NONE',  ( -60.10696580412420076, 1379.726343179680043, 266.0067701417399917 ) ) ;
#25920=CARTESIAN_POINT ( 'NONE',  ( -106.6672824069999876, 1379.424819370810155, 308.2861885763590521 ) ) ;
#25923=CARTESIAN_POINT ( 'NONE',  ( -7.567240553890000498, 1385.515681772639937, 219.0512273331090114 ) ) ;
#25933=CONICAL_SURFACE ( 'NONE', #63553, 7.999999999999996447, 0.02617993877989872875 ) ;
#25946=CARTESIAN_POINT ( 'NONE',  ( -108.0661742336610018, 1378.913060387289988, 308.5496305239910271 ) ) ;
#25947=CARTESIAN_POINT ( 'NONE',  ( -35.68096903199556635, 1379.642192106147149, 218.6344609364291500 ) ) ;
#25948=CARTESIAN_POINT ( 'NONE',  ( -7.630907732839999902, 1377.866160257680122, 206.3143087701089939 ) ) ;
#25969=B_SPLINE_CURVE_WITH_KNOTS ( 'NONE', 3,
 ( #70169, #87491, #28116, #96435 ),
 .UNSPECIFIED., .F., .F.,
 ( 4, 4 ),
 ( -23.36254398669999688, -0.7259150538130008101 ),
 .UNSPECIFIED. ) ;
#25972=CARTESIAN_POINT ( 'NONE',  ( -96.24084593199999915, 1384.955172021569979, 310.5859090792589541 ) ) ;
#25974=CARTESIAN_POINT ( 'NONE',  ( -57.60619611540929697, 1385.078379728229947, 276.7333735769680061 ) ) ;
#25984=CARTESIAN_POINT ( 'NONE',  ( -109.5250186310779981, 1383.241630048620209, 311.1713175981399786 ) ) ;
#25998=EDGE_CURVE ( 'NONE', #48821, #105177, #56477, .T. ) ;
#26014=CARTESIAN_POINT ( 'NONE',  ( -11.28131443171900017, 1384.886896985610065, 218.8719869723099976 ) ) ;
#26079=CARTESIAN_POINT ( 'NONE',  ( -73.12095152039999846, 1385.004348552520014, 272.3390795393589769 ) ) ;
#26081=CARTESIAN_POINT ( 'NONE',  ( -38.53560686260429691, 1384.578460514909921, 211.5649073465099832 ) ) ;
#26093=CARTESIAN_POINT ( 'NONE',  ( -68.70867971649998651, 1379.747832788930054, 279.9818316718590268 ) ) ;
#26101=CARTESIAN_POINT ( 'NONE',  ( -17.46966162369999864, 1385.147636303250010, 219.9515191535590191 ) ) ;
#26103=CARTESIAN_POINT ( 'NONE',  ( -12.47378745274919964, 1385.303368465689800, 218.9863576209239966 ) ) ;
#26117=VERTEX_POINT ( 'NONE', #44952 ) ;
#26151=CARTESIAN_POINT ( 'NONE',  ( -70.29742853679998404, 1383.784953440819891, 295.1360135794139978 ) ) ;
#26160=CARTESIAN_POINT ( 'NONE',  ( -50.70917129120000055, 1383.085947422079926, 226.2616357312589912 ) ) ;
#26163=VERTEX_POINT ( 'NONE', #35144 ) ;
#26169=DIRECTION ( 'NONE',  ( -0.5877852522927941026, 1.077399419887002351E-16, 0.8090169943747143044 ) ) ;
#26170=CARTESIAN_POINT ( 'NONE',  ( -109.3407845659999964, 1384.040961356549815, 297.1897130710590318 ) ) ;
#26194=CARTESIAN_POINT ( 'NONE',  ( -104.4762617860000091, 1389.781270533860152, 306.5625267145589987 ) ) ;
#26229=CARTESIAN_POINT ( 'NONE',  ( -109.9849400530580112, 1384.915723531200001, 311.4561069221339835 ) ) ;
#26248=CARTESIAN_POINT ( 'NONE',  ( -6.042424523860000285, 1389.870610953139931, 214.5741421020690041 ) ) ;
#26258=CARTESIAN_POINT ( 'NONE',  ( -8.982687423579998054, 1383.819621401789846, 218.5044028809089980 ) ) ;
#26265=CARTESIAN_POINT ( 'NONE',  ( -11.39903424189999903, 1388.037600957480208, 201.7885523045490004 ) ) ;
#26294=CARTESIAN_POINT ( 'NONE',  ( -9.129808743239919977, 1383.863787745319996, 218.5279288296370055 ) ) ;
#26300=CARTESIAN_POINT ( 'NONE',  ( -14.49023771376019987, 1379.969971553530058, 208.6314281993359998 ) ) ;
#26304=CARTESIAN_POINT ( 'NONE',  ( -109.0401330529258956, 1382.147805055439449, 310.8429168940339764 ) ) ;
#26305=CARTESIAN_POINT ( 'NONE',  ( -12.31584554800360465, 1377.880485592854939, 209.0191605607812733 ) ) ;
#26307=CARTESIAN_POINT ( 'NONE',  ( -11.67564806959999935, 1391.913060387289988, 208.7639730238099958 ) ) ;
#26308=CARTESIAN_POINT ( 'NONE',  ( -72.68591527607071612, 1385.125501078250181, 271.2577098130889794 ) ) ;
#26326=CARTESIAN_POINT ( 'NONE',  ( -10.25368860849440011, 1391.913060387289988, 204.2726074216130030 ) ) ;
#26347=CARTESIAN_POINT ( 'NONE',  ( -13.93938412159879903, 1379.689544443230034, 208.2922637222520166 ) ) ;
#26373=CARTESIAN_POINT ( 'NONE',  ( -89.02434603483330022, 1384.834799535030015, 291.9443828696540209 ) ) ;
#26390=CARTESIAN_POINT ( 'NONE',  ( -21.11637064600000002, 1379.664572420290142, 209.7302724572810178 ) ) ;
#26407=ORIENTED_EDGE ( 'NONE', *, *, #95293, .F. ) ;
#26413=CARTESIAN_POINT ( 'NONE',  ( -12.26059042640000030, 1378.259319071030177, 207.8536744588589897 ) ) ;
#26439=CARTESIAN_POINT ( 'NONE',  ( -12.23938407635016823, 1377.915032069682411, 210.5017074410068858 ) ) ;
#26444=CARTESIAN_POINT ( 'NONE',  ( -82.57690316193580315, 1384.633320654690124, 305.4287651558460084 ) ) ;
#26446=CARTESIAN_POINT ( 'NONE',  ( -20.72718479384839796, 1384.952021344829973, 201.8520775233429845 ) ) ;
#26452=CARTESIAN_POINT ( 'NONE',  ( -8.370897861499999593, 1384.935302011549993, 199.7749308614990014 ) ) ;
#26462=CARTESIAN_POINT ( 'NONE',  ( -8.297363970850001991, 1383.661068711170174, 199.8123430960490055 ) ) ;
#26476=CARTESIAN_POINT ( 'NONE',  ( -59.63899719916989994, 1379.734822786960194, 264.7657198495529656 ) ) ;
#26482=CARTESIAN_POINT ( 'NONE',  ( -106.9651580870000060, 1379.002928632980002, 308.0502217555589937 ) ) ;
#26498=VERTEX_POINT ( 'NONE', #16745 ) ;
#26510=CARTESIAN_POINT ( 'NONE',  ( -59.04611253552638317, 1379.721492120048424, 259.2250396778080699 ) ) ;
#26545=CARTESIAN_POINT ( 'NONE',  ( -84.12715333319998479, 1385.173288781940073, 288.0594686105589517 ) ) ;
#26567=CARTESIAN_POINT ( 'NONE',  ( -109.8178621839999920, 1385.875214223179910, 297.0872587395590472 ) ) ;
#26581=CARTESIAN_POINT ( 'NONE',  ( -15.36962477406189898, 1384.875951172459963, 219.5140789649539954 ) ) ;
#26604=CARTESIAN_POINT ( 'NONE',  ( -113.4000000000000057, 1376.122490972250034, 306.5935542023590301 ) ) ;
#26612=CARTESIAN_POINT ( 'NONE',  ( -1.658081806242819971E-15, 1375.886883438980021, 209.1218459572589836 ) ) ;
#26626=DIRECTION ( 'NONE',  ( -1.836970198721024757E-16, -1.000000000000000000, -1.001483571081361959E-32 ) ) ;
#26638=CARTESIAN_POINT ( 'NONE',  ( -105.7600638790000005, 1375.390212577269949, 302.0293825393590055 ) ) ;
#26639=CARTESIAN_POINT ( 'NONE',  ( -107.0376884417929944, 1378.913060387299993, 301.1156876987260489 ) ) ;
#26643=CARTESIAN_POINT ( 'NONE',  ( -79.49732243889999950, 1384.913765794120081, 282.9461888724590040 ) ) ;
#26644=CARTESIAN_POINT ( 'NONE',  ( -65.40151035413138914, 1384.707520014439979, 255.9531160123350162 ) ) ;
#26655=CARTESIAN_POINT ( 'NONE',  ( -68.74622153960000048, 1379.747865581630094, 280.1024420339589938 ) ) ;
#26662=CARTESIAN_POINT ( 'NONE',  ( -22.68195036590000058, 1384.853989887049920, 222.0405270882590116 ) ) ;
#26664=CARTESIAN_POINT ( 'NONE',  ( -13.67877973650669965, 1385.299323577030009, 219.1660709978279726 ) ) ;
#26713=CARTESIAN_POINT ( 'NONE',  ( -67.60195043141951032, 1383.787634321580072, 291.9320215662019677 ) ) ;
#26717=CARTESIAN_POINT ( 'NONE',  ( -106.4016663176860078, 1391.913060387289988, 304.1497498221540354 ) ) ;
#26724=CARTESIAN_POINT ( 'NONE',  ( -83.23303318460000355, 1380.073362198620089, 301.6916257618590294 ) ) ;
#26736=CARTESIAN_POINT ( 'NONE',  ( -108.7852627620000021, 1383.811234508949838, 297.2705451043590301 ) ) ;
#26755=CARTESIAN_POINT ( 'NONE',  ( -110.0631843759950499, 1384.903000323588458, 296.9512581633061359 ) ) ;
#26800=CARTESIAN_POINT ( 'NONE',  ( -11.58386370990380065, 1391.913060387200176, 208.1431450511909986 ) ) ;
#26812=CARTESIAN_POINT ( 'NONE',  ( -15.80299171769999944, 1389.615364110129804, 203.8617420411390242 ) ) ;
#26821=EDGE_CURVE ( 'NONE', #8701, #36205, #33201, .T. ) ;
#26823=CARTESIAN_POINT ( 'NONE',  ( -10.31524791190000023, 1382.179600870839977, 217.6122790885089842 ) ) ;
#26846=DIRECTION ( 'NONE',  ( -0.02359658529091402182, 0.000000000000000000, 0.9997215618173935781 ) ) ;
#26863=CARTESIAN_POINT ( 'NONE',  ( -3.078458343110000328, 1380.177950180139987, 203.2132938454989812 ) ) ;
#26870=CARTESIAN_POINT ( 'NONE',  ( -13.66489604771229871, 1390.428739317620057, 209.8137282845850109 ) ) ;
#26880=CARTESIAN_POINT ( 'NONE',  ( -80.37803371308351075, 1385.159040155630009, 283.6058164050980395 ) ) ;
#26882=CARTESIAN_POINT ( 'NONE',  ( -57.93277555979999960, 1379.748264674359916, 257.2455319417590545 ) ) ;
#26893=AXIS2_PLACEMENT_3D ( 'NONE', #42377, #25006, #49700 ) ;
#26904=DIRECTION ( 'NONE',  ( 0.000000000000000000, 0.000000000000000000, -1.000000000000000000 ) ) ;
#26921=CARTESIAN_POINT ( 'NONE',  ( -14.22747554434230111, 1379.717775689809969, 208.2706285310750047 ) ) ;
#26942=CARTESIAN_POINT ( 'NONE',  ( -11.76465091080000036, 1391.913063699309987, 210.9192594439790014 ) ) ;
#26943=CARTESIAN_POINT ( 'NONE',  ( -101.8661395909159921, 1384.880064502870027, 296.5719465711759426 ) ) ;
#26950=VERTEX_POINT ( 'NONE', #77460 ) ;
#26985=ADVANCED_FACE ( 'NONE', ( #17511 ), #1084, .F. ) ;
#26996=CARTESIAN_POINT ( 'NONE',  ( -12.51041414926550033, 1378.851565959029813, 207.9029934983620365 ) ) ;
#27005=DIRECTION ( 'NONE',  ( -6.162707975952100561E-15, -1.000000000000000000, -1.094450614310000083E-14 ) ) ;
#27006=VERTEX_POINT ( 'NONE', #96464 ) ;
#27017=CARTESIAN_POINT ( 'NONE',  ( -77.06261576968471161, 1384.644925923339997, 301.7490929136619684 ) ) ;
#27018=CARTESIAN_POINT ( 'NONE',  ( -22.48406008717340043, 1384.955127046689995, 202.3785104426330008 ) ) ;
#27026=CARTESIAN_POINT ( 'NONE',  ( -7.965791537440000347, 1384.924596536209947, 199.4891613279189926 ) ) ;
#27032=CARTESIAN_POINT ( 'NONE',  ( -106.4289199541310040, 1391.913060387289988, 304.6850071326550164 ) ) ;
#27038=CARTESIAN_POINT ( 'NONE',  ( -9.742013687190000937, 1382.306311483530180, 200.9513237270989805 ) ) ;
#27054=CARTESIAN_POINT ( 'NONE',  ( -66.36191841066799668, 1379.742046394640056, 277.0709747383730246 ) ) ;
#27078=CARTESIAN_POINT ( 'NONE',  ( -5.013435694540000043, 1375.426148861440197, 203.5256706139790310 ) ) ;
#27088=CARTESIAN_POINT ( 'NONE',  ( -50.32639114276440040, 1379.689784808286959, 240.1992801506042099 ) ) ;
#27094=CARTESIAN_POINT ( 'NONE',  ( -104.2285098495619877, 1379.857407253709880, 305.0244821878710013 ) ) ;
#27106=STYLED_ITEM ( 'NONE', ( #16961 ), #89391 ) ;
#27115=CARTESIAN_POINT ( 'NONE',  ( -77.92118381710000108, 1389.362486221770041, 299.0650494567590272 ) ) ;
#27124=CARTESIAN_POINT ( 'NONE',  ( -8.861333410770001251, 1384.870662623919998, 218.6848950059789729 ) ) ;
#27126=CARTESIAN_POINT ( 'NONE',  ( -107.1170720883229990, 1381.212740012770155, 309.4630679377449951 ) ) ;
#27168=DIRECTION ( 'NONE',  ( -1.836970198721029688E-16, -1.000000000000000000, 0.000000000000000000 ) ) ;
#27183=CARTESIAN_POINT ( 'NONE',  ( -110.0628754741750015, 1384.910641149650019, 296.9513051048269858 ) ) ;
#27205=CARTESIAN_POINT ( 'NONE',  ( -73.95609427729999652, 1377.212643071030016, 283.6384370524589826 ) ) ;
#27206=CARTESIAN_POINT ( 'NONE',  ( -106.6936934317039913, 1378.913060387289988, 301.5874337866879955 ) ) ;
#27212=CARTESIAN_POINT ( 'NONE',  ( -94.50571792069999333, 1385.206310935810052, 294.8715553429590273 ) ) ;
#27213=CARTESIAN_POINT ( 'NONE',  ( -66.81431226368310661, 1384.716740919450103, 259.0825501825760284 ) ) ;
#27224=CARTESIAN_POINT ( 'NONE',  ( -68.27348358399999029, 1379.748432006229905, 279.1146441202590722 ) ) ;
#27232=CARTESIAN_POINT ( 'NONE',  ( -54.13602515839999541, 1384.720040384200047, 270.3656545589590223 ) ) ;
#27234=CARTESIAN_POINT ( 'NONE',  ( -11.60595113161150138, 1385.306217073230073, 218.8812244881439995 ) ) ;
#27244=CARTESIAN_POINT ( 'NONE',  ( -5.485381178603089936, 1391.646552095500056, 214.9250346642329816 ) ) ;
#27273=CARTESIAN_POINT ( 'NONE',  ( -91.29898430540859522, 1383.769499161590147, 308.9254833966310230 ) ) ;
#27275=CARTESIAN_POINT ( 'NONE',  ( -109.1111907142439890, 1384.583402408000211, 311.2497943572710142 ) ) ;
#27276=FACE_OUTER_BOUND ( 'NONE', #13396, .T. ) ;
#27281=CARTESIAN_POINT ( 'NONE',  ( -83.50618377039999984, 1381.859495333320183, 288.7003657451589902 ) ) ;
#27282=FACE_BOUND ( 'NONE', #82137, .T. ) ;
#27285=ORIENTED_EDGE ( 'NONE', *, *, #74064, .T. ) ;
#27293=CARTESIAN_POINT ( 'NONE',  ( -107.8906272039999976, 1382.782317645739795, 297.7506189441589868 ) ) ;
#27363=CARTESIAN_POINT ( 'NONE',  ( -1.036208156320000032E-15, 1384.913060387289988, 199.6218459572590120 ) ) ;
#27372=CARTESIAN_POINT ( 'NONE',  ( -8.687735435529999606, 1383.717527281549792, 218.5005275664289854 ) ) ;
#27397=CARTESIAN_POINT ( 'NONE',  ( -25.73187104542529724, 1383.847228980049977, 224.0191246321959682 ) ) ;
#27404=CARTESIAN_POINT ( 'NONE',  ( 12.48894518679548860, 1384.913060387289988, 208.5962528435125591 ) ) ;
#27405=CARTESIAN_POINT ( 'NONE',  ( -8.830847595988496224, 1387.926285407787191, 200.3861648232594348 ) ) ;
#27409=ORIENTED_EDGE ( 'NONE', *, *, #99050, .F. ) ;
#27412=CARTESIAN_POINT ( 'NONE',  ( -14.31906343784990021, 1380.323795378649947, 209.9058136714729983 ) ) ;
#27417=CARTESIAN_POINT ( 'NONE',  ( -12.23669307423070052, 1377.661331666050273, 207.7794331870949804 ) ) ;
#27419=CARTESIAN_POINT ( 'NONE',  ( -10.82437014639999973, 1391.913060387289988, 205.5047960701089949 ) ) ;
#27420=CARTESIAN_POINT ( 'NONE',  ( -87.72787637423360252, 1385.185452115049884, 291.0380262421580255 ) ) ;
#27422=CARTESIAN_POINT ( 'NONE',  ( -65.82430152899999598, 1379.749194687180079, 274.2810710116589803 ) ) ;
#27428=EDGE_LOOP ( 'NONE', ( #101138, #3345, #64341, #88249 ) ) ;
#27458=CARTESIAN_POINT ( 'NONE',  ( -12.35054461905689926, 1378.471275783050260, 209.3240372099530191 ) ) ;
#27466=ORIENTED_EDGE ( 'NONE', *, *, #9792, .T. ) ;
#27487=ADVANCED_FACE ( 'NONE', ( #1731 ), #25933, .T. ) ;
#27501=CARTESIAN_POINT ( 'NONE',  ( -14.16433532520000149, 1379.580334929220044, 207.9040437273089879 ) ) ;
#27539=EDGE_CURVE ( 'NONE', #83109, #33676, #71831, .T. ) ;
#27542=CARTESIAN_POINT ( 'NONE',  ( -13.12582437823970061, 1379.460555358370129, 208.2157137769850124 ) ) ;
#27550=CARTESIAN_POINT ( 'NONE',  ( -7.719966901963539740, 1383.460063487440038, 218.9046041349110112 ) ) ;
#27561=CARTESIAN_POINT ( 'NONE',  ( -74.96511919152730741, 1384.649769891829919, 300.0113357655470168 ) ) ;
#27562=CARTESIAN_POINT ( 'NONE',  ( -9.690554794615099610, 1384.932168088679873, 199.9862972160919981 ) ) ;
#27569=CARTESIAN_POINT ( 'NONE',  ( -8.604130659810000026, 1384.938024752220144, 199.8686491574789841 ) ) ;
#27578=CARTESIAN_POINT ( 'NONE',  ( -7.544890056106759779, 1384.926148859619843, 219.0875905756669795 ) ) ;
#27579=CARTESIAN_POINT ( 'NONE',  ( -9.766491094179999166, 1381.677989206189977, 201.2633182758889916 ) ) ;
#27594=CARTESIAN_POINT ( 'NONE',  ( -65.77537376722109741, 1379.741348619400014, 276.1715386585039482 ) ) ;
#27601=CARTESIAN_POINT ( 'NONE',  ( -109.3080931909999975, 1384.942533863100152, 311.2645480262589786 ) ) ;
#27608=CARTESIAN_POINT ( 'NONE',  ( -105.8549603932629850, 1378.913060387669702, 304.7826772458390110 ) ) ;
#27624=CARTESIAN_POINT ( 'NONE',  ( -7.545074240589999981, 1384.922368660639904, 219.0875752896790232 ) ) ;
#27627=CARTESIAN_POINT ( 'NONE',  ( -35.55178430715702831, 1379.641840282145040, 218.5080530506718048 ) ) ;
#27640=CARTESIAN_POINT ( 'NONE',  ( -37.33274161817728753, 1379.649438190497904, 225.5526503184333365 ) ) ;
#27645=FACE_OUTER_BOUND ( 'NONE', #109617, .T. ) ;
#27659=CARTESIAN_POINT ( 'NONE',  ( -88.55663222859999451, 1388.280866479749875, 293.2112741491590668 ) ) ;
#27672=CARTESIAN_POINT ( 'NONE',  ( -105.3432687185630101, 1381.144191882089899, 308.8504376499449791 ) ) ;
#27699=CARTESIAN_POINT ( 'NONE',  ( -8.862056518773441027, 1384.892951007370129, 218.6851137863439760 ) ) ;
#27721=CARTESIAN_POINT ( 'NONE',  ( -109.5441724399999970, 1379.437034644700134, 304.2217752583950414 ) ) ;
#27722=B_SPLINE_SURFACE_WITH_KNOTS ( 'NONE', 5, 5, ( 
 ( #101675, #93293, #16018, #24965, #16555, #8729, #920, #34498, #85430 ),
 ( #7634, #93828, #7093, #58611, #42909, #77065, #84346, #50745, #375 ),
 ( #41249, #94383, #86001, #43463, #77610, #26638, #50220, #84882, #60834 ),
 ( #94960, #83798, #75421, #109559, #32830, #105019, #27750, #80374, #28310 ),
 ( #78713, #63059, #3136, #88773, #52976, #12056, #97164, #18778, #29394 ),
 ( #1454, #46242, #87107, #62502, #87673, #105579, #36707, #71464, #106118 ),
 ( #53533, #28867, #20434, #61944, #45690, #70901, #19890, #96622, #44564 ),
 ( #2027, #10396, #79275, #37268, #3689, #86551, #96061, #36161, #2585 ),
 ( #54096, #44013, #54641, #95506, #27205, #35596, #37817, #104458, #70346 ),
 ( #72004, #19331, #63595, #88223, #97713, #10962, #52424, #9846, #45133 ),
 ( #69787, #11515, #79829, #78150, #103906, #61388, #30505, #13678, #106658 ),
 ( #81441, #32163, #64694, #21530, #31605, #48989, #55190, #47317, #99901 ),
 ( #29948, #90961, #4752, #73639, #66350, #89864, #4219, #5308, #5870 ),
 ( #38894, #55744, #6418, #73077, #13133, #65783, #91524, #80920, #23198 ),
 ( #64141, #98261, #31055, #46791, #47867, #40563, #22622, #99346, #56825 ),
 ( #48437, #40012, #89315, #82579, #90399, #107217, #39467, #98813, #22075 ),
 ( #57397, #14803, #83121, #74735, #38348, #82002, #65236, #56270, #20985 ),
 ( #12611, #108872, #74192, #107769, #14248, #108321, #72528, #42225, #75831 ),
 ( #60143, #33809, #67448, #76376, #32714, #790, #50087, #34919, #109981 ),
 ( #248, #17539, #23750, #15886, #68548, #100467, #109437, #59585, #84215 ),
 ( #57938, #58483, #83663, #84760, #85307, #102648, #93700, #92070, #7511 ),
 ( #24301, #34375, #94263, #49538, #25948, #6959, #75291, #66896, #8056 ),
 ( #41673, #102114, #92611, #15342, #110525, #16434, #24839, #51741, #85875 ),
 ( #33257, #50626, #9177, #101547, #25393, #59042, #68003, #41113, #16978 ) ),
 .UNSPECIFIED., .F., .F., .F.,
 ( 6, 3, 3, 3, 3, 3, 3, 6 ),
 ( 6, 3, 6 ),
 ( 0.000000000000000000, 19.27951045849999900, 37.56883265599999788, 64.75259520960000259, 97.48063803579999842, 123.9428332119999965, 141.7919792689999952, 160.6499452009999800 ),
 ( 7.853981633970000154, 11.78097245100000023, 15.70796326790000030 ),
 .UNSPECIFIED. ) ;
#27742=EDGE_LOOP ( 'NONE', ( #7322, #10442, #67106, #71748 ) ) ;
#27750=CARTESIAN_POINT ( 'NONE',  ( -101.9210842570000040, 1374.792827289790011, 302.4435101425590346 ) ) ;
#27752=CARTESIAN_POINT ( 'NONE',  ( -105.8811732696050001, 1378.913060387349788, 303.3307478265489863 ) ) ;
#27760=CARTESIAN_POINT ( 'NONE',  ( -9.809994025999090539, 1391.913060387289988, 214.8154631801960193 ) ) ;
#27770=CARTESIAN_POINT ( 'NONE',  ( -66.93998226469999224, 1379.744520212610041, 276.4118626343590108 ) ) ;
#27780=CARTESIAN_POINT ( 'NONE',  ( -19.18216750550000071, 1385.279599344249846, 220.5028985859590023 ) ) ;
#27782=CARTESIAN_POINT ( 'NONE',  ( -113.4000000000000057, 1390.913060387289988, 304.2218459572590064 ) ) ;
#27794=CARTESIAN_POINT ( 'NONE',  ( -5.432410439650000811, 1391.426148861440197, 214.9021618825790085 ) ) ;
#27832=CARTESIAN_POINT ( 'NONE',  ( -78.52563159432189366, 1383.778061994039945, 302.6299618360769728 ) ) ;
#27834=CARTESIAN_POINT ( 'NONE',  ( -109.3672071742060012, 1383.631249172380194, 311.1356417145969999 ) ) ;
#27840=CARTESIAN_POINT ( 'NONE',  ( -70.21063747969999724, 1380.040839330149993, 289.8377882247589810 ) ) ;
#27862=AXIS2_PLACEMENT_3D ( 'NONE', #26612, #84320, #41767 ) ;
#27920=EDGE_CURVE ( 'NONE', #106524, #71158, #41028, .T. ) ;
#27922=CARTESIAN_POINT ( 'NONE',  ( -22.66805973949999853, 1388.284003322340141, 203.4481520923190203 ) ) ;
#27930=CARTESIAN_POINT ( 'NONE',  ( -9.791709161030000885, 1382.673534642720142, 218.0041932793789954 ) ) ;
#27958=CARTESIAN_POINT ( 'NONE',  ( -28.58153792528539583, 1383.843833704670033, 226.4053923691060106 ) ) ;
#27965=CARTESIAN_POINT ( 'NONE',  ( -9.183039342186225085, 1388.489910760221164, 200.7797177079488335 ) ) ;
#27971=CARTESIAN_POINT ( 'NONE',  ( -12.44728924775969858, 1391.409032655050169, 210.6741896695639866 ) ) ;
#27978=CARTESIAN_POINT ( 'NONE',  ( -7.966182304005879899, 1384.912218263729983, 199.4893151478169955 ) ) ;
#27979=CARTESIAN_POINT ( 'NONE',  ( -98.12087982326850977, 1385.216017296190103, 295.8782037632710171 ) ) ;
#27981=CARTESIAN_POINT ( 'NONE',  ( -14.53473304376390018, 1379.710786975620067, 208.2794084638009906 ) ) ;
#28017=ORIENTED_EDGE ( 'NONE', *, *, #65048, .T. ) ;
#28033=CARTESIAN_POINT ( 'NONE',  ( -12.09197207240000083, 1391.856376936869992, 209.7328825797320064 ) ) ;
#28048=CARTESIAN_POINT ( 'NONE',  ( -106.5486053249999969, 1387.898087395329867, 298.3709353731589999 ) ) ;
#28049=CARTESIAN_POINT ( 'NONE',  ( -109.8138132439963499, 1383.469406728881495, 297.1129651261376807 ) ) ;
#28051=CARTESIAN_POINT ( 'NONE',  ( -26.05523246079999922, 1379.607910947010168, 211.4271914385990101 ) ) ;
#28055=CARTESIAN_POINT ( 'NONE',  ( -65.86034991192448729, 1379.747388898481177, 276.1189993386147989 ) ) ;
#28059=ORIENTED_EDGE ( 'NONE', *, *, #73820, .T. ) ;
#28063=CARTESIAN_POINT ( 'NONE',  ( -69.80115760975569117, 1385.024861833069963, 294.8489851850470131 ) ) ;
#28090=CARTESIAN_POINT ( 'NONE',  ( -12.98408369926140082, 1379.322469185889986, 207.9131530563359718 ) ) ;
#28099=CARTESIAN_POINT ( 'NONE',  ( -113.4000000000000057, 1379.913060387289988, 304.2218459572590064 ) ) ;
#28110=CARTESIAN_POINT ( 'NONE',  ( -108.8958719471799981, 1384.583688962449969, 311.2497166588959772 ) ) ;
#28111=CARTESIAN_POINT ( 'NONE',  ( -46.71757468079219677, 1385.008228226510028, 220.5181717465020199 ) ) ;
#28116=CARTESIAN_POINT ( 'NONE',  ( -5.153093391039999638, 1380.759461119849902, 214.7804110970890008 ) ) ;
#28117=CARTESIAN_POINT ( 'NONE',  ( -8.371177922870000288, 1384.930186027270111, 199.7749517192889925 ) ) ;
#28126=CARTESIAN_POINT ( 'NONE',  ( -106.4176595609719982, 1391.913060387289988, 304.5584244006879544 ) ) ;
#28129=CARTESIAN_POINT ( 'NONE',  ( -14.31906343784990021, 1380.323795378649947, 209.9058136714729983 ) ) ;
#28131=CARTESIAN_POINT ( 'NONE',  ( -12.51034971420000019, 1378.851356594869912, 207.9031378654190121 ) ) ;
#28144=CARTESIAN_POINT ( 'NONE',  ( -67.10245500156331389, 1379.743906473960124, 278.1969394921879939 ) ) ;
#28148=ORIENTED_EDGE ( 'NONE', *, *, #84419, .T. ) ;
#28149=CARTESIAN_POINT ( 'NONE',  ( -105.4633178750000013, 1378.947302253090129, 304.0408696983589607 ) ) ;
#28180=CARTESIAN_POINT ( 'NONE',  ( -58.82645245001332768, 1379.720749110920906, 258.7270466031295086 ) ) ;
#28190=CARTESIAN_POINT ( 'NONE',  ( -47.05742503048701764, 1379.681822875473699, 240.2470098597866297 ) ) ;
#28208=CARTESIAN_POINT ( 'NONE',  ( -84.05014466280000818, 1386.741936841920051, 288.1383773578590421 ) ) ;
#28221=CARTESIAN_POINT ( 'NONE',  ( -105.6660805195130024, 1379.161325318640138, 306.4514821997539684 ) ) ;
#28222=ORIENTED_EDGE ( 'NONE', *, *, #64413, .T. ) ;
#28248=CARTESIAN_POINT ( 'NONE',  ( -18.63960087727699744, 1384.866464396289757, 220.4278299832249957 ) ) ;
#28270=B_SPLINE_CURVE_WITH_KNOTS ( 'NONE', 3,
 ( #8518, #100389, #102568, #15794, #75750, #83040, #33175, #109358, #42143, #67366, #42696, #76293, #32084, #6333, #74656, #76851, #84130, #6872, #40482, #49454, #108792, #66272, #59507, #16354, #109895, #41029, #48913, #50552, #84676, #101465, #24752, #23674, #57857, #161 ),
 .UNSPECIFIED., .F., .F.,
 ( 4, 2, 1, 1, 2, 2, 2, 2, 1, 1, 1, 2, 2, 2, 2, 1, 1, 1, 2, 2, 4 ),
 ( 0.000000000000000000, 0.1250000000007119583, 0.1875000000010639267, 0.2187500000012362611, 0.2343750000012936319, 0.2500000000013509749, 0.3750000000019591551, 0.4375000000022347679, 0.4687500000023421265, 0.4843750000024272806, 0.4921875000024374947, 0.4960937500024130697, 0.5000000000023886448, 0.6250000000012784218, 0.6875000000007230883, 0.7187500000004477529, 0.7343750000003123057, 0.7421875000002446932, 0.7460937500002088330, 0.7500000000001729727, 1.000000000000000000 ),
 .UNSPECIFIED. ) ;
#28273=CARTESIAN_POINT ( 'NONE',  ( -83.24330069484520322, 1379.154961504219955, 299.6759861110299994 ) ) ;
#28283=CARTESIAN_POINT ( 'NONE',  ( -8.630315558130000397, 1384.315009893769911, 218.6220459152689841 ) ) ;
#28310=CARTESIAN_POINT ( 'NONE',  ( -101.7780519309999931, 1374.485289779690220, 304.0160546798589962 ) ) ;
#28313=CARTESIAN_POINT ( 'NONE',  ( -106.0964083643799967, 1378.913060387289988, 302.6612236841029926 ) ) ;
#28316=CARTESIAN_POINT ( 'NONE',  ( -98.86909676750001097, 1384.870948519250078, 296.2469157437590184 ) ) ;
#28323=CARTESIAN_POINT ( 'NONE',  ( -3.078458293560000225, 1384.906579013939790, 218.5736861911289850 ) ) ;
#28328=CARTESIAN_POINT ( 'NONE',  ( -67.87070494639999652, 1379.748617063760094, 278.3152404517590526 ) ) ;
#28334=DIRECTION ( 'NONE',  ( -0.03339394388798658936, -0.9993515141380058253, 0.01346832215537827580 ) ) ;
#28336=CARTESIAN_POINT ( 'NONE',  ( -19.17614523219999967, 1385.141607863239869, 220.5180809881589994 ) ) ;
#28338=CARTESIAN_POINT ( 'NONE',  ( -34.66742137116909817, 1385.210832685530022, 233.7091802904559756 ) ) ;
#28360=EDGE_CURVE ( 'NONE', #49801, #47452, #20986, .T. ) ;
#28382=CARTESIAN_POINT ( 'NONE',  ( -86.11627744455289246, 1383.772810929480102, 307.0143598361519821 ) ) ;
#28384=CARTESIAN_POINT ( 'NONE',  ( -109.1783411524900060, 1383.732934801179908, 311.1044898606749598 ) ) ;
#28390=CARTESIAN_POINT ( 'NONE',  ( -74.01743362070000387, 1382.335636213369980, 298.4777005571589825 ) ) ;
#28396=CARTESIAN_POINT ( 'NONE',  ( -109.5349821800000001, 1384.927863536390078, 297.1230985535589753 ) ) ;
#28416=ORIENTED_EDGE ( 'NONE', *, *, #92741, .T. ) ;
#28476=CARTESIAN_POINT ( 'NONE',  ( -30.25680144860000098, 1389.598173243689871, 209.1456520601699935 ) ) ;
#28481=CARTESIAN_POINT ( 'NONE',  ( -14.04578639380744853, 1379.586359795460567, 211.8392331697818634 ) ) ;
#28496=CARTESIAN_POINT ( 'NONE',  ( -12.31067562887320044, 1378.376168525579942, 209.7905782219929733 ) ) ;
#28510=CARTESIAN_POINT ( 'NONE',  ( -27.38624145287259992, 1383.845277887050088, 225.3372244541170062 ) ) ;
#28519=CARTESIAN_POINT ( 'NONE',  ( -3.078458300270000336, 1380.877403101729897, 216.4127659855790284 ) ) ;
#28526=CARTESIAN_POINT ( 'NONE',  ( -9.884511408893031259, 1387.770251651480066, 217.5398018212560203 ) ) ;
#28534=CARTESIAN_POINT ( 'NONE',  ( -7.966104681038361335, 1384.917613660750021, 199.4892774705519969 ) ) ;
#28535=CARTESIAN_POINT ( 'NONE',  ( -105.9580761981150090, 1385.235267633950116, 296.9951120641670173 ) ) ;
#28555=AXIS2_PLACEMENT_3D ( 'NONE', #52651, #10078, #10644 ) ;
#28569=CARTESIAN_POINT ( 'NONE',  ( -12.50000000000000000, 1384.913060387289988, 209.1218459572589836 ) ) ;
#28614=CARTESIAN_POINT ( 'NONE',  ( -61.47253991323098177, 1379.746604392680183, 268.2739652327719000 ) ) ;
#28617=ORIENTED_EDGE ( 'NONE', *, *, #95293, .T. ) ;
#28621=CARTESIAN_POINT ( 'NONE',  ( -75.79396460638429289, 1385.005618079479973, 300.7326138283579553 ) ) ;
#28648=CARTESIAN_POINT ( 'NONE',  ( -12.59362883767730068, 1379.001259401459947, 208.4073637545409952 ) ) ;
#28656=CARTESIAN_POINT ( 'NONE',  ( -7.543897025694540126, 1384.866236297619935, 219.0872343606769732 ) ) ;
#28670=CARTESIAN_POINT ( 'NONE',  ( -98.46962093215799428, 1384.603681201170048, 310.6350572453490031 ) ) ;
#28671=CARTESIAN_POINT ( 'NONE',  ( -48.42360680834229925, 1385.013694626130018, 222.8933081124880005 ) ) ;
#28672=CARTESIAN_POINT ( 'NONE',  ( -5.025617208240078959, 1375.287809068920069, 214.7234685881729774 ) ) ;
#28679=CARTESIAN_POINT ( 'NONE',  ( -8.156361363509999407, 1384.926233631970035, 199.6467913925089874 ) ) ;
#28688=CARTESIAN_POINT ( 'NONE',  ( -106.7343056398989916, 1391.913060387289988, 306.0197523768699739 ) ) ;
#28692=CARTESIAN_POINT ( 'NONE',  ( -12.01638735929999946, 1378.563403400179823, 206.1479454454890003 ) ) ;
#28703=CARTESIAN_POINT ( 'NONE',  ( -68.32997003290930138, 1379.746898581680171, 279.8958236475029935 ) ) ;
#28709=CARTESIAN_POINT ( 'NONE',  ( -109.9853967420000060, 1384.924299815560062, 311.4561928992590083 ) ) ;
#28732=CARTESIAN_POINT ( 'NONE',  ( -12.34367812709999868, 1378.698035246239897, 209.0347064062579818 ) ) ;
#28733=CARTESIAN_POINT ( 'NONE',  ( -63.83653764405461573, 1379.736250008309526, 269.8484324899241642 ) ) ;
#28745=CARTESIAN_POINT ( 'NONE',  ( -56.57320206062674117, 1379.715264457238845, 258.9695720208346756 ) ) ;
#28779=CARTESIAN_POINT ( 'NONE',  ( -105.3217700133209860, 1379.643688862580120, 306.4247263515759983 ) ) ;
#28789=AXIS2_PLACEMENT_3D ( 'NONE', #38242, #62382, #53989 ) ;
#28807=CARTESIAN_POINT ( 'NONE',  ( -27.81979543383449993, 1384.836325904559999, 225.9468839794940038 ) ) ;
#28831=CARTESIAN_POINT ( 'NONE',  ( -52.83507688520099776, 1378.584541267579880, 254.3209184245819756 ) ) ;
#28837=EDGE_LOOP ( 'NONE', ( #12690, #62060, #10562, #96318 ) ) ;
#28842=CARTESIAN_POINT ( 'NONE',  ( -8.873043061549999777, 1384.563416185930009, 218.6696054037190038 ) ) ;
#28867=CARTESIAN_POINT ( 'NONE',  ( -84.75344743939999148, 1379.600296256739966, 297.4377104216590055 ) ) ;
#28869=CARTESIAN_POINT ( 'NONE',  ( -106.3336369974139899, 1378.913060387289988, 302.1715538163180099 ) ) ;
#28883=CARTESIAN_POINT ( 'NONE',  ( -67.25967724030000738, 1379.748837366600128, 277.1187736907589851 ) ) ;
#28889=ORIENTED_EDGE ( 'NONE', *, *, #85128, .F. ) ;
#28890=CARTESIAN_POINT ( 'NONE',  ( -106.6611006919228117, 1391.449730528028113, 300.4457761524841999 ) ) ;
#28892=CARTESIAN_POINT ( 'NONE',  ( -113.4000000000000057, 1384.574445395800012, 311.2057750932590352 ) ) ;
#28895=CARTESIAN_POINT ( 'NONE',  ( -37.05217134432169956, 1385.198326583020162, 237.2200995400409909 ) ) ;
#28944=CARTESIAN_POINT ( 'NONE',  ( -87.30327056457821300, 1383.772041066240035, 307.5216316904810014 ) ) ;
#28945=CARTESIAN_POINT ( 'NONE',  ( -109.0400471772699973, 1383.917152605130013, 311.1276274378030280 ) ) ;
#28949=CARTESIAN_POINT ( 'NONE',  ( -113.4000000000000057, 1382.340570731539856, 310.5600271202590648 ) ) ;
#28954=CARTESIAN_POINT ( 'NONE',  ( -110.0629084960000057, 1384.909053970479818, 296.9513011976590064 ) ) ;
#28990=ADVANCED_FACE ( 'NONE', ( #59714 ), #27722, .F. ) ;
#29031=CARTESIAN_POINT ( 'NONE',  ( -38.63354197089999786, 1386.820476479690115, 239.2314243943589815 ) ) ;
#29055=CARTESIAN_POINT ( 'NONE',  ( -109.3419108030000046, 1385.202749062920020, 297.1491777238589407 ) ) ;
#29068=CARTESIAN_POINT ( 'NONE',  ( -23.46329824210609871, 1383.849819444430068, 222.4997480768529954 ) ) ;
#29075=CARTESIAN_POINT ( 'NONE',  ( -5.973202138170000453, 1382.320070493830144, 217.8378770759090060 ) ) ;
#29081=CARTESIAN_POINT ( 'NONE',  ( -10.51871147594740208, 1389.041396549049978, 216.3808038717850195 ) ) ;
#29088=CARTESIAN_POINT ( 'NONE',  ( -7.966184197910229692, 1384.910162465379926, 199.4893208852380155 ) ) ;
#29089=CARTESIAN_POINT ( 'NONE',  ( -91.21746417506450655, 1385.196499901840070, 293.2697873285799801 ) ) ;
#29162=CARTESIAN_POINT ( 'NONE',  ( -105.9154581355609963, 1391.837543591110034, 304.8725143098620265 ) ) ;
#29163=CARTESIAN_POINT ( 'NONE',  ( -67.60933340036338279, 1379.747570940400010, 278.8523720605941207 ) ) ;
#29169=CARTESIAN_POINT ( 'NONE',  ( -77.05697207116840275, 1385.001984995040175, 301.7532523806860354 ) ) ;
#29172=CARTESIAN_POINT ( 'NONE',  ( -8.888506772567941638, 1385.313486035710184, 218.6606744470870183 ) ) ;
#29175=DIRECTION ( 'NONE',  ( -1.836970198721029688E-16, -1.000000000000000000, 0.000000000000000000 ) ) ;
#29176=VERTEX_POINT ( 'NONE', #51044 ) ;
#29196=CARTESIAN_POINT ( 'NONE',  ( -12.26057121044589948, 1378.259448421470097, 207.8534500484209957 ) ) ;
#29205=CARTESIAN_POINT ( 'NONE',  ( -7.671317258861270361, 1383.657626917639845, 218.9493643440779920 ) ) ;
#29213=B_SPLINE_CURVE_WITH_KNOTS ( 'NONE', 3,
 ( #27699, #87049, #1972, #60210, #102720, #36652, #87618, #26014, #17607, #34988, #19836, #43407, #70849, #51807, #95456, #94329, #35539, #61885, #52917, #85949, #69168, #44509, #104958, #103853, #26581, #77558, #19271, #862, #104405, #18177, #103273, #60778, #86493, #43954, #28248, #52373, #78096, #45079, #10906, #96001, #70294, #18721, #62438, #2529, #61338, #10337, #78656, #36108, #53474, #96564, #79222, #54041, #88170, #56764, #20379, #39401, #47807, #107709, #37759, #30994, #22011, #106602, #21470, #4163, #65170, #3080, #13619, #80312, #56207, #28807, #11458, #107151, #20928, #81943, #5246, #98198, #37208, #72472, #97658, #80862, #55134, #73579, #38290, #99284, #22560, #90339, #89801, #45634, #79774, #88719, #29887, #89254, #71401, #63005, #12550, #81382, #29341, #55680, #12001, #105517, #73015, #64079, #97113, #54584, #46183, #3628, #47258, #13072, #4696, #46729, #71951, #106063, #63542, #38837, #30445, #64630, #98750, #48371, #99841, #84148, #67935, #109377, #75225, #90902, #14741, #83057, #7449, #76312, #6350, #100406, #92544, #100938, #66831, #67385, #32102, #83592, #40498, #24770, #109914, #75766, #32654, #110463, #57337, #6891, #23689, #82514, #108254, #66289, #50016, #108809, #24234, #91463, #50569, #41612, #41047, #101482, #58418, #15812, #74124, #33194, #33740, #58966, #57874, #23132, #102041, #48930, #16371, #74675, #92006, #93099, #5813, #15278, #84695, #25328, #14185, #39952, #65720, #49471, #7994, #42160, #31543, #44944, #94763, #59524, #18039, #36517, #35410, #61745, #104273, #9105, #51671, #68484, #723, #78526, #52232, #103144, #85244, #95321, #8540, #61207, #87485, #86360, #93636, #34302, #86915, #52778, #77963, #1837, #35971, #95867, #18583, #10206, #16916, #103716, #34853, #19133, #51120, #44382, #10772, #69598, #79091, #76869, #27561, #70162, #17470, #182, #2399, #27017, #53337, #1271, #70710, #43273, #104824, #42716, #102585, #43817, #25883, #60083, #77418, #94199, #85808, #69042, #26444, #60639, #9642, #20794, #54451, #62875, #64497, #47129, #11328, #38705, #45500, #73435, #12949, #37618, #98613, #21876, #4035, #19706, #89119, #38163, #72344, #4571, #80173, #54996, #88587, #72881, #81256, #107018, #80727, #30307, #106473, #29758, #63948, #98061, #3490, #56075, #12408, #105382, #96428, #28670, #90202, #89663, #46592, #13486, #21333, #55539, #79642, #47676, #81805, #62301, #96987, #20250, #5106, #53909, #39261, #29219, #28110, #88044, #2944 ),
 .UNSPECIFIED., .F., .F.,
 ( 4, 3, 3, 3, 3, 3, 3, 3, 3, 3, 3, 3, 3, 3, 3, 3, 3, 3, 3, 3, 3, 3, 3, 3, 3, 3, 3, 3, 3, 3, 3, 3, 3, 3, 3, 3, 3, 3, 3, 3, 3, 3, 3, 3, 3, 3, 3, 3, 3, 3, 3, 3, 3, 3, 3, 3, 3, 3, 3, 3, 3, 3, 3, 3, 3, 3, 3, 3, 3, 3, 3, 3, 3, 3, 3, 3, 3, 3, 3, 3, 3, 3, 3, 3, 3, 3, 3, 3, 3, 3, 3, 3, 3, 3, 3, 3, 3, 3, 3, 3, 4 ),
 ( 9.498561704960000185, 10.82581271786099997, 11.98157754783849960, 13.07709420200399997, 14.12652422663150098, 15.12593959681159994, 15.39383910900589925, 16.42924805362760310, 17.50909810246649911, 18.64760857678350092, 19.92915870810679735, 21.39300856659529870, 23.20497190757799899, 24.59301561497350264, 25.84108368276750056, 26.97655774348510249, 27.58084801744849912, 28.68885941005749984, 29.82533532047489899, 30.99492639834819840, 32.20374463193149950, 33.48731841844190171, 34.83172918346869551, 36.25101147155060488, 37.79185539324890897, 39.35626037121420495, 40.84191036018259524, 41.39509552359669442, 43.74764748933439762, 46.15588617650058723, 48.41852181316069448, 50.55859315911320095, 52.47366333285489759, 54.31027375113220046, 56.08354471098009242, 57.80421286508820344, 59.48018875923999360, 61.09911270707588926, 62.69052795272030210, 64.24295526564009151, 65.53909258078100208, 67.16858239626179738, 68.87693503373300530, 70.69370224108921263, 72.67760720951280007, 75.06533303647849209, 77.83954810070869712, 79.89814551137540377, 81.75296411951019593, 83.48762472816490288, 85.13822779119200845, 86.69705361584379943, 88.21559619941889707, 89.68066952009159820, 90.91108773676960197, 92.82807407335819505, 94.79416735270849870, 96.79315978722270586, 98.79695866710609664, 100.7748251777260009, 102.7057122494059911, 104.5720934641509956, 106.3681167381800066, 108.1183885991049891, 109.8272200050709984, 111.4986773274300020, 113.1197408288939954, 114.7157798799740078, 116.2752876061319967, 117.6367619673630003, 119.0756917262879995, 120.5569498931889854, 122.0758578800959810, 123.5880462789450149, 125.0719021203930055, 126.5156553974589997, 127.9164406824140201, 129.2579234214590258, 130.5686603755449937, 131.8387902540730181, 132.4493970714150066, 133.5476357628679978, 134.6466073012290110, 135.7458795129909959, 136.8796545122989983, 137.9777618726589878, 139.0747495574819936, 140.1702608175249907, 141.2639536178200217, 142.3544029523149845, 143.4426570491259838, 144.5274464010880138, 144.8160795074579994, 146.5556413704150032, 148.3807959781919976, 150.2772506426800021, 152.1535931427380035, 153.9584735936539914, 155.6870227822439858, 157.3233957306069897, 157.6324468028149965 ),
 .UNSPECIFIED. ) ;
#29219=CARTESIAN_POINT ( 'NONE',  ( -108.7880151385730017, 1384.583904816670156, 311.2495016965060017 ) ) ;
#29221=CARTESIAN_POINT ( 'NONE',  ( -32.15488896474609248, 1384.972929923339962, 206.8029585035789921 ) ) ;
#29222=CARTESIAN_POINT ( 'NONE',  ( -5.513264357029999729, 1374.913060387289988, 214.9370262455390161 ) ) ;
#29238=CARTESIAN_POINT ( 'NONE',  ( -10.82018256120000110, 1380.538809929369791, 202.7722443582989911 ) ) ;
#29249=CARTESIAN_POINT ( 'NONE',  ( -67.55991329888020402, 1379.745335248140009, 278.8868931239820199 ) ) ;
#29275=CARTESIAN_POINT ( 'NONE',  ( -8.298003019930000335, 1384.922753400079955, 218.7035906743590203 ) ) ;
#29278=CARTESIAN_POINT ( 'NONE',  ( -66.36278826096751970, 1379.742732206253777, 275.1173963032269398 ) ) ;
#29281=CARTESIAN_POINT ( 'NONE',  ( -62.52086756535808831, 1384.688842335020126, 249.5288663568049969 ) ) ;
#29292=DIRECTION ( 'NONE',  ( 0.8775825618903714265, 0.000000000000000000, -0.4794255386042053368 ) ) ;
#29307=CARTESIAN_POINT ( 'NONE',  ( -106.4403080060000093, 1388.016213653540035, 310.4695424982589884 ) ) ;
#29319=CARTESIAN_POINT ( 'NONE',  ( -107.2817012039999867, 1380.464637550900079, 309.2662977502590707 ) ) ;
#29341=CARTESIAN_POINT ( 'NONE',  ( -36.72861643521579822, 1384.801874369770076, 236.7485459430360208 ) ) ;
#29342=AXIS2_PLACEMENT_3D ( 'NONE', #86718, #87847, #29564 ) ;
#29358=CARTESIAN_POINT ( 'NONE',  ( -109.9814841436489985, 1384.590269029640012, 311.4453213042449988 ) ) ;
#29363=CARTESIAN_POINT ( 'NONE',  ( -42.29523164129999202, 1376.793217291669862, 233.4051811251589754 ) ) ;
#29371=LINE ( 'NONE', #55716, #47576 ) ;
#29373=CARTESIAN_POINT ( 'NONE',  ( -8.293045909599999987, 1384.759859680410045, 218.7022228219589977 ) ) ;
#29394=CARTESIAN_POINT ( 'NONE',  ( -94.35247987469999487, 1374.531630663889928, 302.8771378034590498 ) ) ;
#29414=CARTESIAN_POINT ( 'NONE',  ( -67.41494648059999406, 1379.746829620230073, 277.3878582505590202 ) ) ;
#29427=CARTESIAN_POINT ( 'NONE',  ( -27.26703367711199988, 1385.245975695329889, 225.4376821524880086 ) ) ;
#29439=ORIENTED_EDGE ( 'NONE', *, *, #107944, .T. ) ;
#29460=CARTESIAN_POINT ( 'NONE',  ( -105.3886526319999888, 1378.843576906529961, 303.6910441815589934 ) ) ;
#29474=CARTESIAN_POINT ( 'NONE',  ( -94.52376074393620797, 1383.767472540709832, 309.7575467845289836 ) ) ;
#29475=CARTESIAN_POINT ( 'NONE',  ( -109.4169698722499930, 1383.736799322780143, 311.1655289953600345 ) ) ;
#29479=CARTESIAN_POINT ( 'NONE',  ( -109.9987473190000031, 1383.447530301710003, 297.1744276475590141 ) ) ;
#29533=EDGE_CURVE ( 'NONE', #40922, #40014, #45721, .T. ) ;
#29538=CARTESIAN_POINT ( 'NONE',  ( -25.34121475049380123, 1384.545363099709903, 203.4200895163570237 ) ) ;
#29564=DIRECTION ( 'NONE',  ( -1.000000000000000000, 0.000000000000000000, 0.000000000000000000 ) ) ;
#29578=AXIS2_PLACEMENT_3D ( 'NONE', #103707, #9634, #52768 ) ;
#29586=B_SPLINE_SURFACE_WITH_KNOTS ( 'NONE', 5, 5, ( 
 ( #75091, #57197, #21875, #109240, #47675, #5674 ),
 ( #74539, #64496, #83457, #40358, #73981, #107568 ),
 ( #108671, #31961, #30855, #31405, #56074, #30306 ),
 ( #5105, #58281, #100275, #23555, #6752, #66154 ),
 ( #98612, #108111, #40911, #90201, #32524, #92406 ),
 ( #81804, #99700, #39260, #15141, #56628, #15678 ),
 ( #38704, #65030, #22992, #48793, #82915, #57747 ),
 ( #72880, #91867, #49331, #590, #94066, #75641 ),
 ( #9514, #61067, #51529, #43682, #102460, #58828 ) ),
 .UNSPECIFIED., .F., .F., .F.,
 ( 6, 3, 6 ),
 ( 6, 6 ),
 ( 13.44470524419999968, 14.51062177820000088, 15.26427305850000060 ),
 ( 0.000000000000000000, 2.000000000000000000 ),
 .UNSPECIFIED. ) ;
#29588=CARTESIAN_POINT ( 'NONE',  ( -109.7214050949999944, 1385.089256956249983, 297.0893658214590118 ) ) ;
#29598=CARTESIAN_POINT ( 'NONE',  ( -29.19778036811970168, 1383.843077010679963, 226.9952897098220035 ) ) ;
#29599=AXIS2_PLACEMENT_3D ( 'NONE', #37326, #38411, #64759 ) ;
#29609=CARTESIAN_POINT ( 'NONE',  ( -31.82321841959999986, 1383.006323701569954, 206.4748318456290122 ) ) ;
#29616=CARTESIAN_POINT ( 'NONE',  ( -12.06798603031659844, 1389.351698808259925, 215.2113615822289887 ) ) ;
#29625=CARTESIAN_POINT ( 'NONE',  ( -7.966029247037079486, 1384.904051679539862, 199.4892879668419994 ) ) ;
#29626=CARTESIAN_POINT ( 'NONE',  ( -89.54809965716370357, 1385.191320044069926, 292.2920403167919403 ) ) ;
#29649=CARTESIAN_POINT ( 'NONE',  ( -7.770472029140000458, 1385.200197327649903, 218.9075870494289688 ) ) ;
#29676=CARTESIAN_POINT ( 'NONE',  ( -105.0581303879369983, 1379.236400313860031, 304.0328620142400382 ) ) ;
#29679=DIRECTION ( 'NONE',  ( -1.836970198721029688E-16, -1.000000000000000000, 0.000000000000000000 ) ) ;
#29704=CARTESIAN_POINT ( 'NONE',  ( -106.6962466664339928, 1391.913060387289988, 306.0375484597149693 ) ) ;
#29713=CARTESIAN_POINT ( 'NONE',  ( -81.42719599728999924, 1384.990247741029862, 304.7659821400590090 ) ) ;
#29717=ORIENTED_EDGE ( 'NONE', *, *, #24762, .F. ) ;
#29758=CARTESIAN_POINT ( 'NONE',  ( -94.86324456277120021, 1384.610306623129873, 310.0067647644390263 ) ) ;
#29759=CARTESIAN_POINT ( 'NONE',  ( -34.43103305585869833, 1384.977506179140164, 208.2997256558550134 ) ) ;
#29779=CARTESIAN_POINT ( 'NONE',  ( -12.99813084100000005, 1380.049171561279991, 205.3172344645390126 ) ) ;
#29793=CARTESIAN_POINT ( 'NONE',  ( -68.34593601010000441, 1379.747695174430191, 279.8829065415590094 ) ) ;
#29800=CARTESIAN_POINT ( 'NONE',  ( -109.8258757970000090, 1384.928269941609869, 311.3808033402589786 ) ) ;
#29805=CARTESIAN_POINT ( 'NONE',  ( -105.7942887633819993, 1378.913060387289988, 304.0474587704230203 ) ) ;
#29810=DIRECTION ( 'NONE',  ( 1.000000000000000000, 0.000000000000000000, 0.000000000000000000 ) ) ;
#29820=CARTESIAN_POINT ( 'NONE',  ( -8.581591595879999090, 1384.915537926960042, 218.6697260928090145 ) ) ;
#29824=CARTESIAN_POINT ( 'NONE',  ( -67.63483993466537925, 1379.745623042401348, 277.6888451823470518 ) ) ;
#29827=ADVANCED_FACE ( 'NONE', ( #20336 ), #81478, .T. ) ;
#29829=CARTESIAN_POINT ( 'NONE',  ( -56.64330612835929912, 1384.653173750939914, 237.0538881573710057 ) ) ;
#29838=CARTESIAN_POINT ( 'NONE',  ( -108.9547055214669058, 1384.162005982002484, 311.1881122995200144 ) ) ;
#29855=CARTESIAN_POINT ( 'NONE',  ( -113.4000000000000057, 1389.217440337809876, 308.7319511484590180 ) ) ;
#29857=CARTESIAN_POINT ( 'NONE',  ( -9.094739560779999010, 1384.886008049520115, 199.9428817877490019 ) ) ;
#29880=CARTESIAN_POINT ( 'NONE',  ( -12.31997106265569997, 1378.116150552649970, 209.3647867733199917 ) ) ;
#29887=CARTESIAN_POINT ( 'NONE',  ( -34.64930450694949826, 1384.810489686140045, 233.7099306789210118 ) ) ;
#29888=CARTESIAN_POINT ( 'NONE',  ( -105.7943137790000065, 1378.913060387289988, 304.0474592644590075 ) ) ;
#29899=( BOUNDED_CURVE ( )  B_SPLINE_CURVE ( 3, ( #38391, #5347, #20469, #46284 ),
 .UNSPECIFIED., .F., .T. ) 
 B_SPLINE_CURVE_WITH_KNOTS ( ( 4, 4 ),
 ( 6.081914932523700301, 6.202477342412509920 ),
 .UNSPECIFIED. ) 
 CURVE ( )  GEOMETRIC_REPRESENTATION_ITEM ( )  RATIONAL_B_SPLINE_CURVE ( ( 1.000000000000000000, 0.9987890921955699941, 0.9987890921955699941, 1.000000000000000000 ) ) 
 REPRESENTATION_ITEM ( '' )  );
#29910=CARTESIAN_POINT ( 'NONE',  ( -69.40599705544170206, 1377.319800895099888, 286.7245655447559898 ) ) ;
#29914=VERTEX_POINT ( 'NONE', #55081 ) ;
#29923=CARTESIAN_POINT ( 'NONE',  ( -103.5990824459999970, 1389.912137903419989, 305.4537645068589882 ) ) ;
#29944=CARTESIAN_POINT ( 'NONE',  ( -14.49998591057999953, 1379.933159328379816, 208.5575498442950106 ) ) ;
#29948=CARTESIAN_POINT ( 'NONE',  ( -55.15130194409999831, 1379.936376805820146, 253.2598301361589961 ) ) ;
#29962=CARTESIAN_POINT ( 'NONE',  ( -17.48604280480000028, 1384.189952027930076, 219.8991676458590234 ) ) ;
#29966=CARTESIAN_POINT ( 'NONE',  ( -64.02521122240000295, 1379.736828862030052, 270.2693837840589595 ) ) ;
#29975=CARTESIAN_POINT ( 'NONE',  ( -76.09571452209999620, 1384.765849691730182, 301.2247121768590432 ) ) ;
#29977=CARTESIAN_POINT ( 'NONE',  ( -21.52308197379570132, 1385.270236681489905, 221.6137937885669942 ) ) ;
#30001=CARTESIAN_POINT ( 'NONE',  ( -107.9977940029999957, 1389.297716649579797, 298.4487110492589750 ) ) ;
#30003=CARTESIAN_POINT ( 'NONE',  ( -106.5586238660000049, 1390.939237335530152, 300.3883543639590243 ) ) ;
#30024=CARTESIAN_POINT ( 'NONE',  ( -98.44283016700001099, 1380.746464150679913, 298.5816860277590195 ) ) ;
#30030=CARTESIAN_POINT ( 'NONE',  ( -11.28831067177809011, 1378.749259193316448, 204.1390151436862368 ) ) ;
#30064=ORIENTED_EDGE ( 'NONE', *, *, #97224, .F. ) ;
#30080=CARTESIAN_POINT ( 'NONE',  ( -21.59949889905290021, 1384.536962887880009, 202.1273486796540055 ) ) ;
#30123=EDGE_CURVE ( 'NONE', #103478, #52311, #95556, .T. ) ;
#30143=CARTESIAN_POINT ( 'NONE',  ( -38.10078795722100153, 1383.831025482150153, 238.5878336628740044 ) ) ;
#30153=CARTESIAN_POINT ( 'NONE',  ( -19.42552366969999866, 1382.322281656330006, 219.8856874478589987 ) ) ;
#30160=CARTESIAN_POINT ( 'NONE',  ( -8.968339577419470743, 1387.329609371060087, 218.0566458167560029 ) ) ;
#30163=B_SPLINE_CURVE_WITH_KNOTS ( 'NONE', 3,
 ( #93631, #16910, #51115, #85239, #58961, #60078, #110457, #50011, #41042, #8535, #26439, #176, #33734, #102036 ),
 .UNSPECIFIED., .F., .F.,
 ( 4, 2, 2, 2, 2, 2, 4 ),
 ( 0.000000000000000000, 0.2499999999999910072, 0.3749999999999862887, 0.4999999999999815703, 0.6249999999999769074, 0.7499999999999721334, 1.000000000000000000 ),
 .UNSPECIFIED. ) ;
#30181=CARTESIAN_POINT ( 'NONE',  ( -109.1462309409999989, 1385.214558625939844, 311.2612093662589814 ) ) ;
#30191=CARTESIAN_POINT ( 'NONE',  ( -8.296211591059998725, 1385.071719360819998, 218.6997762507590153 ) ) ;
#30214=CARTESIAN_POINT ( 'NONE',  ( -3.078458355219999998, 1384.919541752539999, 199.6700055799090023 ) ) ;
#30255=CARTESIAN_POINT ( 'NONE',  ( -86.03043292017589749, 1384.978873078290235, 307.1765789634189900 ) ) ;
#30258=CARTESIAN_POINT ( 'NONE',  ( -9.236133890019999626, 1386.337655059579902, 200.2251704754490333 ) ) ;
#30306=CARTESIAN_POINT ( 'NONE',  ( -14.26063306530000041, 1380.301850145579920, 210.3217779679890214 ) ) ;
#30307=CARTESIAN_POINT ( 'NONE',  ( -94.05632786852450522, 1384.611781857200185, 309.8312009487510181 ) ) ;
#30308=CARTESIAN_POINT ( 'NONE',  ( -38.90163946207999857, 1384.987285049699949, 211.8655680313669905 ) ) ;
#30316=FACE_OUTER_BOUND ( 'NONE', #79587, .T. ) ;
#30338=CARTESIAN_POINT ( 'NONE',  ( -67.95945271801031140, 1379.746190535669939, 279.4408408362929777 ) ) ;
#30350=CARTESIAN_POINT ( 'NONE',  ( -106.2552881945959911, 1378.913060387629912, 305.9595024995889503 ) ) ;
#30370=CARTESIAN_POINT ( 'NONE',  ( -65.41890721609597392, 1379.740427344783711, 273.1811798692826869 ) ) ;
#30374=CARTESIAN_POINT ( 'NONE',  ( -54.90523341576640348, 1384.643634548589944, 233.6959364829789934 ) ) ;
#30403=CARTESIAN_POINT ( 'NONE',  ( -109.9987472809999929, 1384.922094923150098, 311.2741087182590149 ) ) ;
#30411=CARTESIAN_POINT ( 'NONE',  ( -109.6164617405599984, 1383.195791559909821, 311.2195161898379752 ) ) ;
#30413=ADVANCED_FACE ( 'NONE', ( #13992 ), #22235, .T. ) ;
#30435=CARTESIAN_POINT ( 'NONE',  ( -12.31888632814230000, 1377.996605654810082, 209.2056224712380015 ) ) ;
#30437=ADVANCED_FACE ( 'NONE', ( #81203 ), #41948, .T. ) ;
#30445=CARTESIAN_POINT ( 'NONE',  ( -41.60735100269249642, 1384.780218127079934, 245.0215821269129890 ) ) ;
#30470=CARTESIAN_POINT ( 'NONE',  ( -93.73871268780000321, 1376.241061248600090, 305.1982575765590013 ) ) ;
#30472=CARTESIAN_POINT ( 'NONE',  ( -16.69452037209399720, 1379.657147668529888, 211.9950716805600166 ) ) ;
#30481=CARTESIAN_POINT ( 'NONE',  ( -103.8898877650000117, 1389.939929192370073, 304.1778643809590221 ) ) ;
#30498=CARTESIAN_POINT ( 'NONE',  ( -109.6278266837281308, 1386.599212502288538, 311.2267068848897225 ) ) ;
#30501=CARTESIAN_POINT ( 'NONE',  ( -12.34254106707480148, 1378.948974406790057, 209.4210321092819811 ) ) ;
#30505=CARTESIAN_POINT ( 'NONE',  ( -64.29757574260000297, 1375.128795883580096, 269.4006999320590126 ) ) ;
#30519=CARTESIAN_POINT ( 'NONE',  ( -81.18324780579999356, 1384.635789063720040, 304.9525423562590163 ) ) ;
#30524=CARTESIAN_POINT ( 'NONE',  ( -62.86822150409999921, 1379.735228420929843, 268.0109119421590549 ) ) ;
#30535=CARTESIAN_POINT ( 'NONE',  ( -32.59564481479979747, 1385.221210322680236, 230.9840656712089810 ) ) ;
#30565=CARTESIAN_POINT ( 'NONE',  ( -106.0714421419999951, 1390.773723034939849, 301.0054119742590046 ) ) ;
#30571=CARTESIAN_POINT ( 'NONE',  ( -105.5930518189999958, 1377.934166709269903, 303.6724188547589733 ) ) ;
#30590=CARTESIAN_POINT ( 'NONE',  ( -106.4361662359999912, 1382.339669133240022, 310.6646033542589862 ) ) ;
#30596=DIRECTION ( 'NONE',  ( -1.000000000000000000, 0.000000000000000000, 0.000000000000000000 ) ) ;
#30607=CARTESIAN_POINT ( 'NONE',  ( -107.6675087117007337, 1379.017122048784131, 308.8731021086181840 ) ) ;
#30613=EDGE_LOOP ( 'NONE', ( #93167, #58484, #22329, #96907 ) ) ;
#30624=B_SPLINE_CURVE_WITH_KNOTS ( 'NONE', 3,
 ( #98580, #14013, #15646, #73949, #49852, #22396, #21846, #56596, #92374, #66121, #15111, #83985, #31375, #57166, #75060, #38674, #107536, #100244, #23522, #90170, #83427, #13453, #99668, #106984, #48202, #109209, #22958, #39790, #32493, #5640, #91288, #40880, #64463, #47642 ),
 .UNSPECIFIED., .F., .F.,
 ( 4, 2, 2, 2, 2, 2, 1, 1, 2, 2, 2, 2, 1, 1, 1, 1, 2, 2, 2, 4 ),
 ( 0.000000000000000000, 0.1250000000011176893, 0.1875000000016989743, 0.2500000000022802316, 0.3750000000034041658, 0.4375000000039372949, 0.4687500000041737724, 0.4843750000042577053, 0.4921875000042996717, 0.5000000000043415271, 0.6250000000054165561, 0.6875000000059233729, 0.7187500000061731731, 0.7343750000063343775, 0.7421875000064136474, 0.7460937500064499517, 0.7480468750064269701, 0.7500000000064039885, 0.8750000000032021052, 1.000000000000000000 ),
 .UNSPECIFIED. ) ;
#30632=ORIENTED_EDGE ( 'NONE', *, *, #54520, .T. ) ;
#30646=CARTESIAN_POINT ( 'NONE',  ( -27.67980887459539829, 1384.550718709600005, 204.4238776538969944 ) ) ;
#30658=CIRCLE ( 'NONE', #45007, 3.113774230133182108 ) ;
#30672=CARTESIAN_POINT ( 'NONE',  ( -9.095668477162160315, 1384.718387101820099, 199.9489932286030296 ) ) ;
#30690=CARTESIAN_POINT ( 'NONE',  ( -12.31929927220420140, 1378.277686418020039, 209.5358532329640013 ) ) ;
#30705=CARTESIAN_POINT ( 'NONE',  ( -47.25133509456620118, 1383.816458045290119, 255.6949490582159967 ) ) ;
#30714=CARTESIAN_POINT ( 'NONE',  ( -31.98577773140000247, 1378.974038310059996, 216.6963266813090172 ) ) ;
#30720=CARTESIAN_POINT ( 'NONE',  ( -9.932403141389999135, 1389.845799269120107, 216.5446580629090079 ) ) ;
#30738=CIRCLE ( 'NONE', #105894, 12.26364123839999998 ) ;
#30743=CARTESIAN_POINT ( 'NONE',  ( -109.7531415440000018, 1385.295312989849890, 311.3520341442589938 ) ) ;
#30752=CARTESIAN_POINT ( 'NONE',  ( -8.040000583239999443, 1385.375414080450128, 218.7592922916490181 ) ) ;
#30768=ORIENTED_EDGE ( 'NONE', *, *, #43130, .F. ) ;
#30769=CARTESIAN_POINT ( 'NONE',  ( -108.2039566672529958, 1378.913060387289988, 299.7295690038039879 ) ) ;
#30778=CARTESIAN_POINT ( 'NONE',  ( -105.0454790209999913, 1379.237143502780100, 304.6380415787589868 ) ) ;
#30790=EDGE_LOOP ( 'NONE', ( #23868, #54508, #52927, #102217 ) ) ;
#30803=CARTESIAN_POINT ( 'NONE',  ( -106.2236770203270027, 1391.605574620240077, 306.9900364964820483 ) ) ;
#30811=CARTESIAN_POINT ( 'NONE',  ( -82.20220381884530525, 1384.988272905459780, 305.2249867120139584 ) ) ;
#30812=CARTESIAN_POINT ( 'NONE',  ( -8.837192375920000842, 1385.223969493600180, 199.9173279994789993 ) ) ;
#30815=EDGE_LOOP ( 'NONE', ( #9313, #91178, #107578, #61098, #52563 ) ) ;
#30848=CARTESIAN_POINT ( 'NONE',  ( -106.7685201332123199, 1382.142799015560513, 310.0933617201660013 ) ) ;
#30855=CARTESIAN_POINT ( 'NONE',  ( -12.56073376859999868, 1379.581444859680232, 210.0898675169879937 ) ) ;
#30857=CARTESIAN_POINT ( 'NONE',  ( -64.86877180440029633, 1385.085976455889977, 254.7512439600910170 ) ) ;
#30865=CARTESIAN_POINT ( 'NONE',  ( -109.1315215469999913, 1384.880650352859902, 311.2646143532589917 ) ) ;
#30868=CARTESIAN_POINT ( 'NONE',  ( -109.8097233119999885, 1384.480660791949958, 311.3604857892590303 ) ) ;
#30880=CARTESIAN_POINT ( 'NONE',  ( -5.013264327984152224, 1375.413060387289988, 203.5257471471711312 ) ) ;
#30884=CARTESIAN_POINT ( 'NONE',  ( -109.1649968403673796, 1384.882110519183016, 297.1327717510318394 ) ) ;
#30886=CARTESIAN_POINT ( 'NONE',  ( -68.37438365947571128, 1379.747068193089945, 279.9710327514259802 ) ) ;
#30897=EDGE_CURVE ( 'NONE', #96593, #106524, #43410, .T. ) ;
#30899=CARTESIAN_POINT ( 'NONE',  ( -107.5294434371819818, 1378.913060387289988, 307.8840114082699984 ) ) ;
#30918=CARTESIAN_POINT ( 'NONE',  ( -14.48645815959999794, 1379.659240074840000, 208.2003399408750113 ) ) ;
#30919=CARTESIAN_POINT ( 'NONE',  ( -68.43993043927554254, 1379.747308170265114, 279.3533182895065465 ) ) ;
#30925=CARTESIAN_POINT ( 'NONE',  ( -75.33592628756510123, 1384.769391308340118, 276.0432066516839882 ) ) ;
#30984=CARTESIAN_POINT ( 'NONE',  ( -106.1577607520000015, 1391.913060387289988, 304.2026179676581705 ) ) ;
#30994=CARTESIAN_POINT ( 'NONE',  ( -25.09809013212120377, 1384.845757878930044, 223.7730809620549906 ) ) ;
#30995=CARTESIAN_POINT ( 'NONE',  ( -106.4810267374109998, 1391.913060387289988, 303.2786322724959973 ) ) ;
#30997=FACE_OUTER_BOUND ( 'NONE', #86417, .T. ) ;
#31018=CARTESIAN_POINT ( 'NONE',  ( -39.84051976466280109, 1379.672107560330005, 228.6815457374439973 ) ) ;
#31020=CARTESIAN_POINT ( 'NONE',  ( -19.27348165808830061, 1379.660826776269914, 212.5863292630419892 ) ) ;
#31029=CARTESIAN_POINT ( 'NONE',  ( -8.580669785929998739, 1384.878224714389944, 218.6695462856589813 ) ) ;
#31049=CARTESIAN_POINT ( 'NONE',  ( -13.80262683337540075, 1380.210689512640101, 209.0012437275910315 ) ) ;
#31053=CARTESIAN_POINT ( 'NONE',  ( -4.145978979534980458E-15, 1375.413060387289988, 209.1218459572589836 ) ) ;
#31055=CARTESIAN_POINT ( 'NONE',  ( -45.66666430340000460, 1379.776249196590243, 231.3493056156590058 ) ) ;
#31068=CARTESIAN_POINT ( 'NONE',  ( -38.64161925439999834, 1383.830331748989920, 239.2263113910589993 ) ) ;
#31071=EDGE_CURVE ( 'NONE', #8871, #33676, #21941, .T. ) ;
#31073=CARTESIAN_POINT ( 'NONE',  ( -58.09331443159999964, 1379.714558625850032, 257.1750531167589884 ) ) ;
#31079=CARTESIAN_POINT ( 'NONE',  ( -107.4307047400000101, 1391.913060387289988, 300.8770155100590387 ) ) ;
#31081=( BOUNDED_CURVE ( )  B_SPLINE_CURVE ( 3, ( #54865, #13919, #99031, #88988 ),
 .UNSPECIFIED., .F., .T. ) 
 B_SPLINE_CURVE_WITH_KNOTS ( ( 4, 4 ),
 ( 6.278255371134338070, 6.312181817398001549 ),
 .UNSPECIFIED. ) 
 CURVE ( )  GEOMETRIC_REPRESENTATION_ITEM ( )  RATIONAL_B_SPLINE_CURVE ( ( 1.000000000000000000, 0.9999040853203211565, 0.9999040853203211565, 1.000000000000000000 ) ) 
 REPRESENTATION_ITEM ( '' )  );
#31082=CARTESIAN_POINT ( 'NONE',  ( -113.4000000000000057, 1384.687144183860028, 311.2164849012590366 ) ) ;
#31083=CARTESIAN_POINT ( 'NONE',  ( -46.06193801929999410, 1386.649016502250106, 219.0505733356889948 ) ) ;
#31085=CARTESIAN_POINT ( 'NONE',  ( -48.62444006980110345, 1385.130390675030185, 258.8912542385650113 ) ) ;
#31113=CARTESIAN_POINT ( 'NONE',  ( -107.7385742300000118, 1388.132002054980148, 298.3363211298590159 ) ) ;
#31133=CARTESIAN_POINT ( 'NONE',  ( -102.7832239250000015, 1382.339223999440037, 310.5717497612590137 ) ) ;
#31159=CARTESIAN_POINT ( 'NONE',  ( -5.013321581124261961, 1375.421791045822374, 214.7179703222298883 ) ) ;
#31162=CARTESIAN_POINT ( 'NONE',  ( -9.096737447160000656, 1384.691502115709909, 199.9504659608490158 ) ) ;
#31174=EDGE_CURVE ( 'NONE', #61114, #99409, #110108, .T. ) ;
#31205=CARTESIAN_POINT ( 'NONE',  ( -68.75925446219999060, 1379.747924465840015, 280.1317017307590049 ) ) ;
#31221=CARTESIAN_POINT ( 'NONE',  ( -9.097854467734780570, 1384.691521587119723, 199.9510732930289976 ) ) ;
#31240=CARTESIAN_POINT ( 'NONE',  ( -12.31949146158819985, 1378.253793448930082, 209.5105130821430066 ) ) ;
#31253=CARTESIAN_POINT ( 'NONE',  ( -14.47255314515679991, 1379.648765529259890, 208.1785496007449865 ) ) ;
#31259=CARTESIAN_POINT ( 'NONE',  ( -40.54665132019379570, 1383.827310385500141, 242.7435723248869976 ) ) ;
#31267=CARTESIAN_POINT ( 'NONE',  ( -17.67357672280000003, 1382.321958893279771, 219.3032393030590015 ) ) ;
#31272=PRODUCT ( 'Crank Arm', 'Crank Arm', '', ( #5156 ) ) ;
#31277=CARTESIAN_POINT ( 'NONE',  ( -106.9415904979999965, 1381.793463357829978, 298.5192869564590410 ) ) ;
#31294=CARTESIAN_POINT ( 'NONE',  ( -109.1721745879999901, 1385.500491102209935, 311.2318004082590051 ) ) ;
#31318=CARTESIAN_POINT ( 'NONE',  ( -107.6093135319519973, 1378.913060387369796, 300.4165847144340091 ) ) ;
#31324=CARTESIAN_POINT ( 'NONE',  ( -9.851472566700000044, 1384.510545767029953, 199.8981574268189831 ) ) ;
#31349=CARTESIAN_POINT ( 'NONE',  ( -108.5358826105733812, 1381.246854040435437, 297.9911112566219344 ) ) ;
#31354=CARTESIAN_POINT ( 'NONE',  ( -105.5686611308969987, 1391.210113098429929, 305.6570713065560199 ) ) ;
#31361=CARTESIAN_POINT ( 'NONE',  ( -83.32062985459390347, 1384.985472285010019, 305.8467810391779835 ) ) ;
#31363=CARTESIAN_POINT ( 'NONE',  ( -8.264565553860000691, 1386.032785243389981, 199.7638704706089925 ) ) ;
#31375=CARTESIAN_POINT ( 'NONE',  ( -108.2947392991006978, 1388.907026348439786, 298.1986017272994900 ) ) ;
#31378=CARTESIAN_POINT ( 'NONE',  ( -113.4000000000000057, 1384.926148861439970, 304.2218459572590064 ) ) ;
#31401=CARTESIAN_POINT ( 'NONE',  ( -104.7665161994586072, 1380.738255385528419, 308.0305743392281101 ) ) ;
#31405=CARTESIAN_POINT ( 'NONE',  ( -13.04097860699999956, 1380.055736578640108, 210.2016245823089946 ) ) ;
#31407=CARTESIAN_POINT ( 'NONE',  ( -60.86887317925939556, 1385.065624857220200, 245.8709774141379967 ) ) ;
#31415=CARTESIAN_POINT ( 'NONE',  ( -109.1321491280000089, 1384.869787261709916, 311.2644938432590038 ) ) ;
#31419=CARTESIAN_POINT ( 'NONE',  ( -109.9878849640000027, 1384.810441490199992, 311.4547210892589533 ) ) ;
#31433=CARTESIAN_POINT ( 'NONE',  ( -5.512208796550649659, 1374.913060387289988, 203.3071194642340345 ) ) ;
#31438=CARTESIAN_POINT ( 'NONE',  ( -68.69955443098810122, 1379.747795958880261, 280.2901399885819842 ) ) ;
#31472=CARTESIAN_POINT ( 'NONE',  ( -84.62715972491490390, 1384.816154433129896, 288.3829489245200079 ) ) ;
#31480=LINE ( 'NONE', #99778, #17707 ) ;
#31482=DIRECTION ( 'NONE',  ( 0.000000000000000000, 0.000000000000000000, 1.000000000000000000 ) ) ;
#31497=AXIS2_PLACEMENT_3D ( 'NONE', #90971, #38905, #57410 ) ;
#31508=CARTESIAN_POINT ( 'NONE',  ( -109.6125588903939985, 1383.187010251420133, 311.2171431170959863 ) ) ;
#31529=FACE_BOUND ( 'NONE', #61079, .T. ) ;
#31534=CARTESIAN_POINT ( 'NONE',  ( -105.9134739529999933, 1391.838461175369957, 304.2044424958581885 ) ) ;
#31543=CARTESIAN_POINT ( 'NONE',  ( -59.96123856990180201, 1384.695927338900219, 280.8926189855779967 ) ) ;
#31559=CARTESIAN_POINT ( 'NONE',  ( -14.01565498306790047, 1379.590400379700213, 211.9190739246080284 ) ) ;
#31570=CARTESIAN_POINT ( 'NONE',  ( 8.335345713666398798E-14, 1380.413060386289999, 209.1217751689949864 ) ) ;
#31579=DIRECTION ( 'NONE',  ( 0.9076061524720596685, 1.962993793439040551E-32, -0.4198226673190293412 ) ) ;
#31598=CARTESIAN_POINT ( 'NONE',  ( -109.5723520410060843, 1386.720847671712136, 311.1928145605723444 ) ) ;
#31600=CARTESIAN_POINT ( 'NONE',  ( -13.20215179197749933, 1379.610106626019842, 208.3537467556710112 ) ) ;
#31605=CARTESIAN_POINT ( 'NONE',  ( -60.40574806380000439, 1377.395658627419834, 258.0520616922589738 ) ) ;
#31618=CARTESIAN_POINT ( 'NONE',  ( -27.62991514189999975, 1384.504118323729926, 225.6271822822590138 ) ) ;
#31632=CARTESIAN_POINT ( 'NONE',  ( -27.63867464639999838, 1385.244481134689977, 225.6178332698589770 ) ) ;
#31634=CARTESIAN_POINT ( 'NONE',  ( -54.74390983765479746, 1385.094081698930040, 271.3100142828129719 ) ) ;
#31662=CARTESIAN_POINT ( 'NONE',  ( -108.9824555929999974, 1388.007023282849786, 297.6230262977589973 ) ) ;
#31664=CARTESIAN_POINT ( 'NONE',  ( -106.3970662050000016, 1391.913060387289988, 303.5338388646590033 ) ) ;
#31699=EDGE_CURVE ( 'NONE', #82014, #106524, #94065, .T. ) ;
#31753=CARTESIAN_POINT ( 'NONE',  ( -68.76896737129999337, 1379.747921602020142, 280.1883489107589753 ) ) ;
#31800=AXIS2_PLACEMENT_3D ( 'NONE', #26, #34159, #16229 ) ;
#31810=CARTESIAN_POINT ( 'NONE',  ( -40.79815830855969949, 1383.826919031519992, 243.1918157079990124 ) ) ;
#31819=CARTESIAN_POINT ( 'NONE',  ( -9.333610200140000757, 1378.889285013490280, 208.6192618550260249 ) ) ;
#31821=ORIENTED_EDGE ( 'NONE', *, *, #27539, .T. ) ;
#31823=CARTESIAN_POINT ( 'NONE',  ( -9.071346014019580295, 1385.910705005249838, 218.5589227285099980 ) ) ;
#31826=DIRECTION ( 'NONE',  ( -1.836970198721029688E-16, -1.000000000000000000, 0.000000000000000000 ) ) ;
#31828=CARTESIAN_POINT ( 'NONE',  ( -106.0162444670000070, 1379.399730046070090, 300.9954964968589479 ) ) ;
#31835=EDGE_CURVE ( 'NONE', #26950, #7882, #37948, .T. ) ;
#31847=CARTESIAN_POINT ( 'NONE',  ( -109.0826469409999930, 1385.476187853860210, 311.2341188642590168 ) ) ;
#31877=CARTESIAN_POINT ( 'NONE',  ( -46.08898162120000563, 1384.736188145109963, 219.0284454471089646 ) ) ;
#31909=CARTESIAN_POINT ( 'NONE',  ( -13.59371612979999888, 1379.659895191500027, 212.3998098368589922 ) ) ;
#31915=CARTESIAN_POINT ( 'NONE',  ( -9.082734998440001206, 1385.203252519110038, 199.9450228470490174 ) ) ;
#31954=CARTESIAN_POINT ( 'NONE',  ( -104.2957601855958814, 1380.406565240221653, 307.1919735274812524 ) ) ;
#31961=CARTESIAN_POINT ( 'NONE',  ( -12.31607806409999917, 1378.979632277839983, 209.9715911835569955 ) ) ;
#31963=CARTESIAN_POINT ( 'NONE',  ( -50.69150226891620292, 1385.021539566839920, 226.3387534530459959 ) ) ;
#31964=CARTESIAN_POINT ( 'NONE',  ( -11.18264923832449931, 1391.913060387289988, 212.0534155766569882 ) ) ;
#31977=CARTESIAN_POINT ( 'NONE',  ( -109.1258763339999973, 1384.668900320659986, 311.2567808922589734 ) ) ;
#31995=CARTESIAN_POINT ( 'NONE',  ( -68.62638760068000465, 1379.747582755300073, 280.2329060256320190 ) ) ;
#31998=CARTESIAN_POINT ( 'NONE',  ( -7.896115406091596789, 1382.897682410418156, 218.7445328676782594 ) ) ;
#32025=CARTESIAN_POINT ( 'NONE',  ( -12.31752013540000057, 1377.944433778000075, 209.1218459012849848 ) ) ;
#32029=CARTESIAN_POINT ( 'NONE',  ( -10.67458293690000026, 1390.939237263959967, 215.3172610932390114 ) ) ;
#32030=CARTESIAN_POINT ( 'NONE',  ( -83.57387407986560390, 1384.811398240090057, 287.3271726340860255 ) ) ;
#32068=CARTESIAN_POINT ( 'NONE',  ( -55.15130194409999831, 1379.936376805820146, 253.2598301361589961 ) ) ;
#32084=CARTESIAN_POINT ( 'NONE',  ( -9.179967000164252156, 1389.194332180375795, 217.4405442298740354 ) ) ;
#32088=AXIS2_PLACEMENT_3D ( 'NONE', #41870, #33447, #25044 ) ;
#32093=CARTESIAN_POINT ( 'NONE',  ( -12.31987546767580000, 1378.182896808870055, 209.4394671972719948 ) ) ;
#32102=CARTESIAN_POINT ( 'NONE',  ( -46.75536493990070142, 1384.755724536759772, 255.0759030878719784 ) ) ;
#32103=CARTESIAN_POINT ( 'NONE',  ( -106.5401037502859936, 1391.913060387289988, 302.9983041365559870 ) ) ;
#32120=CARTESIAN_POINT ( 'NONE',  ( -12.81053755176069942, 1379.345370588119977, 211.6929659203159986 ) ) ;
#32132=CARTESIAN_POINT ( 'NONE',  ( -47.95030196609049966, 1379.684879134860012, 241.5716482886410006 ) ) ;
#32157=CARTESIAN_POINT ( 'NONE',  ( -106.9654571391928641, 1390.307193624053525, 308.7685348267781933 ) ) ;
#32163=CARTESIAN_POINT ( 'NONE',  ( -58.56722970770000103, 1379.895658628519868, 258.8926058799589782 ) ) ;
#32175=VERTEX_POINT ( 'NONE', #100622 ) ;
#32178=CARTESIAN_POINT ( 'NONE',  ( -38.54974011449999693, 1384.147589378169869, 239.2788492578590080 ) ) ;
#32191=CARTESIAN_POINT ( 'NONE',  ( -47.38272174249999580, 1385.138016709929843, 256.2741787814589998 ) ) ;
#32193=CARTESIAN_POINT ( 'NONE',  ( -50.04085626606729420, 1385.121777519389980, 261.8108732571790256 ) ) ;
#32222=CARTESIAN_POINT ( 'NONE',  ( -107.0237318669999951, 1390.464738565959806, 299.4840498548589949 ) ) ;
#32251=CARTESIAN_POINT ( 'NONE',  ( -8.862056518773441027, 1384.892951007370129, 218.6851137863439760 ) ) ;
#32271=CARTESIAN_POINT ( 'NONE',  ( -110.0632822187059929, 1384.922692771400079, 296.9512106417570294 ) ) ;
#32300=EDGE_CURVE ( 'NONE', #32175, #33852, #39774, .T. ) ;
#32301=CARTESIAN_POINT ( 'NONE',  ( -34.79440155389130496, 1384.568141483509862, 208.5850534773520053 ) ) ;
#32327=CARTESIAN_POINT ( 'NONE',  ( -13.36039414200000230, 1385.021583142659892, 218.9683482914990122 ) ) ;
#32348=CARTESIAN_POINT ( 'NONE',  ( 10.11243515225062772, 1384.899971913130003, 216.4689601570715638 ) ) ;
#32356=CARTESIAN_POINT ( 'NONE',  ( -110.0636328970000051, 1384.926148861439970, 296.9511395936589793 ) ) ;
#32359=ORIENTED_EDGE ( 'NONE', *, *, #97392, .T. ) ;
#32370=CARTESIAN_POINT ( 'NONE',  ( -45.33985951152630633, 1383.819616475409930, 251.8326084204159940 ) ) ;
#32379=CARTESIAN_POINT ( 'NONE',  ( -39.71502537339999606, 1379.912275921419905, 233.1978909833590023 ) ) ;
#32388=CARTESIAN_POINT ( 'NONE',  ( -105.9513423759999995, 1381.041490069900192, 299.4116665826589951 ) ) ;
#32404=CIRCLE ( 'NONE', #75270, 2.000011244141678635 ) ;
#32409=CARTESIAN_POINT ( 'NONE',  ( -109.3221271740000020, 1385.236114835410035, 311.2661557522589533 ) ) ;
#32420=CARTESIAN_POINT ( 'NONE',  ( -14.36584259495580085, 1379.600156427309912, 208.0333617596500062 ) ) ;
#32430=CARTESIAN_POINT ( 'NONE',  ( -13.82378397995019981, 1379.696997726179916, 208.1617145838290241 ) ) ;
#32440=ORIENTED_EDGE ( 'NONE', *, *, #84635, .T. ) ;
#32442=CARTESIAN_POINT ( 'NONE',  ( -39.76804797110000322, 1384.988983489909742, 212.4493689816489734 ) ) ;
#32461=ORIENTED_EDGE ( 'NONE', *, *, #62348, .T. ) ;
#32475=CARTESIAN_POINT ( 'NONE',  ( -10.76003433109999996, 1379.099935777159772, 215.2151889901689970 ) ) ;
#32482=CARTESIAN_POINT ( 'NONE',  ( -9.868952737369999895, 1387.120338798609964, 200.7479674930190185 ) ) ;
#32488=CARTESIAN_POINT ( 'NONE',  ( -9.128811013672018859, 1383.865584117230128, 218.5284686629279918 ) ) ;
#32493=CARTESIAN_POINT ( 'NONE',  ( -109.4272857735724358, 1387.208746469848847, 297.3473037064583764 ) ) ;
#32512=CARTESIAN_POINT ( 'NONE',  ( -7.956327371650409042, 1385.264409114995033, 199.4928816929445077 ) ) ;
#32515=CARTESIAN_POINT ( 'NONE',  ( -109.3497582309999814, 1384.888520030000109, 297.1386468897590021 ) ) ;
#32519=CARTESIAN_POINT ( 'NONE',  ( -103.6745750688534429, 1379.960313182111804, 305.2256231368813246 ) ) ;
#32524=CARTESIAN_POINT ( 'NONE',  ( -13.57778968770000105, 1380.131028916370269, 210.8119687010990049 ) ) ;
#32526=CARTESIAN_POINT ( 'NONE',  ( -64.59939480701859793, 1385.084584694940077, 254.1492228190850255 ) ) ;
#32537=CARTESIAN_POINT ( 'NONE',  ( -109.8283088200000037, 1384.770372820250032, 311.3782655042589909 ) ) ;
#32544=CARTESIAN_POINT ( 'NONE',  ( -13.88938230474218294, 1379.665440102101456, 212.4764176185094868 ) ) ;
#32554=CARTESIAN_POINT ( 'NONE',  ( -68.69823031144730408, 1379.747764229889981, 280.2920408481639925 ) ) ;
#32584=CARTESIAN_POINT ( 'NONE',  ( -13.82378400310000011, 1379.696997732550017, 208.1617145800939852 ) ) ;
#32589=CARTESIAN_POINT ( 'NONE',  ( -11.84252628229999971, 1391.501155191750058, 212.7918940593590094 ) ) ;
#32590=CARTESIAN_POINT ( 'NONE',  ( -84.89198071708958082, 1384.817327810709912, 288.6329308340300486 ) ) ;
#32654=CARTESIAN_POINT ( 'NONE',  ( -48.91894787223070296, 1384.745253908090035, 259.5132730780889574 ) ) ;
#32655=CARTESIAN_POINT ( 'NONE',  ( -106.8704702527970056, 1391.913060387289988, 302.0021170729179971 ) ) ;
#32661=CARTESIAN_POINT ( 'NONE',  ( -9.574034133352039788, 1380.787723534742099, 201.2514544285035640 ) ) ;
#32680=CARTESIAN_POINT ( 'NONE',  ( -7.543042896288979726, 1380.366160256679905, 209.1217757912289983 ) ) ;
#32682=CARTESIAN_POINT ( 'NONE',  ( -43.42514567895799615, 1379.701639055019996, 233.3025972862479875 ) ) ;
#32689=CARTESIAN_POINT ( 'NONE',  ( -106.0972438490000087, 1378.969065180200005, 306.6607963967590536 ) ) ;
#32711=EDGE_LOOP ( 'NONE', ( #18769, #21114, #39176, #30064 ) ) ;
#32714=CARTESIAN_POINT ( 'NONE',  ( -26.93900968170000354, 1377.750345454750004, 210.6882938058390096 ) ) ;
#32729=CARTESIAN_POINT ( 'NONE',  ( -73.61402272690000359, 1384.068034839990105, 298.8931160141590340 ) ) ;
#32741=CARTESIAN_POINT ( 'NONE',  ( -43.21308294339999634, 1386.785232113230222, 247.4412949693590065 ) ) ;
#32743=CARTESIAN_POINT ( 'NONE',  ( -46.76181045157920124, 1385.141772473130004, 255.0711131765360165 ) ) ;
#32766=CARTESIAN_POINT ( 'NONE',  ( -108.8461099330000081, 1385.969494106900129, 297.2525754554590094 ) ) ;
#32786=CARTESIAN_POINT ( 'NONE',  ( -12.11621817362850351, 1378.266527857301298, 211.6883570102415035 ) ) ;
#32795=CARTESIAN_POINT ( 'NONE',  ( -15.23481017189999953, 1380.318026959200097, 210.0536512759839809 ) ) ;
#32813=CARTESIAN_POINT ( 'NONE',  ( -8.154724234939999761, 1384.732207671340120, 199.6512008194690111 ) ) ;
#32830=CARTESIAN_POINT ( 'NONE',  ( -102.0335792520000098, 1376.985289779790037, 301.2067031052590664 ) ) ;
#32832=CARTESIAN_POINT ( 'NONE',  ( -109.6086345746109885, 1383.178240054900016, 311.2147542219479988 ) ) ;
#32833=CARTESIAN_POINT ( 'NONE',  ( -28.80308794735720213, 1384.553337952709853, 204.9648910289260186 ) ) ;
#32847=CARTESIAN_POINT ( 'NONE',  ( -68.78553819374839406, 1379.747969107289919, 280.2964879544919654 ) ) ;
#32850=DIRECTION ( 'NONE',  ( -0.03508471684983520411, 0.9993076967569471947, -0.01237698856314710383 ) ) ;
#32871=CARTESIAN_POINT ( 'NONE',  ( -8.860943469877430090, 1385.062452151980096, 218.6812855941350051 ) ) ;
#32874=DIRECTION ( 'NONE',  ( 0.000000000000000000, -1.000000000000000000, 0.000000000000000000 ) ) ;
#32897=B_SPLINE_CURVE_WITH_KNOTS ( 'NONE', 3,
 ( #3872, #37999, #63769, #28496, #96812, #19526, #97885, #21159, #12791, #88401, #53161, #35795, #18966, #87302, #10595, #78917, #30690, #82752, #31240 ),
 .UNSPECIFIED., .F., .F.,
 ( 4, 3, 3, 3, 3, 3, 4 ),
 ( -136.9023999274239998, -136.8784091759999910, -136.4141923412300059, -135.9934039197389950, -135.7136470572270071, -135.3701148500000215, -135.0843709324570057 ),
 .UNSPECIFIED. ) ;
#32900=CARTESIAN_POINT ( 'NONE',  ( -59.78493395224469964, 1383.796987562569939, 280.2502008579959920 ) ) ;
#32910=CARTESIAN_POINT ( 'NONE',  ( -73.11457663749999369, 1384.756954744069844, 272.3426209276589702 ) ) ;
#32922=CARTESIAN_POINT ( 'NONE',  ( -105.0999857459999873, 1379.412654380750155, 302.9955102991589797 ) ) ;
#32942=CARTESIAN_POINT ( 'NONE',  ( -105.0227953419999949, 1390.444196973850012, 305.3128289140589686 ) ) ;
#32962=CARTESIAN_POINT ( 'NONE',  ( -14.47191459792289869, 1379.648775954749908, 208.1784578746709826 ) ) ;
#32971=CARTESIAN_POINT ( 'NONE',  ( -31.92192241209999892, 1384.697425913300094, 206.3077903497789691 ) ) ;
#32978=ORIENTED_EDGE ( 'NONE', *, *, #10873, .T. ) ;
#32980=CARTESIAN_POINT ( 'NONE',  ( -11.07039285444999877, 1391.913060387000087, 206.1852823654230065 ) ) ;
#33003=CARTESIAN_POINT ( 'NONE',  ( -12.04121675010000025, 1380.488207265379970, 215.2564011276290046 ) ) ;
#33011=CARTESIAN_POINT ( 'NONE',  ( -11.88252267529999884, 1391.725460676640068, 205.4510509948789831 ) ) ;
#33032=CARTESIAN_POINT ( 'NONE',  ( -14.31392993066779873, 1383.859213631680177, 219.1254165421789821 ) ) ;
#33044=CARTESIAN_POINT ( 'NONE',  ( -7.965680540240001051, 1384.926148861439970, 199.4891222871690104 ) ) ;
#33047=CARTESIAN_POINT ( 'NONE',  ( -109.1655176280000035, 1384.872415562570040, 297.1329087283589843 ) ) ;
#33052=CARTESIAN_POINT ( 'NONE',  ( -103.6828773697239399, 1379.966495660962892, 305.2745416132092942 ) ) ;
#33060=CARTESIAN_POINT ( 'NONE',  ( -78.64707799225199381, 1385.152071352919847, 281.2464940805660376 ) ) ;
#33071=CARTESIAN_POINT ( 'NONE',  ( -109.6459781550000088, 1384.546124173760063, 311.3068487942589968 ) ) ;
#33085=ORIENTED_EDGE ( 'NONE', *, *, #70946, .F. ) ;
#33090=CARTESIAN_POINT ( 'NONE',  ( -68.65906241868358961, 1379.747658069470162, 280.2648999511130228 ) ) ;
#33092=CARTESIAN_POINT ( 'NONE',  ( -9.445418716914016244, 1380.274608993225684, 217.1226397039540075 ) ) ;
#33124=CARTESIAN_POINT ( 'NONE',  ( -76.44953714789230048, 1384.775617543210046, 277.8908186701659702 ) ) ;
#33140=CARTESIAN_POINT ( 'NONE',  ( -63.89205165820000332, 1379.749420737849960, 270.3321189449590065 ) ) ;
#33156=CARTESIAN_POINT ( 'NONE',  ( -8.848600347999999727, 1384.909289574200102, 199.9247552632990050 ) ) ;
#33175=CARTESIAN_POINT ( 'NONE',  ( -9.873265212564325211, 1390.063525629135029, 216.5660449977083317 ) ) ;
#33194=CARTESIAN_POINT ( 'NONE',  ( -53.58244648229940310, 1384.723190384210056, 269.0228002601600110 ) ) ;
#33198=CARTESIAN_POINT ( 'NONE',  ( -107.0293272779999967, 1378.913060310580022, 300.7012236569590300 ) ) ;
#33201=CIRCLE ( 'NONE', #27862, 12.26364123839999998 ) ;
#33203=CARTESIAN_POINT ( 'NONE',  ( -9.752354139992853277, 1380.553637087837387, 201.4862867480141233 ) ) ;
#33209=AXIS2_PLACEMENT_3D ( 'NONE', #86997, #103807, #87570 ) ;
#33223=CARTESIAN_POINT ( 'NONE',  ( -39.19971590621860003, 1377.724600137430116, 229.1242316895250042 ) ) ;
#33226=CARTESIAN_POINT ( 'NONE',  ( -25.97809490251969677, 1379.634779511279930, 215.3796568787460046 ) ) ;
#33232=CARTESIAN_POINT ( 'NONE',  ( -106.6183162539999927, 1379.688366450070134, 308.3260602744589960 ) ) ;
#33234=CARTESIAN_POINT ( 'NONE',  ( -8.321621049119999114, 1385.382011555610006, 218.6716072806289901 ) ) ;
#33248=VERTEX_POINT ( 'NONE', #103962 ) ;
#33257=CARTESIAN_POINT ( 'NONE',  ( 8.345162679097549211E-14, 1380.413060387289988, 209.1218459572589836 ) ) ;
#33263=CARTESIAN_POINT ( 'NONE',  ( -103.5697756572089929, 1379.884498099829898, 304.5397370025139594 ) ) ;
#33282=CARTESIAN_POINT ( 'NONE',  ( -68.75438398539999696, 1390.682777697860047, 280.7419924920590120 ) ) ;
#33284=CARTESIAN_POINT ( 'NONE',  ( -40.89054236768439665, 1385.176891340569910, 243.6910935257890003 ) ) ;
#33292=CARTESIAN_POINT ( 'NONE',  ( -7.769118763749999879, 1384.901714565510019, 218.9178983622890087 ) ) ;
#33294=CARTESIAN_POINT ( 'NONE',  ( -107.7743377200740014, 1382.722932455570117, 310.5776286012699643 ) ) ;
#33306=CARTESIAN_POINT ( 'NONE',  ( -109.8773115550000057, 1385.345135485559922, 297.0432615881589982 ) ) ;
#33339=CARTESIAN_POINT ( 'NONE',  ( -12.30920746619560013, 1378.375653480090023, 209.8169089701579821 ) ) ;
#33380=CARTESIAN_POINT ( 'NONE',  ( -43.99263692700240114, 1384.595883470080025, 217.1388236433490135 ) ) ;
#33387=CARTESIAN_POINT ( 'NONE',  ( -57.81504981494947515, 1379.719253180389387, 261.4703589277106630 ) ) ;
#33392=CARTESIAN_POINT ( 'NONE',  ( -68.33454988889999981, 1379.748399532440089, 279.2380605676589767 ) ) ;
#33401=CARTESIAN_POINT ( 'NONE',  ( -1.253790794730949977E-15, 1385.340268378329938, 218.5931445290690078 ) ) ;
#33445=CARTESIAN_POINT ( 'NONE',  ( -67.95646974556258613, 1383.787266834509865, 292.3773730337559869 ) ) ;
#33446=CARTESIAN_POINT ( 'NONE',  ( -107.4538559658096801, 1379.578066768433700, 299.0810616127055823 ) ) ;
#33447=DIRECTION ( 'NONE',  ( 0.1144950856934970618, -0.9861828161603604093, 0.1197260559028810595 ) ) ;
#33452=CARTESIAN_POINT ( 'NONE',  ( -43.54658723890000260, 1380.341181800959930, 221.0116611961589967 ) ) ;
#33462=CARTESIAN_POINT ( 'NONE',  ( -108.4209992690000064, 1381.081465263680002, 298.0761733255590116 ) ) ;
#33484=CARTESIAN_POINT ( 'NONE',  ( -108.0434378409999994, 1387.272578177979995, 310.5209596992589809 ) ) ;
#33505=ORIENTED_EDGE ( 'NONE', *, *, #9115, .F. ) ;
#33521=CARTESIAN_POINT ( 'NONE',  ( -10.31714591064990039, 1391.913060387289988, 204.4067887391230158 ) ) ;
#33534=CARTESIAN_POINT ( 'NONE',  ( -6.355004503879999156, 1384.926023117790010, 199.7181650675090054 ) ) ;
#33541=CIRCLE ( 'NONE', #97969, 2.500000000000002220 ) ;
#33544=CARTESIAN_POINT ( 'NONE',  ( -12.20251463719999840, 1379.349961885989842, 213.2031273694090032 ) ) ;
#33563=ADVANCED_FACE ( 'NONE', ( #88822 ), #73200, .F. ) ;
#33575=CARTESIAN_POINT ( 'NONE',  ( -16.90947605223539796, 1383.856729902519874, 219.7128039564150015 ) ) ;
#33582=ORIENTED_EDGE ( 'NONE', *, *, #102175, .T. ) ;
#33595=CARTESIAN_POINT ( 'NONE',  ( -108.0762150893491338, 1380.825853547843508, 310.0506996129533377 ) ) ;
#33598=CARTESIAN_POINT ( 'NONE',  ( -12.56636063060000019, 1391.397300678690044, 209.2272092290610033 ) ) ;
#33599=CARTESIAN_POINT ( 'NONE',  ( -74.21234409784548802, 1385.132681138179805, 274.0804497861159916 ) ) ;
#33600=CARTESIAN_POINT ( 'NONE',  ( -11.49366809032010117, 1391.913060387289988, 210.9873680687220201 ) ) ;
#33624=EDGE_CURVE ( 'NONE', #23648, #67802, #30658, .T. ) ;
#33627=AXIS2_PLACEMENT_3D ( 'NONE', #102011, #6857, #42679 ) ;
#33628=CARTESIAN_POINT ( 'NONE',  ( -68.71065145783319394, 1379.747782736039881, 280.3144169757910049 ) ) ;
#33668=CARTESIAN_POINT ( 'NONE',  ( -91.22062739730009184, 1384.843445976460089, 293.2615258250190209 ) ) ;
#33676=VERTEX_POINT ( 'NONE', #97101 ) ;
#33685=CARTESIAN_POINT ( 'NONE',  ( -62.09998818780000818, 1379.733235768160057, 266.3407746977590023 ) ) ;
#33710=PLANE ( 'NONE',  #81923 ) ;
#33734=CARTESIAN_POINT ( 'NONE',  ( -12.27691143406236840, 1378.140212871909853, 210.1884462337374089 ) ) ;
#33740=CARTESIAN_POINT ( 'NONE',  ( -53.77010317427249930, 1384.722329602369882, 269.3966670172729891 ) ) ;
#33741=CARTESIAN_POINT ( 'NONE',  ( -10.89685441944650002, 1384.934403369409893, 200.0946264938700097 ) ) ;
#33748=CARTESIAN_POINT ( 'NONE',  ( -11.62722270852152207, 1378.375229821887842, 205.0204712162364160 ) ) ;
#33772=AXIS2_PLACEMENT_3D ( 'NONE', #96980, #93764, #102716 ) ;
#33773=CARTESIAN_POINT ( 'NONE',  ( -40.76586742162339760, 1379.696137550030016, 229.2042884337240025 ) ) ;
#33779=CARTESIAN_POINT ( 'NONE',  ( -106.3768849420000038, 1379.360965665230196, 307.8405492843589855 ) ) ;
#33780=CARTESIAN_POINT ( 'NONE',  ( -109.8254558940000010, 1384.920634213669928, 311.3807750492590003 ) ) ;
#33809=CARTESIAN_POINT ( 'NONE',  ( -26.01089419480000231, 1380.250345454860053, 212.5061481324489705 ) ) ;
#33839=CARTESIAN_POINT ( 'NONE',  ( -54.22998853240000017, 1386.694956673949946, 270.3205869870589595 ) ) ;
#33840=VERTEX_POINT ( 'NONE', #81518 ) ;
#33841=CARTESIAN_POINT ( 'NONE',  ( -57.27474470154499642, 1385.080142571920078, 276.1243206708509774 ) ) ;
#33852=VERTEX_POINT ( 'NONE', #47941 ) ;
#33865=CARTESIAN_POINT ( 'NONE',  ( -108.9467996200000073, 1386.017383885020081, 297.2678332311589884 ) ) ;
#33872=DIRECTION ( 'NONE',  ( -1.000000000000000000, 0.000000000000000000, 0.000000000000000000 ) ) ;
#33896=CARTESIAN_POINT ( 'NONE',  ( -12.29913530678689959, 1378.337136344450073, 209.9620885240399843 ) ) ;
#33945=CARTESIAN_POINT ( 'NONE',  ( -31.12598708176519935, 1384.558886231360020, 206.2155377277939863 ) ) ;
#33953=CARTESIAN_POINT ( 'NONE',  ( -46.93859675662718445, 1379.681402112373007, 240.0333065786191753 ) ) ;
#33958=CARTESIAN_POINT ( 'NONE',  ( -68.63570658849999973, 1379.747733383370132, 279.8437119496589958 ) ) ;
#33968=DIRECTION ( 'NONE',  ( 1.000000000000000000, 0.000000000000000000, 0.000000000000000000 ) ) ;
#33989=DIRECTION ( 'NONE',  ( -0.02359658529091402182, 0.000000000000000000, 0.9997215618173935781 ) ) ;
#34013=CARTESIAN_POINT ( 'NONE',  ( -57.76806226941249633, 1383.799805416490017, 276.6705433862790073 ) ) ;
#34022=CARTESIAN_POINT ( 'NONE',  ( -32.23247795450000552, 1383.839374993809770, 229.8499276021589992 ) ) ;
#34028=DIRECTION ( 'NONE',  ( -0.02359658529091402182, 0.000000000000000000, 0.9997215618173935781 ) ) ;
#34034=CARTESIAN_POINT ( 'NONE',  ( -109.1500278820000034, 1384.113452266690047, 297.1923599218590084 ) ) ;
#34056=CARTESIAN_POINT ( 'NONE',  ( -106.2645803829999949, 1391.084643298059973, 307.7533666201589426 ) ) ;
#34101=CARTESIAN_POINT ( 'NONE',  ( -109.9849726248329915, 1384.916895159399928, 311.4561123681800154 ) ) ;
#34107=CARTESIAN_POINT ( 'NONE',  ( -16.33302336319999881, 1384.944327755149970, 200.5749513780490076 ) ) ;
#34115=B_SPLINE_CURVE_WITH_KNOTS ( 'NONE', 3,
 ( #81910, #31508, #30411, #41014, #56730, #64600, #24199, #58385, #49438, #108220, #22530, #83560, #92511, #23101, #65689, #5215, #6853, #66258, #108774 ),
 .UNSPECIFIED., .F., .F.,
 ( 4, 3, 3, 3, 3, 3, 4 ),
 ( -6.813843844574179798, -6.758570408419999787, -5.962361183245239893, -5.075104183334910424, -4.429419003180000480, -4.352120018539999968, -4.284224695669999861 ),
 .UNSPECIFIED. ) ;
#34116=CARTESIAN_POINT ( 'NONE',  ( -12.36377300989999917, 1379.230270180880098, 212.7119248548690109 ) ) ;
#34118=ORIENTED_EDGE ( 'NONE', *, *, #50782, .T. ) ;
#34123=CARTESIAN_POINT ( 'NONE',  ( -10.39050546589999868, 1389.480500668439845, 202.2954434700990021 ) ) ;
#34159=DIRECTION ( 'NONE',  ( -1.836970198721029688E-16, -1.000000000000000000, 0.000000000000000000 ) ) ;
#34162=CARTESIAN_POINT ( 'NONE',  ( -11.87131397077319939, 1392.058811529140030, 212.5838674967049826 ) ) ;
#34169=CARTESIAN_POINT ( 'NONE',  ( -11.88051395989999826, 1391.844827726459926, 207.0742441280090134 ) ) ;
#34170=CARTESIAN_POINT ( 'NONE',  ( -81.42081042106549660, 1385.163088500089998, 284.9116589515040232 ) ) ;
#34171=CARTESIAN_POINT ( 'NONE',  ( -11.35261338943339915, 1391.913060387289988, 211.5365630498070004 ) ) ;
#34223=CARTESIAN_POINT ( 'NONE',  ( -14.30929470490690036, 1380.323785527690006, 209.9761919504450134 ) ) ;
#34230=CARTESIAN_POINT ( 'NONE',  ( -10.66758891619999972, 1391.248054696180134, 215.3132018404290022 ) ) ;
#34231=CARTESIAN_POINT ( 'NONE',  ( -99.64292198833310010, 1384.873041396320104, 296.2006670694589729 ) ) ;
#34250=CARTESIAN_POINT ( 'NONE',  ( -14.12491790450000018, 1379.654561017129936, 208.1472458495740057 ) ) ;
#34300=CARTESIAN_POINT ( 'NONE',  ( -10.67458942334280003, 1390.939239166159950, 215.3172498179779666 ) ) ;
#34302=CARTESIAN_POINT ( 'NONE',  ( -67.78736533448140733, 1384.668913691839862, 292.4440920854070214 ) ) ;
#34303=CARTESIAN_POINT ( 'NONE',  ( -16.95405163836110063, 1384.945347557320019, 200.9633990510879755 ) ) ;
#34323=CARTESIAN_POINT ( 'NONE',  ( -12.26989794379589860, 1378.707268951720152, 210.4706525970389919 ) ) ;
#34337=CARTESIAN_POINT ( 'NONE',  ( -63.32122928202920065, 1379.740723965109964, 271.7760642072729524 ) ) ;
#34357=ADVANCED_FACE ( 'NONE', ( #70511 ), #55706, .T. ) ;
#34372=EDGE_CURVE ( 'NONE', #46666, #33840, #76412, .T. ) ;
#34374=CARTESIAN_POINT ( 'NONE',  ( -58.44481929797314734, 1379.719446205599070, 257.8613692807373923 ) ) ;
#34375=CARTESIAN_POINT ( 'NONE',  ( -7.567621161420000853, 1380.366160257679894, 208.3364483334960084 ) ) ;
#34379=CARTESIAN_POINT ( 'NONE',  ( -105.0114562248090095, 1379.360439012370080, 304.5078138772479974 ) ) ;
#34388=CARTESIAN_POINT ( 'NONE',  ( -96.24310955420000369, 1384.607824056739901, 310.5744048422590140 ) ) ;
#34393=EDGE_CURVE ( 'NONE', #29176, #84984, #43107, .T. ) ;
#34400=CARTESIAN_POINT ( 'NONE',  ( -63.53051246150000253, 1388.282315597190063, 254.4959482329590230 ) ) ;
#34402=CARTESIAN_POINT ( 'NONE',  ( -73.70661426834119823, 1385.011922779980068, 298.8812608434159870 ) ) ;
#34412=CARTESIAN_POINT ( 'NONE',  ( -109.3456642170559974, 1383.364683205310030, 311.1052009544930002 ) ) ;
#34413=VERTEX_POINT ( 'NONE', #107377 ) ;
#34439=FACE_OUTER_BOUND ( 'NONE', #40703, .T. ) ;
#34466=CARTESIAN_POINT ( 'NONE',  ( -101.6055713061119974, 1379.039955027740234, 305.9123634697640455 ) ) ;
#34476=CARTESIAN_POINT ( 'NONE',  ( -110.0628542964510075, 1384.912107091729922, 296.9513069434060526 ) ) ;
#34488=DIRECTION ( 'NONE',  ( 1.000000000000000000, 0.000000000000000000, 0.000000000000000000 ) ) ;
#34498=CARTESIAN_POINT ( 'NONE',  ( -113.4000000000000057, 1374.413060387289988, 303.4364477938589744 ) ) ;
#34503=CARTESIAN_POINT ( 'NONE',  ( -48.41198906934850044, 1384.612818244999971, 222.9035708180709889 ) ) ;
#34505=CARTESIAN_POINT ( 'NONE',  ( -108.1428528709999881, 1386.591709523359896, 310.8553624892590506 ) ) ;
#34513=CARTESIAN_POINT ( 'NONE',  ( -68.71730874239999309, 1379.747867717230065, 280.0458894567590278 ) ) ;
#34521=CARTESIAN_POINT ( 'NONE',  ( -22.69270896030000273, 1385.265743060869909, 222.0224438233589979 ) ) ;
#34523=CARTESIAN_POINT ( 'NONE',  ( -15.10282486604810082, 1385.294410954709974, 219.4312743640260237 ) ) ;
#34547=ADVANCED_FACE ( 'NONE', ( #92776 ), #75440, .T. ) ;
#34549=FACE_OUTER_BOUND ( 'NONE', #50511, .T. ) ;
#34556=ORIENTED_EDGE ( 'NONE', *, *, #24049, .T. ) ;
#34567=CARTESIAN_POINT ( 'NONE',  ( -55.19953390322370268, 1383.803617683420043, 271.8223894180929960 ) ) ;
#34574=CARTESIAN_POINT ( 'NONE',  ( -50.19412065850000459, 1382.330029049169980, 260.6313422064590100 ) ) ;
#34586=CARTESIAN_POINT ( 'NONE',  ( -109.9774785470000040, 1383.769209515950024, 297.0228034975589821 ) ) ;
#34609=CARTESIAN_POINT ( 'NONE',  ( -107.6642996119999935, 1387.006294017490063, 310.6297471052590140 ) ) ;
#34618=CARTESIAN_POINT ( 'NONE',  ( -11.74761972249999964, 1388.317445593919956, 202.1816773684589919 ) ) ;
#34630=CARTESIAN_POINT ( 'NONE',  ( -12.31752010984839885, 1377.944433743309901, 209.1218459601290078 ) ) ;
#34659=CARTESIAN_POINT ( 'NONE',  ( -5.959427381639999410, 1385.323914143830052, 218.4985401614089824 ) ) ;
#34668=CARTESIAN_POINT ( 'NONE',  ( -8.399519332060000565, 1383.604135713759888, 218.5402868535989853 ) ) ;
#34674=CARTESIAN_POINT ( 'NONE',  ( -12.37007360149999968, 1392.005019490570021, 208.3240639513470001 ) ) ;
#34680=CARTESIAN_POINT ( 'NONE',  ( -8.860621825987630373, 1384.732557084630116, 218.6806150536880011 ) ) ;
#34711=CARTESIAN_POINT ( 'NONE',  ( -12.11525460871600046, 1391.926222251029913, 211.6230311456439779 ) ) ;
#34715=CARTESIAN_POINT ( 'NONE',  ( -108.9994242794780774, 1382.084811078559824, 310.8140300984987334 ) ) ;
#34718=CARTESIAN_POINT ( 'NONE',  ( -12.40942180589999921, 1391.563918014709998, 208.1819200904450042 ) ) ;
#34720=CARTESIAN_POINT ( 'NONE',  ( -86.96116641772189837, 1385.182907219819754, 290.4451672760540077 ) ) ;
#34761=CARTESIAN_POINT ( 'NONE',  ( -13.51598722900789973, 1379.587471014289804, 208.3760841589739812 ) ) ;
#34766=ORIENTED_EDGE ( 'NONE', *, *, #94757, .F. ) ;
#34774=CARTESIAN_POINT ( 'NONE',  ( -113.4825880485180960, 1378.913060387289988, 307.7208714236177798 ) ) ;
#34784=CARTESIAN_POINT ( 'NONE',  ( -98.60731883373840390, 1384.869673098270141, 295.9819570146710248 ) ) ;
#34801=CARTESIAN_POINT ( 'NONE',  ( -18.87405122379999867, 1379.591274692699926, 208.8065027751330263 ) ) ;
#34824=CARTESIAN_POINT ( 'NONE',  ( -109.7114252020000009, 1385.241546091740020, 297.0985743051589907 ) ) ;
#34853=CARTESIAN_POINT ( 'NONE',  ( -71.67470056025189251, 1384.657983990050070, 296.8765295567630460 ) ) ;
#34854=CARTESIAN_POINT ( 'NONE',  ( -12.32867557342049913, 1384.937034356689992, 200.2425605594509932 ) ) ;
#34872=CARTESIAN_POINT ( 'NONE',  ( -9.529255394169998894, 1383.081092453330029, 200.4708585788389712 ) ) ;
#34873=DIRECTION ( 'NONE',  ( -1.000000000000000000, 0.000000000000000000, 0.000000000000000000 ) ) ;
#34884=CARTESIAN_POINT ( 'NONE',  ( -63.29683978332329986, 1379.736344894609829, 271.7896898339670315 ) ) ;
#34890=CARTESIAN_POINT ( 'NONE',  ( -106.9474174639999973, 1379.784802923450115, 308.7531441963589600 ) ) ;
#34909=ORIENTED_EDGE ( 'NONE', *, *, #54520, .F. ) ;
#34918=CARTESIAN_POINT ( 'NONE',  ( -59.11715075928610474, 1379.721731477463663, 259.3860365151069800 ) ) ;
#34919=CARTESIAN_POINT ( 'NONE',  ( -26.01089419480000231, 1375.250345454859826, 212.5061481324989927 ) ) ;
#34923=CARTESIAN_POINT ( 'NONE',  ( -103.5761608689879978, 1379.883057947149837, 303.9966227597010402 ) ) ;
#34942=DIRECTION ( 'NONE',  ( -1.000000000000000000, 0.000000000000000000, 0.000000000000000000 ) ) ;
#34945=CARTESIAN_POINT ( 'NONE',  ( -102.7967040260000005, 1388.030066489820001, 310.3607065762589627 ) ) ;
#34957=CARTESIAN_POINT ( 'NONE',  ( -108.2374560124399920, 1381.012625538590100, 310.2283385330259762 ) ) ;
#34971=CARTESIAN_POINT ( 'NONE',  ( -109.9639389480000062, 1385.359154056490070, 297.0096814836590511 ) ) ;
#34988=CARTESIAN_POINT ( 'NONE',  ( -11.88161848974299950, 1384.885346608229838, 218.9388788513960264 ) ) ;
#34995=ORIENTED_EDGE ( 'NONE', *, *, #67363, .T. ) ;
#35045=CARTESIAN_POINT ( 'NONE',  ( -105.9558246502879939, 1378.913060387299993, 303.0503163561330098 ) ) ;
#35050=CARTESIAN_POINT ( 'NONE',  ( -46.09131934240000561, 1385.005100670120100, 219.0267588369590044 ) ) ;
#35051=CARTESIAN_POINT ( 'NONE',  ( -53.44135509795150085, 1384.636011670080052, 231.0131721128049662 ) ) ;
#35052=CARTESIAN_POINT ( 'NONE',  ( -14.53473304376390018, 1379.710786975620067, 208.2794084638009906 ) ) ;
#35063=CARTESIAN_POINT ( 'NONE',  ( -68.56795313739999642, 1379.747562649819884, 279.6372059696590213 ) ) ;
#35072=CARTESIAN_POINT ( 'NONE',  ( -43.08084643290000315, 1384.773678278489797, 247.5054735941590138 ) ) ;
#35075=CARTESIAN_POINT ( 'NONE',  ( -9.652326224251600806, 1385.312451791279727, 218.7068224263840079 ) ) ;
#35086=CARTESIAN_POINT ( 'NONE',  ( -8.862914948930789905, 1385.109572092439976, 218.6788282648730046 ) ) ;
#35120=CIRCLE ( 'NONE', #83386, 2.500000000000002220 ) ;
#35121=CARTESIAN_POINT ( 'NONE',  ( -59.44742613381180263, 1383.797447908259983, 279.6660484894090359 ) ) ;
#35128=CARTESIAN_POINT ( 'NONE',  ( -68.60662485189999416, 1380.998604106370067, 291.0269659081590135 ) ) ;
#35139=CARTESIAN_POINT ( 'NONE',  ( -108.6520057740000027, 1383.101129953369991, 297.5200802490589922 ) ) ;
#35144=CARTESIAN_POINT ( 'NONE',  ( -110.0629084955440078, 1384.909053975289908, 296.9513011978259556 ) ) ;
#35153=CARTESIAN_POINT ( 'NONE',  ( -113.4000000000000057, 1390.913060387289988, 304.2218459572590064 ) ) ;
#35212=CARTESIAN_POINT ( 'NONE',  ( -3.078458293700000237, 1385.332091261079995, 218.5458417419390003 ) ) ;
#35223=CARTESIAN_POINT ( 'NONE',  ( -7.769784805680000517, 1383.283764732429972, 218.8591787099389876 ) ) ;
#35230=CARTESIAN_POINT ( 'NONE',  ( -11.41905458360000125, 1390.240470065509953, 203.8447139951190081 ) ) ;
#35237=AXIS2_PLACEMENT_3D ( 'NONE', #48041, #5478, #45991 ) ;
#35246=EDGE_CURVE ( 'NONE', #66491, #46370, #102957, .T. ) ;
#35248=AXIS2_PLACEMENT_3D ( 'NONE', #103162, #85829, #34873 ) ;
#35259=CARTESIAN_POINT ( 'NONE',  ( -9.584235951726055802, 1389.063355496089798, 201.2627618223007744 ) ) ;
#35262=EDGE_LOOP ( 'NONE', ( #29717, #15528, #19442, #101187, #18203, #55302 ) ) ;
#35275=CARTESIAN_POINT ( 'NONE',  ( -11.87927758770000075, 1391.913060425439880, 209.7224555632550107 ) ) ;
#35276=CARTESIAN_POINT ( 'NONE',  ( -85.67243720148771047, 1385.178525901309968, 289.3562383022049858 ) ) ;
#35303=CARTESIAN_POINT ( 'NONE',  ( -120.0391016774570403, 1391.913060387289988, 305.8779575274093077 ) ) ;
#35314=CARTESIAN_POINT ( 'NONE',  ( -13.18655059090340131, 1379.448246895369948, 208.4926571931940202 ) ) ;
#35336=CARTESIAN_POINT ( 'NONE',  ( -92.68261419228250020, 1384.848981413319962, 293.9963934270520554 ) ) ;
#35355=CARTESIAN_POINT ( 'NONE',  ( -14.17772861709999965, 1379.591530681489985, 207.8208986663090059 ) ) ;
#35359=CARTESIAN_POINT ( 'NONE',  ( -68.71629745417266122, 1379.747847503009552, 280.3053889065544126 ) ) ;
#35410=CARTESIAN_POINT ( 'NONE',  ( -61.96637076363960261, 1384.688313717450228, 284.1926743991750186 ) ) ;
#35411=CARTESIAN_POINT ( 'NONE',  ( -24.54314185457210229, 1384.958787300020049, 203.0891551377700068 ) ) ;
#35419=AXIS2_PLACEMENT_3D ( 'NONE', #31053, #57395, #65234 ) ;
#35429=CARTESIAN_POINT ( 'NONE',  ( -9.171139168049998958, 1384.273561242960113, 200.0050165398689899 ) ) ;
#35442=CARTESIAN_POINT ( 'NONE',  ( -65.41331928280889940, 1379.741107854490110, 275.4574184064960036 ) ) ;
#35450=CARTESIAN_POINT ( 'NONE',  ( -7.767752774649999914, 1385.091807982149930, 218.9133695865889990 ) ) ;
#35473=CARTESIAN_POINT ( 'NONE',  ( -32.99886885496665911, 1379.635068102732703, 216.1939695130954249 ) ) ;
#35503=CARTESIAN_POINT ( 'NONE',  ( -89.66056332210000335, 1386.526336894989981, 308.7176818193590293 ) ) ;
#35514=CARTESIAN_POINT ( 'NONE',  ( -108.5976781527699870, 1382.685102817129973, 310.7253367639360704 ) ) ;
#35539=CARTESIAN_POINT ( 'NONE',  ( -13.59805687866929880, 1384.880812014989942, 219.1775672781149922 ) ) ;
#35568=EDGE_CURVE ( 'NONE', #85936, #32175, #10173, .T. ) ;
#35596=CARTESIAN_POINT ( 'NONE',  ( -73.44525057620001007, 1375.641846743739961, 283.9849195986590189 ) ) ;
#35602=CARTESIAN_POINT ( 'NONE',  ( -66.36363792712158727, 1384.713802119680167, 258.0891102980660321 ) ) ;
#35611=CONICAL_SURFACE ( 'NONE', #33772, 7.500000000000000000, 0.02617993877989872875 ) ;
#35612=CARTESIAN_POINT ( 'NONE',  ( -68.36902399430000798, 1379.746974201359990, 279.2217794733590495 ) ) ;
#35620=CARTESIAN_POINT ( 'NONE',  ( -43.07689360599999873, 1384.903938649839802, 247.5074275424589985 ) ) ;
#35622=CARTESIAN_POINT ( 'NONE',  ( -16.85980286139739803, 1385.288128647810026, 219.8538196921649899 ) ) ;
#35670=DIRECTION ( 'NONE',  ( 0.000000000000000000, 0.000000000000000000, -1.000000000000000000 ) ) ;
#35672=CARTESIAN_POINT ( 'NONE',  ( -98.51084969631571653, 1383.764957257319793, 310.4650094518850096 ) ) ;
#35679=CARTESIAN_POINT ( 'NONE',  ( -67.57883611510000321, 1382.334558834929794, 291.7886434181590403 ) ) ;
#35690=CARTESIAN_POINT ( 'NONE',  ( -108.3255562700000070, 1381.229067324740072, 298.1483132478589937 ) ) ;
#35715=EDGE_CURVE ( 'NONE', #98535, #88625, #56178, .T. ) ;
#35724=VERTEX_POINT ( 'NONE', #96108 ) ;
#35771=CARTESIAN_POINT ( 'NONE',  ( -3.078458299170000245, 1388.638918953580060, 216.9987451616589738 ) ) ;
#35781=CARTESIAN_POINT ( 'NONE',  ( -9.129809187350000244, 1383.863787716160004, 218.5279288458490043 ) ) ;
#35795=CARTESIAN_POINT ( 'NONE',  ( -12.31782664275830008, 1378.331050523219801, 209.6139402054469940 ) ) ;
#35812=CARTESIAN_POINT ( 'NONE',  ( -33.61606591832439506, 1383.837376072390043, 232.0323804794959983 ) ) ;
#35815=DIRECTION ( 'NONE',  ( 1.000000000000000000, 0.000000000000000000, 0.000000000000000000 ) ) ;
#35821=CARTESIAN_POINT ( 'NONE',  ( -1.094146225179760032E-15, 1380.165560287059861, 203.1907195691389916 ) ) ;
#35828=DIRECTION ( 'NONE',  ( -0.05651223375311825725, 0.3161865716976207663, -0.9470123649215663741 ) ) ;
#35836=CARTESIAN_POINT ( 'NONE',  ( -11.45492292490000175, 1391.035318004910096, 204.4802647352790075 ) ) ;
#35837=CARTESIAN_POINT ( 'NONE',  ( -90.33759372070990423, 1385.193793571259903, 292.7742252942939558 ) ) ;
#35888=ORIENTED_EDGE ( 'NONE', *, *, #25408, .F. ) ;
#35901=CARTESIAN_POINT ( 'NONE',  ( -99.99820827492719388, 1384.874182120719979, 296.2685436471570029 ) ) ;
#35918=CARTESIAN_POINT ( 'NONE',  ( -18.85193010680000114, 1379.597462637329954, 208.8881565698789871 ) ) ;
#35922=CARTESIAN_POINT ( 'NONE',  ( -68.54407940728098936, 1379.747756885784611, 280.1275194419689001 ) ) ;
#35936=CARTESIAN_POINT ( 'NONE',  ( -7.545020141288169668, 1384.905783179920036, 219.0876432115910006 ) ) ;
#35959=CARTESIAN_POINT ( 'NONE',  ( -7.766930450867759461, 1383.293315432029885, 218.8617756867199944 ) ) ;
#35971=CARTESIAN_POINT ( 'NONE',  ( -69.45404346786109784, 1384.664049648719811, 294.4447972851179429 ) ) ;
#35974=CARTESIAN_POINT ( 'NONE',  ( -5.013264356492538099, 1375.413060387289761, 214.7179447576738482 ) ) ;
#35987=CARTESIAN_POINT ( 'NONE',  ( -106.6249237206099991, 1391.913060387289988, 305.6722210509360025 ) ) ;
#35992=CARTESIAN_POINT ( 'NONE',  ( -10.06558583579999855, 1380.695348830889998, 201.8564714307489680 ) ) ;
#36004=CARTESIAN_POINT ( 'NONE',  ( -66.95006683284590565, 1379.743526258429938, 277.9676770911790413 ) ) ;
#36036=FACE_OUTER_BOUND ( 'NONE', #30790, .T. ) ;
#36041=CARTESIAN_POINT ( 'NONE',  ( -45.68166716313724862, 1379.673069186346083, 231.7062482893097695 ) ) ;
#36053=CARTESIAN_POINT ( 'NONE',  ( -57.65665968917219431, 1379.718748827512627, 261.1525070835933207 ) ) ;
#36070=CARTESIAN_POINT ( 'NONE',  ( -76.73601434870001015, 1388.129781852509950, 300.4664286386590106 ) ) ;
#36078=CIRCLE ( 'NONE', #43191, 3.500000000000003109 ) ;
#36082=CARTESIAN_POINT ( 'NONE',  ( -106.3539583109999995, 1379.482941952589954, 307.8537995074590299 ) ) ;
#36108=CARTESIAN_POINT ( 'NONE',  ( -22.27559603053860116, 1384.855102641009807, 222.0256361789579955 ) ) ;
#36126=CARTESIAN_POINT ( 'NONE',  ( -109.9742488199109971, 1384.497342733709957, 311.4391987445749805 ) ) ;
#36161=CARTESIAN_POINT ( 'NONE',  ( -77.77200720220001529, 1374.656469663290181, 291.9281914796590058 ) ) ;
#36168=CARTESIAN_POINT ( 'NONE',  ( -54.02940655686400362, 1384.639031856270094, 232.0758257302100276 ) ) ;
#36180=CARTESIAN_POINT ( 'NONE',  ( -65.37434784279999178, 1379.739354356529930, 273.2054369558589997 ) ) ;
#36188=CARTESIAN_POINT ( 'NONE',  ( -62.07030651009999644, 1385.055139444880069, 284.7661505247589844 ) ) ;
#36205=VERTEX_POINT ( 'NONE', #75207 ) ;
#36231=CARTESIAN_POINT ( 'NONE',  ( -75.94647945793420263, 1383.780046445180005, 300.6252629312149907 ) ) ;
#36232=CARTESIAN_POINT ( 'NONE',  ( -109.2888349613960060, 1384.560112836649978, 311.2476446514990016 ) ) ;
#36233=CARTESIAN_POINT ( 'NONE',  ( -113.4000000000000057, 1384.913060387289988, 304.2218459572590064 ) ) ;
#36238=CARTESIAN_POINT ( 'NONE',  ( -85.62072771500000101, 1379.320813475580053, 297.8911852074589888 ) ) ;
#36294=ORIENTED_EDGE ( 'NONE', *, *, #104202, .F. ) ;
#36302=CARTESIAN_POINT ( 'NONE',  ( -11.66658784013729999, 1391.913060387289988, 209.7120188154370339 ) ) ;
#36313=CARTESIAN_POINT ( 'NONE',  ( -31.35957567500000209, 1388.283776034970060, 207.2672171163289931 ) ) ;
#36318=CARTESIAN_POINT ( 'NONE',  ( -9.094910673856409389, 1384.931050598509955, 199.9427862989620053 ) ) ;
#36352=CARTESIAN_POINT ( 'NONE',  ( -20.17056002823349914, 1383.853403695010002, 220.8314763200619950 ) ) ;
#36361=CARTESIAN_POINT ( 'NONE',  ( -5.380564766416549850E-17, 1384.485850024879937, 199.6505477045689929 ) ) ;
#36368=CARTESIAN_POINT ( 'NONE',  ( -12.25109094605330107, 1392.007944422769924, 210.6850267857309973 ) ) ;
#36378=CARTESIAN_POINT ( 'NONE',  ( -99.28926058784159636, 1385.219051903349964, 296.1397385972409779 ) ) ;
#36385=EDGE_LOOP ( 'NONE', ( #11917, #21793, #12652, #43343 ) ) ;
#36431=CARTESIAN_POINT ( 'NONE',  ( -11.84966374040000048, 1391.913060387289988, 210.3228853754790180 ) ) ;
#36451=CARTESIAN_POINT ( 'NONE',  ( -42.01596790420000360, 1379.656258535449979, 226.0503548403590059 ) ) ;
#36456=CARTESIAN_POINT ( 'NONE',  ( -65.44977854107980875, 1379.747342584464377, 275.4353169227350691 ) ) ;
#36464=CARTESIAN_POINT ( 'NONE',  ( -68.45946465731660169, 1385.029717728800051, 293.2748923492039808 ) ) ;
#36509=EDGE_CURVE ( 'NONE', #70768, #67802, #72454, .T. ) ;
#36517=CARTESIAN_POINT ( 'NONE',  ( -61.62836627276490020, 1384.689555943140022, 283.6559180833200458 ) ) ;
#36518=CARTESIAN_POINT ( 'NONE',  ( -45.28208375225440818, 1385.003918354740108, 218.6697845988200015 ) ) ;
#36524=CARTESIAN_POINT ( 'NONE',  ( -9.094536456969999350, 1384.945384211949886, 199.9428478864389831 ) ) ;
#36546=CARTESIAN_POINT ( 'NONE',  ( -67.13862316386790496, 1379.745831551899983, 278.1727330697519847 ) ) ;
#36570=EDGE_LOOP ( 'NONE', ( #85162, #21755, #796, #29439, #109141 ) ) ;
#36576=CARTESIAN_POINT ( 'NONE',  ( -8.023209542600000077, 1384.926838732019860, 218.7874811480190260 ) ) ;
#36579=CARTESIAN_POINT ( 'NONE',  ( -59.10074528520486581, 1379.721676241261093, 259.3488587256716187 ) ) ;
#36592=CARTESIAN_POINT ( 'NONE',  ( -57.28860159201197177, 1379.717568064870875, 260.4116547525887881 ) ) ;
#36609=CARTESIAN_POINT ( 'NONE',  ( -92.02227936059999536, 1390.573016258800180, 301.9656767862589959 ) ) ;
#36624=CARTESIAN_POINT ( 'NONE',  ( -105.9692983431669973, 1380.841777212760235, 308.5995165648880629 ) ) ;
#36652=CARTESIAN_POINT ( 'NONE',  ( -10.65556547286379896, 1384.888491042710257, 218.8119669670159908 ) ) ;
#36677=CARTESIAN_POINT ( 'NONE',  ( -113.4000000000000057, 1379.413060386290226, 304.2217751689950092 ) ) ;
#36686=CARTESIAN_POINT ( 'NONE',  ( -107.1062838689999950, 1390.174440383410001, 309.0839720245589888 ) ) ;
#36707=CARTESIAN_POINT ( 'NONE',  ( -88.16707049670000629, 1374.885509058189882, 298.5681932088589861 ) ) ;
#36710=CARTESIAN_POINT ( 'NONE',  ( -106.8013500654249981, 1378.913060387289988, 301.4297679048889904 ) ) ;
#36714=B_SPLINE_SURFACE_WITH_KNOTS ( 'NONE', 5, 5, ( 
 ( #19091, #45452, #79594, #20747, #54944, #10730, #2897, #2352, #44901 ),
 ( #108628, #81757, #108068, #66107, #72838, #40317, #30812, #64449, #31915 ),
 ( #64989, #39777, #5626, #89617, #22946, #74499, #82869, #99107, #48189 ),
 ( #65546, #15098, #31363, #106971, #49290, #98565, #23511, #21834, #73936 ),
 ( #22384, #13440, #90718, #5062, #99655, #100232, #30258, #57704, #56583 ),
 ( #91820, #83418, #14002, #57151, #91276, #12908, #14556, #6714, #6163 ),
 ( #82327, #48746, #40869, #75046, #109198, #56032, #32482, #90159, #66654 ),
 ( #21284, #4529, #55492, #47087, #47630, #81213, #38662, #39209, #73386 ),
 ( #107521, #41436, #50942, #68862, #77792, #67198, #8914, #43089, #26265 ),
 ( #25702, #100756, #34123, #41984, #101296, #43640, #68312, #101858, #76679 ),
 ( #60454, #25151, #1101, #35230, #85614, #58239, #9476, #83972, #110274 ),
 ( #33011, #93463, #24046, #86184, #16196, #92363, #550, #77250, #15636 ),
 ( #24592, #8357, #58785, #94572, #50397, #17845, #59355, #51484, #92924 ),
 ( #84526, #34674, #94025, #42523, #17288, #110830, #16735, #67748, #102421 ),
 ( #85067, #49842, #59904, #7814, #7272, #76133, #102966, #52048, #75602 ) ),
 .UNSPECIFIED., .F., .F., .F.,
 ( 6, 3, 3, 3, 6 ),
 ( 6, 3, 6 ),
 ( 8.074854476129999625, 11.27964861890000137, 15.06487702990000166, 20.05826248609999851, 31.54355322360000002 ),
 ( 0.000000000000000000, 1.000000000000000000, 2.000000000000000000 ),
 .UNSPECIFIED. ) ;
#36715=CARTESIAN_POINT ( 'NONE',  ( -89.15855235860000505, 1384.953912536200050, 292.2553702161590081 ) ) ;
#36722=CARTESIAN_POINT ( 'NONE',  ( -19.17520157370000078, 1384.525909681719895, 220.5202403064590158 ) ) ;
#36727=CARTESIAN_POINT ( 'NONE',  ( -67.28931209470000852, 1379.745217898479950, 277.1039849055590594 ) ) ;
#36736=CARTESIAN_POINT ( 'NONE',  ( -43.08024461549999273, 1385.034280802249896, 247.5058162161589905 ) ) ;
#36738=CARTESIAN_POINT ( 'NONE',  ( -24.35956345089839914, 1385.258544084970026, 223.2439328304530193 ) ) ;
#36740=EDGE_CURVE ( 'NONE', #27006, #43749, #994, .T. ) ;
#36784=CARTESIAN_POINT ( 'NONE',  ( -84.17015566942070848, 1383.774096447810052, 306.0826382659470255 ) ) ;
#36785=CARTESIAN_POINT ( 'NONE',  ( -109.7475505361389878, 1384.114406720439774, 311.3182628089780337 ) ) ;
#36792=CARTESIAN_POINT ( 'NONE',  ( -75.49415276370000072, 1384.770980541030212, 276.6885382114589902 ) ) ;
#36797=CARTESIAN_POINT ( 'NONE',  ( -109.3494501450000058, 1384.931116597319942, 297.1385459540589977 ) ) ;
#36803=B_SPLINE_CURVE_WITH_KNOTS ( 'NONE', 3,
 ( #7277, #67753, #24597, #85620, #76685, #34680, #100763, #110282, #50947, #50405, #86188, #102426, #52053, #41442, #17294, #8920, #109737, #75607, #68868, #25157, #109203, #84531, #40875, #75053, #42531, #32488, #15641, #44312 ),
 .UNSPECIFIED., .F., .F.,
 ( 4, 3, 3, 3, 3, 3, 3, 3, 3, 4 ),
 ( -27.07213034072810132, -26.96001054729109825, -26.59046874310789832, -26.18598420665719928, -25.74274519917580051, -25.56107395287200035, -25.09940057177660222, -24.72598341592859938, -24.42045415469999980, -24.41308947359999948 ),
 .UNSPECIFIED. ) ;
#36815=AXIS2_PLACEMENT_3D ( 'NONE', #91170, #14448, #60910 ) ;
#36858=CARTESIAN_POINT ( 'NONE',  ( -11.62269725585159996, 1391.913060387140149, 208.4322474913049916 ) ) ;
#36868=CARTESIAN_POINT ( 'NONE',  ( -23.42580017550000093, 1388.535583196000061, 220.7761725842590010 ) ) ;
#36893=CARTESIAN_POINT ( 'NONE',  ( -109.7179997069999899, 1385.165587680520048, 297.0932178332590183 ) ) ;
#36904=CARTESIAN_POINT ( 'NONE',  ( -22.97691509383379938, 1383.850362194360059, 222.2151806931460385 ) ) ;
#36913=CARTESIAN_POINT ( 'NONE',  ( -8.350980490578317372, 1386.945100721060726, 199.8923438227050724 ) ) ;
#36919=CARTESIAN_POINT ( 'NONE',  ( -11.37528348128880040, 1389.803332359200112, 215.0420196902499868 ) ) ;
#36923=CARTESIAN_POINT ( 'NONE',  ( -12.31314964446622362, 1377.826519118230408, 208.9131911094586940 ) ) ;
#36926=CARTESIAN_POINT ( 'NONE',  ( -93.07006015126680154, 1385.202033573790004, 294.1823754421509989 ) ) ;
#36927=CARTESIAN_POINT ( 'NONE',  ( -10.08173109987140137, 1391.913060387289988, 214.3435508543619790 ) ) ;
#37000=CARTESIAN_POINT ( 'NONE',  ( -109.1645132478509908, 1384.901512804259937, 297.1326343494729940 ) ) ;
#37014=CARTESIAN_POINT ( 'NONE',  ( -75.37352950217560021, 1385.006855903410042, 300.3767631137689591 ) ) ;
#37066=CARTESIAN_POINT ( 'NONE',  ( -38.18457335657470963, 1384.985636250929929, 211.2360860694770111 ) ) ;
#37067=CARTESIAN_POINT ( 'NONE',  ( -5.013264356663312604, 1375.410824559817684, 214.7179447577057658 ) ) ;
#37072=CARTESIAN_POINT ( 'NONE',  ( -8.371372866679999802, 1384.925069025969833, 199.7749685622990228 ) ) ;
#37078=CARTESIAN_POINT ( 'NONE',  ( -106.5387865765160029, 1391.913060387289988, 305.3438590551860443 ) ) ;
#37082=CARTESIAN_POINT ( 'NONE',  ( -11.59475506509999931, 1379.773093697659988, 204.2227873110190046 ) ) ;
#37096=CARTESIAN_POINT ( 'NONE',  ( -68.28858713622280163, 1379.746781482150027, 279.8552178119970222 ) ) ;
#37104=CARTESIAN_POINT ( 'NONE',  ( -109.8256948709999961, 1384.925724839099757, 311.3807902692590233 ) ) ;
#37128=CARTESIAN_POINT ( 'NONE',  ( -8.023381802619999448, 1384.920841448390092, 218.7875057646990058 ) ) ;
#37130=EDGE_CURVE ( 'NONE', #71158, #59489, #18671, .T. ) ;
#37132=CARTESIAN_POINT ( 'NONE',  ( -68.45463625549879794, 1379.747337658472588, 279.3853496566876515 ) ) ;
#37136=ADVANCED_FACE ( 'NONE', ( #17327 ), #100943, .F. ) ;
#37139=ORIENTED_EDGE ( 'NONE', *, *, #4984, .F. ) ;
#37142=ORIENTED_EDGE ( 'NONE', *, *, #53675, .F. ) ;
#37145=CARTESIAN_POINT ( 'NONE',  ( -58.12963253436136313, 1379.720251017925648, 262.1005719551359334 ) ) ;
#37168=CARTESIAN_POINT ( 'NONE',  ( -91.60491507549998857, 1389.456972387929909, 296.8809262675589480 ) ) ;
#37176=AXIS2_PLACEMENT_3D ( 'NONE', #38009, #46976, #105778 ) ;
#37180=CARTESIAN_POINT ( 'NONE',  ( -105.5548029506649925, 1381.074381071139896, 308.7453718054549654 ) ) ;
#37187=TOROIDAL_SURFACE ( 'NONE', #35419, 8.013264357029999729, 0.5000000000000000000 ) ;
#37195=DIRECTION ( 'NONE',  ( -0.4186104444426561599, -0.02615378819618780631, 0.9077892239757592296 ) ) ;
#37208=CARTESIAN_POINT ( 'NONE',  ( -29.93716070313080024, 1384.828683197690225, 227.9879461525169972 ) ) ;
#37232=CARTESIAN_POINT ( 'NONE',  ( -83.77787960067068695, 1379.600322909919896, 298.8836558466570636 ) ) ;
#37241=CARTESIAN_POINT ( 'NONE',  ( -8.307395124150000143, 1384.509440565790101, 218.6838747432389880 ) ) ;
#37268=CARTESIAN_POINT ( 'NONE',  ( -78.82321740920001218, 1378.727265989730085, 290.9639565884590411 ) ) ;
#37271=CARTESIAN_POINT ( 'NONE',  ( -105.8090605497289971, 1378.913060387299993, 303.7886957086479924 ) ) ;
#37274=CARTESIAN_POINT ( 'NONE',  ( -113.4000000000000057, 1385.026018367459983, 297.2218459572590064 ) ) ;
#37281=CARTESIAN_POINT ( 'NONE',  ( -22.71366063019999970, 1384.180912115839874, 221.9862684950589937 ) ) ;
#37283=CONICAL_SURFACE ( 'NONE', #98089, 7.500000000000000000, 0.02617993877989872875 ) ;
#37287=CARTESIAN_POINT ( 'NONE',  ( -67.30421475440000734, 1379.744441735729879, 277.0965467265589837 ) ) ;
#37298=CARTESIAN_POINT ( 'NONE',  ( -36.42513895959979919, 1385.201677668759885, 236.2565189331969862 ) ) ;
#37312=ORIENTED_EDGE ( 'NONE', *, *, #78217, .T. ) ;
#37326=CARTESIAN_POINT ( 'NONE',  ( -108.6556974451439999, 1383.125878945329987, 312.9723968252589543 ) ) ;
#37341=CARTESIAN_POINT ( 'NONE',  ( -95.02475577813770258, 1383.767157683600090, 309.8628875536620058 ) ) ;
#37342=CARTESIAN_POINT ( 'NONE',  ( -109.4279020612130040, 1384.328769556499765, 311.2418332238150356 ) ) ;
#37346=CARTESIAN_POINT ( 'NONE',  ( -79.44287100420000058, 1383.304495963870067, 282.9878770193590185 ) ) ;
#37351=CARTESIAN_POINT ( 'NONE',  ( -109.1643463520000097, 1384.912499995879898, 297.1325824111589782 ) ) ;
#37377=ADVANCED_FACE ( 'NONE', ( #42427 ), #81443, .F. ) ;
#37393=ORIENTED_EDGE ( 'NONE', *, *, #64413, .F. ) ;
#37412=EDGE_CURVE ( 'NONE', #55324, #48821, #51385, .T. ) ;
#37429=CARTESIAN_POINT ( 'NONE',  ( -43.65213544080000219, 1390.875024450579986, 230.7167253256590129 ) ) ;
#37446=LINE ( 'NONE', #4930, #46037 ) ;
#37452=CARTESIAN_POINT ( 'NONE',  ( -109.3310407770000126, 1385.265527105730143, 297.1549990084589581 ) ) ;
#37463=CARTESIAN_POINT ( 'NONE',  ( -22.73541431592179762, 1383.850630038179816, 222.0790162367429730 ) ) ;
#37471=CARTESIAN_POINT ( 'NONE',  ( -6.354406034210000165, 1384.502204350209922, 199.7451528500290010 ) ) ;
#37478=CARTESIAN_POINT ( 'NONE',  ( -9.233185807659999966, 1388.318973794420117, 217.5719053405290140 ) ) ;
#37486=CARTESIAN_POINT ( 'NONE',  ( -7.966153717961919511, 1384.908122895999895, 199.4893165508340189 ) ) ;
#37487=CARTESIAN_POINT ( 'NONE',  ( -88.24164336956870613, 1385.187133139050275, 291.4137164603869792 ) ) ;
#37506=CARTESIAN_POINT ( 'NONE',  ( -8.594535950999999230, 1385.265555896049818, 218.6506679551489754 ) ) ;
#37513=ADVANCED_FACE ( 'NONE', ( #81001 ), #109010, .F. ) ;
#37553=CARTESIAN_POINT ( 'NONE',  ( -103.5801209296959939, 1379.883073482990085, 303.9981235976169955 ) ) ;
#37565=CARTESIAN_POINT ( 'NONE',  ( -54.44063311572099906, 1379.743533639908492, 254.0790799865290239 ) ) ;
#37572=CARTESIAN_POINT ( 'NONE',  ( -60.96689588341559585, 1385.061429299729980, 282.5775017028749971 ) ) ;
#37618=CARTESIAN_POINT ( 'NONE',  ( -87.62118790240700150, 1384.623622514330009, 307.8351744068140192 ) ) ;
#37619=CARTESIAN_POINT ( 'NONE',  ( -39.59907641771560094, 1384.988928994350090, 212.5044586702960032 ) ) ;
#37620=CARTESIAN_POINT ( 'NONE',  ( -5.473267998913230237, 1374.913303669990000, 214.9198275724610028 ) ) ;
#37625=CARTESIAN_POINT ( 'NONE',  ( -8.156119896610000808, 1384.930225391789918, 199.6467426484390160 ) ) ;
#37633=CARTESIAN_POINT ( 'NONE',  ( -106.4903149258919939, 1391.913060387289988, 305.1044923263290229 ) ) ;
#37650=CARTESIAN_POINT ( 'NONE',  ( -68.44382096765579604, 1379.747259237049775, 280.0252539470139936 ) ) ;
#37656=CARTESIAN_POINT ( 'NONE',  ( -109.9855944279999989, 1384.926148861439970, 311.4562326602589906 ) ) ;
#37669=ORIENTED_EDGE ( 'NONE', *, *, #42486, .F. ) ;
#37682=CARTESIAN_POINT ( 'NONE',  ( -68.13057759640398103, 1379.746676104469316, 278.6999125972471347 ) ) ;
#37695=CARTESIAN_POINT ( 'NONE',  ( -109.0938067140002232, 1384.498046937599838, 311.2419503292331342 ) ) ;
#37702=CARTESIAN_POINT ( 'NONE',  ( 2.140036995326180090E-16, 1390.913060387289988, 209.1218459572589836 ) ) ;
#37704=EDGE_CURVE ( 'NONE', #61557, #51642, #54669, .T. ) ;
#37714=CARTESIAN_POINT ( 'NONE',  ( -109.9987472970000084, 1390.510529229799886, 304.4717760960590454 ) ) ;
#37726=CARTESIAN_POINT ( 'NONE',  ( -105.6827308188049983, 1379.955630914150106, 307.3343922173510236 ) ) ;
#37737=CIRCLE ( 'NONE', #62794, 1.999997933727205579 ) ;
#37759=CARTESIAN_POINT ( 'NONE',  ( -24.84597174231020134, 1384.846610513310225, 223.5967099743799906 ) ) ;
#37768=ORIENTED_EDGE ( 'NONE', *, *, #17950, .T. ) ;
#37784=CARTESIAN_POINT ( 'NONE',  ( -69.65452950130000431, 1376.422073654990072, 286.5559970480589982 ) ) ;
#37794=CARTESIAN_POINT ( 'NONE',  ( -7.764758114139999279, 1384.743521014100224, 218.9160524088590023 ) ) ;
#37817=CARTESIAN_POINT ( 'NONE',  ( -72.92954128540000625, 1375.020180580649821, 284.3347022688589618 ) ) ;
#37823=CARTESIAN_POINT ( 'NONE',  ( -109.9987473190000031, 1385.131185875960000, 297.1742054003590283 ) ) ;
#37829=CARTESIAN_POINT ( 'NONE',  ( -19.19648987400000095, 1384.187074975920041, 220.4662455178590221 ) ) ;
#37832=CIRCLE ( 'NONE', #100401, 12.49965726619999984 ) ;
#37835=CARTESIAN_POINT ( 'NONE',  ( -65.02291513639998755, 1379.744055000310027, 272.5993806172590439 ) ) ;
#37844=CARTESIAN_POINT ( 'NONE',  ( -86.93036351089999414, 1384.859295106799891, 307.7327112012590078 ) ) ;
#37846=CARTESIAN_POINT ( 'NONE',  ( -20.71467568763819855, 1385.273462423449928, 221.2323961153799985 ) ) ;
#37881=CARTESIAN_POINT ( 'NONE',  ( -103.9247617160000203, 1379.900991233349941, 303.2459714484589881 ) ) ;
#37893=EDGE_CURVE ( 'NONE', #70768, #17951, #31081, .T. ) ;
#37896=CARTESIAN_POINT ( 'NONE',  ( -85.71654444118949812, 1383.773072311060105, 306.8335668707890136 ) ) ;
#37897=CARTESIAN_POINT ( 'NONE',  ( -108.9547098300069905, 1384.162005566360222, 311.1881139208990135 ) ) ;
#37902=CARTESIAN_POINT ( 'NONE',  ( -106.4664531209999865, 1381.040142295360056, 309.4626932862590252 ) ) ;
#37906=CARTESIAN_POINT ( 'NONE',  ( -110.0628372420000005, 1384.916020893610039, 296.9513042793590216 ) ) ;
#37920=CARTESIAN_POINT ( 'NONE',  ( -107.8662654264032170, 1378.913060344626274, 308.7118336974646695 ) ) ;
#37948=CIRCLE ( 'NONE', #46918, 7.842199003069996621 ) ;
#37954=CARTESIAN_POINT ( 'NONE',  ( -15.50041385721359966, 1384.523326672639996, 200.7202488855130014 ) ) ;
#37984=CARTESIAN_POINT ( 'NONE',  ( -14.05223976236401207, 1379.587684537167888, 211.8183454839635260 ) ) ;
#37999=CARTESIAN_POINT ( 'NONE',  ( -12.31052647389649835, 1378.376188973679973, 209.7933296302919928 ) ) ;
#38003=CARTESIAN_POINT ( 'NONE',  ( -109.5388894170000071, 1385.012700822230272, 297.1239152411590112 ) ) ;
#38005=EDGE_LOOP ( 'NONE', ( #107086, #53757, #24701, #33505, #19320, #6303, #76801, #39455, #69891, #83818, #74948, #82475 ) ) ;
#38009=CARTESIAN_POINT ( 'NONE',  ( -113.4000000000000057, 1379.886883438980021, 304.2218459572590064 ) ) ;
#38016=CARTESIAN_POINT ( 'NONE',  ( -25.99927661702099968, 1383.846917199799918, 224.2199440044900030 ) ) ;
#38024=CARTESIAN_POINT ( 'NONE',  ( -37.09676805939999866, 1383.024146519360102, 210.3189902961190114 ) ) ;
#38030=CARTESIAN_POINT ( 'NONE',  ( -12.31798489929459883, 1389.268006845099990, 215.3113464096479959 ) ) ;
#38037=CARTESIAN_POINT ( 'NONE',  ( -7.965810688893188996, 1384.899971919800009, 199.4892299149449855 ) ) ;
#38038=CARTESIAN_POINT ( 'NONE',  ( -98.60501928763169133, 1385.217285518659992, 295.9932508494239869 ) ) ;
#38041=CARTESIAN_POINT ( 'NONE',  ( -67.63612853559999394, 1379.748709736400087, 277.8550023105590299 ) ) ;
#38082=B_SPLINE_CURVE_WITH_KNOTS ( 'NONE', 3,
 ( #13226, #107308, #41210, #25485, #58573, #7599, #110614, #8141, #24923, #50711, #50180, #41753, #33896, #92701, #75912, #16520, #84841, #42307, #51260, #109519, #59134, #102205, #42870, #84307, #66979, #33339, #24389, #68092, #110064, #67534, #101634 ),
 .UNSPECIFIED., .F., .F.,
 ( 4, 3, 3, 3, 3, 3, 3, 3, 3, 3, 4 ),
 ( -15.26427302110819895, -15.05934333483120113, -14.73799943699000004, -14.51062177820000088, -14.45665274134599976, -14.26912914067029980, -14.02763650314049926, -13.81025237607900102, -13.62933106218500079, -13.46144724711600027, -13.44470524421359947 ),
 .UNSPECIFIED. ) ;
#38087=CARTESIAN_POINT ( 'NONE',  ( -113.4000000000000057, 1390.913060387289988, 304.2218459572590064 ) ) ;
#38110=CARTESIAN_POINT ( 'NONE',  ( -43.47249194638170877, 1379.734446419809728, 233.2730947036674820 ) ) ;
#38116=CARTESIAN_POINT ( 'NONE',  ( -86.43489313709348210, 1384.977908500060039, 307.3521131436049814 ) ) ;
#38163=CARTESIAN_POINT ( 'NONE',  ( -90.01802904232170022, 1384.619177581419990, 308.7061652526469970 ) ) ;
#38164=CARTESIAN_POINT ( 'NONE',  ( -36.70638529991089882, 1384.982332475140083, 210.0042769290089950 ) ) ;
#38178=CARTESIAN_POINT ( 'NONE',  ( -106.4682402945449979, 1391.913060387289988, 304.9855591817990330 ) ) ;
#38182=CARTESIAN_POINT ( 'NONE',  ( -12.47403649690000016, 1380.456715030230043, 204.1115024872290178 ) ) ;
#38193=CARTESIAN_POINT ( 'NONE',  ( -67.60933340069999531, 1379.747570940439800, 278.8523720603590164 ) ) ;
#38209=CARTESIAN_POINT ( 'NONE',  ( -113.4000000000000057, 1384.926148861439970, 304.2218459572590064 ) ) ;
#38220=CARTESIAN_POINT ( 'NONE',  ( -8.861481481760000278, 1384.950957064560043, 218.6848129458689982 ) ) ;
#38222=CARTESIAN_POINT ( 'NONE',  ( -68.43253263535059716, 1379.747293324333214, 279.3372337453455998 ) ) ;
#38226=CARTESIAN_POINT ( 'NONE',  ( -53.73769481676529836, 1384.637522084219881, 231.5445279993439840 ) ) ;
#38233=LINE ( 'NONE', #72957, #3465 ) ;
#38235=CARTESIAN_POINT ( 'NONE',  ( -108.6616353267809956, 1383.758284946439971, 311.0749865448200353 ) ) ;
#38242=CARTESIAN_POINT ( 'NONE',  ( -113.4000000000000057, 1379.913060387289988, 304.2218459572590064 ) ) ;
#38256=CARTESIAN_POINT ( 'NONE',  ( -8.156522882179999101, 1384.901372997500175, 199.6468678763889955 ) ) ;
#38265=CARTESIAN_POINT ( 'NONE',  ( -14.08142637225379978, 1379.709117121690042, 211.5303641152310092 ) ) ;
#38271=B_SPLINE_CURVE_WITH_KNOTS ( 'NONE', 3,
 ( #17118, #101689, #50762, #24980, #85443, #8190, #62950, #53983, #96502, #53410, #42356, #45022, #37145, #33387, #36053, #105456, #10850, #87561, #79167, #77081, #36592, #70789, #16567, #28745, #67583, #95948, #59186, #11406, #84898, #93305, #110660, #88117, #59727, #68147, #93846, #28190, #33953, #62376, #104347, #97061, #42924, #102257, #61825, #41806, #104901, #70240, #20326, #45574, #25536, #27640, #389, #51306, #79716, #19208, #19782, #3023, #54531, #7649, #75963, #99225 ),
 .UNSPECIFIED., .F., .F.,
 ( 4, 2, 2, 2, 2, 2, 2, 1, 1, 1, 1, 1, 1, 2, 2, 2, 2, 2, 2, 2, 1, 1, 1, 1, 1, 1, 2, 2, 2, 2, 2, 2, 2, 2, 2, 4 ),
 ( 0.000000000000000000, 0.06249999999921360128, 0.1249999999984272026, 0.1874999999976408038, 0.2187499999972475906, 0.2343749999970505260, 0.2421874999969520492, 0.2460937499969024223, 0.2480468749968771647, 0.2490234374968641196, 0.2495117187468572084, 0.2497558593718541831, 0.2498779296843522402, 0.2499389648406012965, 0.2499999999968503250, 0.3124999999970974884, 0.3749999999973447351, 0.4374999999975927589, 0.4687499999977168263, 0.4843749999977786103, 0.4921874999978098630, 0.4960937499978254617, 0.4980468749978333443, 0.4990234374978368970, 0.4995117187478387843, 0.4997558593728400056, 0.4998779296853406162, 0.4999999999978411713, 0.5624999999981110665, 0.6249999999983808507, 0.6874999999986507460, 0.7499999999989206412, 0.8124999999991905364, 0.8749999999994603206, 0.9374999999997302158, 1.000000000000000000 ),
 .UNSPECIFIED. ) ;
#38290=CARTESIAN_POINT ( 'NONE',  ( -31.26379401350899556, 1384.823741200369795, 229.4291413252929885 ) ) ;
#38310=CARTESIAN_POINT ( 'NONE',  ( -109.9870827704239957, 1384.734719174579823, 311.4521501216929664 ) ) ;
#38315=CARTESIAN_POINT ( 'NONE',  ( -70.05038419870359689, 1379.267308317730112, 286.2875064122259801 ) ) ;
#38317=CARTESIAN_POINT ( 'NONE',  ( -14.06310996700590010, 1379.653384448290126, 211.5922490258780044 ) ) ;
#38326=CARTESIAN_POINT ( 'NONE',  ( -8.163788229310002365, 1383.802161292700021, 218.6403764234589744 ) ) ;
#38341=CARTESIAN_POINT ( 'NONE',  ( 11.33251049156513623, 1391.913060387289988, 208.6449207241230965 ) ) ;
#38345=CARTESIAN_POINT ( 'NONE',  ( -14.39218230554089928, 1380.275882964069979, 209.3755301335680201 ) ) ;
#38348=CARTESIAN_POINT ( 'NONE',  ( -37.92577313569999831, 1377.672836988610015, 218.5611944450689919 ) ) ;
#38350=EDGE_CURVE ( 'NONE', #101907, #1545, #29371, .T. ) ;
#38354=CARTESIAN_POINT ( 'NONE',  ( 7.513435694541056975, 1375.426148861440197, 209.1218459572589836 ) ) ;
#38364=CARTESIAN_POINT ( 'NONE',  ( -25.97701990859999910, 1384.174749255760162, 224.1963252206589914 ) ) ;
#38369=CARTESIAN_POINT ( 'NONE',  ( -67.44338435920001018, 1379.744787917099757, 277.3736694360590036 ) ) ;
#38379=CARTESIAN_POINT ( 'NONE',  ( -102.7375125960000020, 1384.595838641269893, 311.2202755702589911 ) ) ;
#38381=CARTESIAN_POINT ( 'NONE',  ( -29.36584213358230144, 1385.236513890409924, 227.3793372904949877 ) ) ;
#38391=CARTESIAN_POINT ( 'NONE',  ( -7.989567385690000023, 1384.306347471770096, 199.5291465469090042 ) ) ;
#38409=CARTESIAN_POINT ( 'NONE',  ( -106.0175964039999883, 1391.835588392369800, 302.7430365994590034 ) ) ;
#38411=DIRECTION ( 'NONE',  ( -0.4709675661680092218, 0.8364468003938373419, 0.2802611313198711263 ) ) ;
#38413=CARTESIAN_POINT ( 'NONE',  ( -104.2041774089999961, 1379.825158453460062, 303.6443917302590307 ) ) ;
#38430=CARTESIAN_POINT ( 'NONE',  ( -109.9987473190000031, 1384.904025801279886, 297.1695833602590255 ) ) ;
#38442=ADVANCED_FACE ( 'NONE', ( #14222 ), #86893, .T. ) ;
#38485=CARTESIAN_POINT ( 'NONE',  ( -16.04653612434290011, 1384.524557204450048, 200.8152124474479763 ) ) ;
#38539=CARTESIAN_POINT ( 'NONE',  ( -110.0571759400000076, 1385.284143576950100, 296.9644176183589366 ) ) ;
#38548=CARTESIAN_POINT ( 'NONE',  ( -49.92459275517279593, 1383.812035811190071, 261.1885675870709633 ) ) ;
#38557=CARTESIAN_POINT ( 'NONE',  ( -9.008611445770000614, 1379.827692983760016, 214.1021766380889915 ) ) ;
#38562=ORIENTED_EDGE ( 'NONE', *, *, #22945, .F. ) ;
#38564=CARTESIAN_POINT ( 'NONE',  ( -11.54871805396859941, 1389.257702312929950, 215.5751257078669880 ) ) ;
#38583=ADVANCED_FACE ( 'NONE', ( #59013 ), #7998, .F. ) ;
#38597=CARTESIAN_POINT ( 'NONE',  ( -7.543140222519999938, 1385.044701444139946, 219.0850215955189810 ) ) ;
#38642=DIRECTION ( 'NONE',  ( 0.9991156149436395406, 0.000000000000000000, -0.04204744909971582650 ) ) ;
#38653=CARTESIAN_POINT ( 'NONE',  ( -105.4653038608459923, 1391.248269531060259, 304.9316119955079785 ) ) ;
#38661=CARTESIAN_POINT ( 'NONE',  ( -88.41096488174009949, 1384.973236710020046, 308.1529525611489930 ) ) ;
#38662=CARTESIAN_POINT ( 'NONE',  ( -10.43611966299999949, 1387.704879639269848, 201.2730187963089747 ) ) ;
#38674=CARTESIAN_POINT ( 'NONE',  ( -108.4218473026954257, 1388.739376737770726, 298.0879157462472335 ) ) ;
#38704=CARTESIAN_POINT ( 'NONE',  ( -12.29258316900000025, 1378.290984699069895, 210.0372636615540216 ) ) ;
#38705=CARTESIAN_POINT ( 'NONE',  ( -86.03463923215619502, 1384.626609384469930, 307.1684108349550115 ) ) ;
#38706=CARTESIAN_POINT ( 'NONE',  ( -28.43854200076519945, 1384.965860001799911, 204.7629818153700114 ) ) ;
#38714=CARTESIAN_POINT ( 'NONE',  ( -109.1308226289999936, 1384.913202581150017, 311.2647286892589591 ) ) ;
#38725=CARTESIAN_POINT ( 'NONE',  ( -11.82847241660000037, 1380.969823483590062, 203.0484502812290089 ) ) ;
#38726=CARTESIAN_POINT ( 'NONE',  ( -11.39126005979999867, 1381.496251003520001, 216.9356158229890070 ) ) ;
#38737=CARTESIAN_POINT ( 'NONE',  ( -67.67707935839548838, 1379.746493294780066, 278.9722144515000082 ) ) ;
#38743=CARTESIAN_POINT ( 'NONE',  ( -109.1316882649999940, 1384.947817856130087, 311.2645137162589890 ) ) ;
#38749=CARTESIAN_POINT ( 'NONE',  ( -107.8376371489249976, 1378.913060387289988, 308.2679488075570475 ) ) ;
#38759=CARTESIAN_POINT ( 'NONE',  ( -11.15007135000000105, 1391.248055150329947, 203.8486859877390032 ) ) ;
#38769=CARTESIAN_POINT ( 'NONE',  ( -68.43664974299086623, 1379.747301587279026, 279.3461838679465927 ) ) ;
#38773=CARTESIAN_POINT ( 'NONE',  ( -50.68086562047950139, 1384.622718412899758, 226.3488145558480085 ) ) ;
#38783=CARTESIAN_POINT ( 'NONE',  ( -108.7285119980398207, 1383.837283289873085, 311.1015258184347658 ) ) ;
#38802=CARTESIAN_POINT ( 'NONE',  ( -113.4000000000000057, 1384.913060387289988, 311.2218459572590064 ) ) ;
#38837=CARTESIAN_POINT ( 'NONE',  ( -41.36494379132859223, 1384.781339806650067, 244.5749991835589867 ) ) ;
#38839=AXIS2_PLACEMENT_3D ( 'NONE', #465, #86644, #78811 ) ;
#38841=CARTESIAN_POINT ( 'NONE',  ( -105.4633420800000039, 1378.947304614410086, 304.0408918711589763 ) ) ;
#38853=DIRECTION ( 'NONE',  ( 1.000000000000000000, 0.000000000000000000, 0.000000000000000000 ) ) ;
#38861=CARTESIAN_POINT ( 'NONE',  ( -93.69296856029690446, 1378.179795124779957, 305.3712508567500095 ) ) ;
#38872=CARTESIAN_POINT ( 'NONE',  ( -103.5807003099999974, 1389.940341032420065, 304.1776946944589781 ) ) ;
#38888=CARTESIAN_POINT ( 'NONE',  ( -109.4005255434914972, 1387.066694983333036, 311.0856849982282029 ) ) ;
#38890=CARTESIAN_POINT ( 'NONE',  ( -12.34596455585159980, 1378.847116221920032, 209.2104869998679817 ) ) ;
#38894=CARTESIAN_POINT ( 'NONE',  ( -50.14839348009999753, 1380.010081756269983, 242.5009839091590038 ) ) ;
#38905=DIRECTION ( 'NONE',  ( 0.000000000000000000, 0.000000000000000000, -1.000000000000000000 ) ) ;
#38907=CARTESIAN_POINT ( 'NONE',  ( -49.58793988690000276, 1384.741903095260113, 260.9101892837590526 ) ) ;
#38911=CARTESIAN_POINT ( 'NONE',  ( -50.79448650070000326, 1379.685520326630012, 241.2356115758589965 ) ) ;
#38924=CARTESIAN_POINT ( 'NONE',  ( -30.72941576718060119, 1385.230165571390216, 228.8128147210159966 ) ) ;
#38948=CARTESIAN_POINT ( 'NONE',  ( -103.5806803890000083, 1389.940350142260058, 304.1776731731589507 ) ) ;
#38951=CARTESIAN_POINT ( 'NONE',  ( -106.5381113420000077, 1391.812866088840110, 301.3072072504589869 ) ) ;
#38960=CARTESIAN_POINT ( 'NONE',  ( -113.4000000000000057, 1384.913060387289988, 304.2218459572590064 ) ) ;
#38980=CARTESIAN_POINT ( 'NONE',  ( -109.7177012239999954, 1384.912553384849843, 297.0861780560589978 ) ) ;
#38981=CARTESIAN_POINT ( 'NONE',  ( -11.42312749683812356, 1378.600463633266827, 204.4622889030064243 ) ) ;
#39012=CARTESIAN_POINT ( 'NONE',  ( -11.45492292490000175, 1391.035318004910096, 204.4802647352790075 ) ) ;
#39027=CARTESIAN_POINT ( 'NONE',  ( -27.30026132067300182, 1384.549843020650087, 204.2521262686249770 ) ) ;
#39058=CARTESIAN_POINT ( 'NONE',  ( -14.08275829279420499, 1379.695270052737214, 211.5466488430092795 ) ) ;
#39087=CARTESIAN_POINT ( 'NONE',  ( -14.17772861730700207, 1379.591530685439920, 207.8208986668599891 ) ) ;
#39091=CARTESIAN_POINT ( 'NONE',  ( -50.45191962221719706, 1383.811169775679900, 262.2738409289869992 ) ) ;
#39102=CARTESIAN_POINT ( 'NONE',  ( -19.23736494940000341, 1383.854422637459948, 220.3626903602589948 ) ) ;
#39110=CARTESIAN_POINT ( 'NONE',  ( -10.91935502263179991, 1388.739090993680065, 216.4564496294659932 ) ) ;
#39118=CARTESIAN_POINT ( 'NONE',  ( -109.0556933945980091, 1385.242281295139946, 297.1439643352929920 ) ) ;
#39132=CARTESIAN_POINT ( 'NONE',  ( -108.9389063659999977, 1385.729741725900112, 311.1830050262590248 ) ) ;
#39145=CARTESIAN_POINT ( 'NONE',  ( -7.776723803980000405, 1385.308312221739925, 218.8990009525190317 ) ) ;
#39149=ADVANCED_FACE ( 'NONE', ( #6572 ), #55312, .F. ) ;
#39176=ORIENTED_EDGE ( 'NONE', *, *, #78940, .F. ) ;
#39194=CARTESIAN_POINT ( 'NONE',  ( -108.6053824472246561, 1381.341894323206361, 297.9344204043421769 ) ) ;
#39198=CARTESIAN_POINT ( 'NONE',  ( -106.7386023904570038, 1391.793764057960061, 307.5809146916449777 ) ) ;
#39207=CARTESIAN_POINT ( 'NONE',  ( -95.82886112073660456, 1384.956069587409957, 310.2164913438589906 ) ) ;
#39209=CARTESIAN_POINT ( 'NONE',  ( -10.60441893339999986, 1387.604333835939997, 201.2306567222790363 ) ) ;
#39230=TOROIDAL_SURFACE ( 'NONE', #24905, 6.868727599660000571, 1.000000000000000000 ) ;
#39252=CARTESIAN_POINT ( 'NONE',  ( -103.9670040342639794, 1380.172649198307454, 306.3874380259700274 ) ) ;
#39260=CARTESIAN_POINT ( 'NONE',  ( -12.50373372780000025, 1379.339414555010080, 210.6530944808689867 ) ) ;
#39261=CARTESIAN_POINT ( 'NONE',  ( -108.2169316518169921, 1384.585047728120117, 311.2483635071519643 ) ) ;
#39262=CARTESIAN_POINT ( 'NONE',  ( -55.20995173741290074, 1385.039367042840013, 234.2426462848850122 ) ) ;
#39275=CARTESIAN_POINT ( 'NONE',  ( -109.4870104200000043, 1384.778285814570154, 311.2819397492589815 ) ) ;
#39297=CARTESIAN_POINT ( 'NONE',  ( -68.30538991723700804, 1379.747268421340095, 279.8418067756310279 ) ) ;
#39311=CARTESIAN_POINT ( 'NONE',  ( -14.53473304376390018, 1379.710786975620067, 208.2794084638009906 ) ) ;
#39333=CARTESIAN_POINT ( 'NONE',  ( -67.88352385773819719, 1384.723690489739965, 261.4186645314100588 ) ) ;
#39364=CARTESIAN_POINT ( 'NONE',  ( -7.966175666139999834, 1384.907333411119907, 199.4893255676990123 ) ) ;
#39376=CARTESIAN_POINT ( 'NONE',  ( -13.48561026711389843, 1379.693410661539929, 211.4566350483709982 ) ) ;
#39389=EDGE_CURVE ( 'NONE', #56949, #62022, #40369, .T. ) ;
#39391=CARTESIAN_POINT ( 'NONE',  ( -106.4020496450190052, 1391.913060387289988, 304.2007955189830568 ) ) ;
#39399=CARTESIAN_POINT ( 'NONE',  ( -9.240621257877769779, 1384.939706531919910, 197.9480711716310282 ) ) ;
#39401=CARTESIAN_POINT ( 'NONE',  ( -24.10034866325270286, 1384.849111676500115, 223.0989387258899797 ) ) ;
#39402=CARTESIAN_POINT ( 'NONE',  ( -106.4135441880139865, 1391.913060387269979, 303.8057445950980195 ) ) ;
#39406=CARTESIAN_POINT ( 'NONE',  ( -105.4748444820000088, 1379.159997331010118, 302.2473400626589637 ) ) ;
#39430=CARTESIAN_POINT ( 'NONE',  ( -16.64413823199859976, 1379.585478419799983, 212.2328527173980035 ) ) ;
#39455=ORIENTED_EDGE ( 'NONE', *, *, #42486, .T. ) ;
#39459=CARTESIAN_POINT ( 'NONE',  ( -109.1939007313264369, 1387.425512231509856, 310.9496258952415246 ) ) ;
#39462=CARTESIAN_POINT ( 'NONE',  ( -12.32664172942340031, 1378.996309998719880, 209.7960268208129833 ) ) ;
#39467=CARTESIAN_POINT ( 'NONE',  ( -42.70366651140000158, 1375.424979822739942, 226.7036006363589991 ) ) ;
#39474=B_SPLINE_SURFACE_WITH_KNOTS ( 'NONE', 5, 5, ( 
 ( #11493, #56246, #98787, #96598, #19869, #71440 ),
 ( #73051, #71982, #62478, #20412, #20962, #4193 ),
 ( #12585, #90375, #38326, #72505, #3112, #13653 ),
 ( #81976, #54073, #88749, #5284, #64114, #45668 ),
 ( #70880, #79807, #104992, #21504, #28283, #98235 ),
 ( #63573, #12033, #105555, #37241, #46766, #28842 ),
 ( #63038, #55718, #89837, #97144, #46214, #81417 ),
 ( #80348, #37794, #106095, #29373, #97689, #55166 ),
 ( #89290, #13110, #47293, #40538, #31029, #99875 ) ),
 .UNSPECIFIED., .F., .F., .F.,
 ( 6, 3, 6 ),
 ( 6, 6 ),
 ( 24.41308947359999948, 25.74260990720000208, 27.07213034080000114 ),
 ( 0.000000000000000000, 2.000000000000000000 ),
 .UNSPECIFIED. ) ;
#39481=CARTESIAN_POINT ( 'NONE',  ( -89.65362972180000156, 1384.619809472219913, 308.7387643915590161 ) ) ;
#39486=CARTESIAN_POINT ( 'NONE',  ( -47.65858604169999779, 1379.688530322980114, 235.3355530128589805 ) ) ;
#39495=CARTESIAN_POINT ( 'NONE',  ( -45.21221387570000161, 1388.283329091300175, 219.7150970607590068 ) ) ;
#39497=CARTESIAN_POINT ( 'NONE',  ( -42.52088808034810086, 1385.167360014890164, 246.7025410803429963 ) ) ;
#39524=CARTESIAN_POINT ( 'NONE',  ( -104.1029534810000001, 1389.819474454779993, 301.8406320987589879 ) ) ;
#39529=CARTESIAN_POINT ( 'NONE',  ( -104.5268087689999987, 1379.723412970779918, 303.3030969148589975 ) ) ;
#39546=CARTESIAN_POINT ( 'NONE',  ( -89.86981536200001131, 1382.337715003790208, 308.1217387938589809 ) ) ;
#39562=CARTESIAN_POINT ( 'NONE',  ( -107.3811187542021912, 1379.376395203810944, 309.1054750742122224 ) ) ;
#39579=CARTESIAN_POINT ( 'NONE',  ( -8.602704958620000397, 1384.751806508920026, 199.8723417454790194 ) ) ;
#39601=CARTESIAN_POINT ( 'NONE',  ( -13.70478788754319943, 1384.519254815689919, 200.4442307571110007 ) ) ;
#39611=CARTESIAN_POINT ( 'NONE',  ( -11.38166339569999863, 1381.807649517150139, 201.7589817661390157 ) ) ;
#39667=CARTESIAN_POINT ( 'NONE',  ( -45.07337503762840214, 1383.820054821190070, 251.3008954162190207 ) ) ;
#39676=CARTESIAN_POINT ( 'NONE',  ( -29.04720760670000246, 1380.913020375419819, 224.0879423276590217 ) ) ;
#39682=CARTESIAN_POINT ( 'NONE',  ( -8.945497862365648700, 1385.615016313520073, 218.6252861300649784 ) ) ;
#39685=CARTESIAN_POINT ( 'NONE',  ( -106.5042781940000083, 1381.696109913969849, 298.6533303033589846 ) ) ;
#39703=CARTESIAN_POINT ( 'NONE',  ( -109.2173541970000059, 1385.843882786750100, 311.1794573962590107 ) ) ;
#39729=CARTESIAN_POINT ( 'NONE',  ( -107.7967585290650021, 1378.913060387369796, 300.1988973161450076 ) ) ;
#39735=CARTESIAN_POINT ( 'NONE',  ( -9.853078183510000088, 1384.932634673870098, 199.8720430995890069 ) ) ;
#39774=CIRCLE ( 'NONE', #73766, 12.49965726619999984 ) ;
#39776=CARTESIAN_POINT ( 'NONE',  ( -82.94653126506901231, 1384.986406227859788, 305.6412706045470600 ) ) ;
#39777=CARTESIAN_POINT ( 'NONE',  ( -8.083309084479999740, 1385.702140206949935, 199.6133739923190262 ) ) ;
#39783=CARTESIAN_POINT ( 'NONE',  ( -7.544821708607240218, 1384.901423427800182, 219.0876899943770013 ) ) ;
#39790=CARTESIAN_POINT ( 'NONE',  ( -109.4257410045153165, 1387.211591992306467, 297.3482829929823765 ) ) ;
#39814=CARTESIAN_POINT ( 'NONE',  ( -107.6855514720864306, 1382.839660080642034, 310.6340048910524274 ) ) ;
#39817=DIRECTION ( 'NONE',  ( -0.9996573249755569268, -0.02617694830788819954, 0.000000000000000000 ) ) ;
#39818=CARTESIAN_POINT ( 'NONE',  ( -109.1314732179999965, 1384.943873489550015, 311.2645625782590173 ) ) ;
#39820=FACE_OUTER_BOUND ( 'NONE', #20854, .T. ) ;
#39822=CARTESIAN_POINT ( 'NONE',  ( -50.05828054499940549, 1385.019276194180065, 225.3411702308840177 ) ) ;
#39833=CARTESIAN_POINT ( 'NONE',  ( -113.4000000000000057, 1389.413060387289988, 304.2218459572590064 ) ) ;
#39852=CARTESIAN_POINT ( 'NONE',  ( -68.69425754540708340, 1379.747748063760127, 280.2977437733629813 ) ) ;
#39863=CARTESIAN_POINT ( 'NONE',  ( -106.7579877504269916, 1378.913060387289988, 306.8343690171730032 ) ) ;
#39885=CARTESIAN_POINT ( 'NONE',  ( -81.16297568175110655, 1384.800030316710036, 284.5901439566409863 ) ) ;
#39895=CARTESIAN_POINT ( 'NONE',  ( -5.013435694540000043, 1375.426148861440197, 209.1218459569879826 ) ) ;
#39922=CARTESIAN_POINT ( 'NONE',  ( -68.77278092737650184, 1379.747928288920093, 280.3133413970129482 ) ) ;
#39952=CARTESIAN_POINT ( 'NONE',  ( -58.27305785222070256, 1384.702705549079838, 277.9433341154070263 ) ) ;
#39977=CARTESIAN_POINT ( 'NONE',  ( -25.65044697828639997, 1380.250345453750015, 213.2121384338130099 ) ) ;
#40005=CARTESIAN_POINT ( 'NONE',  ( -108.4178825058906170, 1388.553815689287148, 310.3588190281001857 ) ) ;
#40007=CARTESIAN_POINT ( 'NONE',  ( -12.33756948541939913, 1378.984672000980254, 209.5697532986669671 ) ) ;
#40012=CARTESIAN_POINT ( 'NONE',  ( -42.05438492420000074, 1380.117442312619914, 227.1521432528590196 ) ) ;
#40014=VERTEX_POINT ( 'NONE', #93464 ) ;
#40025=CARTESIAN_POINT ( 'NONE',  ( -62.07136965400000150, 1384.687060561920134, 284.7656473558590164 ) ) ;
#40039=CARTESIAN_POINT ( 'NONE',  ( -50.80916825539999593, 1386.657926508519949, 226.1996310703590041 ) ) ;
#40041=CARTESIAN_POINT ( 'NONE',  ( -53.36249814381680068, 1385.102014360260227, 268.5762821108210119 ) ) ;
#40051=CARTESIAN_POINT ( 'NONE',  ( -8.297772639310000642, 1384.896939720920045, 218.7035975184890049 ) ) ;
#40070=CARTESIAN_POINT ( 'NONE',  ( -106.3702501619999907, 1389.389845767869929, 299.7163509613590122 ) ) ;
#40072=CARTESIAN_POINT ( 'NONE',  ( -106.5052939700000110, 1391.913060387289988, 302.8727176574589635 ) ) ;
#40090=CARTESIAN_POINT ( 'NONE',  ( -103.3000534650000048, 1379.387642428310073, 303.1956711788589587 ) ) ;
#40093=EDGE_LOOP ( 'NONE', ( #97349, #1081, #11739, #106345 ) ) ;
#40110=EDGE_LOOP ( 'NONE', ( #15375, #95082, #59407, #15387 ) ) ;
#40118=CARTESIAN_POINT ( 'NONE',  ( -8.617791468060000071, 1384.526991232059800, 199.8918045177789793 ) ) ;
#40131=CARTESIAN_POINT ( 'NONE',  ( -107.2899050854710055, 1379.886892357829993, 309.1794776302379546 ) ) ;
#40159=CARTESIAN_POINT ( 'NONE',  ( -68.77190080519999071, 1379.747925807450201, 280.3125203366930123 ) ) ;
#40166=VERTEX_POINT ( 'NONE', #2477 ) ;
#40190=ADVANCED_FACE ( 'NONE', ( #97063 ), #108605, .F. ) ;
#40213=CARTESIAN_POINT ( 'NONE',  ( -41.29375914184250007, 1383.826143227880038, 244.0855120829130271 ) ) ;
#40221=CARTESIAN_POINT ( 'NONE',  ( -31.91391880200000131, 1384.560375756019766, 206.3213236589990061 ) ) ;
#40225=CARTESIAN_POINT ( 'NONE',  ( -7.924974002880879276, 1385.447079371110021, 218.8285693757050012 ) ) ;
#40230=CARTESIAN_POINT ( 'NONE',  ( -103.9810530660000012, 1379.936289390329875, 302.8711362071589974 ) ) ;
#40277=CARTESIAN_POINT ( 'NONE',  ( -68.71403817000000913, 1384.980557972010047, 263.4288273180590068 ) ) ;
#40287=AXIS2_PLACEMENT_3D ( 'NONE', #76586, #110737, #34028 ) ;
#40308=DIRECTION ( 'NONE',  ( 1.836970198721029688E-16, 1.000000000000000000, -1.793662034335764721E-47 ) ) ;
#40312=EDGE_LOOP ( 'NONE', ( #5518, #46664, #72241, #110352, #28017 ) ) ;
#40315=CARTESIAN_POINT ( 'NONE',  ( -82.57267637850920039, 1384.987339562300122, 305.4358940477329725 ) ) ;
#40317=CARTESIAN_POINT ( 'NONE',  ( -8.716424698579999131, 1385.235525592430122, 199.8893934550389986 ) ) ;
#40333=DIRECTION ( 'NONE',  ( 1.836970198721029688E-16, 1.000000000000000000, -2.953460612019999929E-19 ) ) ;
#40353=CARTESIAN_POINT ( 'NONE',  ( -103.9934435520329572, 1380.191563112924086, 306.4628881227609440 ) ) ;
#40358=CARTESIAN_POINT ( 'NONE',  ( -13.06039920679999966, 1380.082784840310069, 210.0204466537629742 ) ) ;
#40360=CARTESIAN_POINT ( 'NONE',  ( -65.65150386709079555, 1385.090028818440032, 256.4968730652950057 ) ) ;
#40361=CARTESIAN_POINT ( 'NONE',  ( -5.512208796550629231, 1374.913060387289988, 214.9365724502839896 ) ) ;
#40369=CIRCLE ( 'NONE', #75944, 2.000048419052109061 ) ;
#40373=CARTESIAN_POINT ( 'NONE',  ( -109.4760068020000006, 1384.604117400059977, 311.2718567032590045 ) ) ;
#40374=FACE_OUTER_BOUND ( 'NONE', #15606, .T. ) ;
#40390=CARTESIAN_POINT ( 'NONE',  ( -68.54637881447411019, 1379.747431728610081, 280.1644567549890326 ) ) ;
#40393=CARTESIAN_POINT ( 'NONE',  ( -9.431129421125392653, 1380.292824618373061, 217.1402169329579692 ) ) ;
#40402=CARTESIAN_POINT ( 'NONE',  ( -107.1548411235229992, 1378.913060387289988, 307.3968287292940431 ) ) ;
#40412=VERTEX_POINT ( 'NONE', #60604 ) ;
#40425=DIRECTION ( 'NONE',  ( 1.836970198721029688E-16, 1.000000000000000000, 0.000000000000000000 ) ) ;
#40427=CARTESIAN_POINT ( 'NONE',  ( -67.46733395234829800, 1384.720989913540052, 260.5131342236279579 ) ) ;
#40434=ORIENTED_EDGE ( 'NONE', *, *, #104226, .F. ) ;
#40464=CARTESIAN_POINT ( 'NONE',  ( -61.49666415160000099, 1379.841752510579909, 267.0938153646590649 ) ) ;
#40482=CARTESIAN_POINT ( 'NONE',  ( -8.894733913401703163, 1388.790479115094513, 217.7593060885732825 ) ) ;
#40488=DIRECTION ( 'NONE',  ( 0.02617694830785712717, 0.9996573249755577040, 1.162500616384811670E-17 ) ) ;
#40498=CARTESIAN_POINT ( 'NONE',  ( -47.50847041448220409, 1384.752078445960024, 256.6134531784289834 ) ) ;
#40499=CARTESIAN_POINT ( 'NONE',  ( -106.7778451161910169, 1391.913060387289988, 302.2346433575910396 ) ) ;
#40514=CARTESIAN_POINT ( 'NONE',  ( -12.24109810896139905, 1378.509644311850025, 210.6652527242490009 ) ) ;
#40524=CARTESIAN_POINT ( 'NONE',  ( -3.771520279010110333, 1379.944275571289836, 211.0169301715230006 ) ) ;
#40528=CARTESIAN_POINT ( 'NONE',  ( -48.00211451008600250, 1379.678745322079976, 241.5445238333160205 ) ) ;
#40538=CARTESIAN_POINT ( 'NONE',  ( -8.297292677919999804, 1384.885217424229950, 218.7035352471990279 ) ) ;
#40558=CARTESIAN_POINT ( 'NONE',  ( -12.31949145670699863, 1378.253786499809848, 209.5105070175480080 ) ) ;
#40563=CARTESIAN_POINT ( 'NONE',  ( -46.19755678850000180, 1376.012990379910207, 231.0255711751590013 ) ) ;
#40576=CARTESIAN_POINT ( 'NONE',  ( -32.23247795450000552, 1383.839374993809770, 229.8499276021589992 ) ) ;
#40591=CARTESIAN_POINT ( 'NONE',  ( -52.53197402710000574, 1389.553010688960057, 259.5557295571589975 ) ) ;
#40593=CARTESIAN_POINT ( 'NONE',  ( -46.06484833219570163, 1385.146025147649880, 253.6578770933249984 ) ) ;
#40603=CARTESIAN_POINT ( 'NONE',  ( -7.768947876059999480, 1384.898102977279905, 218.9179155823389920 ) ) ;
#40620=CARTESIAN_POINT ( 'NONE',  ( -105.9329978819999951, 1390.513368602009905, 301.0435293657589568 ) ) ;
#40622=CARTESIAN_POINT ( 'NONE',  ( -106.8917078750000087, 1391.793768397970098, 300.5749944091589896 ) ) ;
#40697=CARTESIAN_POINT ( 'NONE',  ( -29.17179959739380379, 1384.554205719389984, 205.1512235203240095 ) ) ;
#40703=EDGE_LOOP ( 'NONE', ( #69946, #42253, #95654, #81587 ) ) ;
#40710=AXIS2_PLACEMENT_3D ( 'NONE', #100913, #75203, #5228 ) ;
#40712=CARTESIAN_POINT ( 'NONE',  ( -68.78404569073209984, 1379.747969732330148, 280.2963111448109998 ) ) ;
#40720=CARTESIAN_POINT ( 'NONE',  ( -8.743902791170000910, 1385.175134629190097, 218.5746284983589760 ) ) ;
#40721=ORIENTED_EDGE ( 'NONE', *, *, #96917, .F. ) ;
#40748=CARTESIAN_POINT ( 'NONE',  ( -109.7187103849999943, 1384.936990287839990, 297.0861910508589858 ) ) ;
#40763=CARTESIAN_POINT ( 'NONE',  ( -44.53843405880110140, 1383.820931003150008, 250.2441383139970128 ) ) ;
#40773=CARTESIAN_POINT ( 'NONE',  ( -47.53302541269999892, 1383.816002435690052, 256.2046081452590442 ) ) ;
#40778=CARTESIAN_POINT ( 'NONE',  ( -8.951560400169498166, 1386.309576927779972, 218.4184569005070102 ) ) ;
#40783=CARTESIAN_POINT ( 'NONE',  ( -106.6208966620000069, 1378.950518748449895, 300.1891795401589320 ) ) ;
#40831=CARTESIAN_POINT ( 'NONE',  ( -84.13410175530000856, 1384.933881297359903, 288.0523788940590180 ) ) ;
#40863=CARTESIAN_POINT ( 'NONE',  ( -12.49949197370000142, 1379.134263153570146, 212.2053367160189907 ) ) ;
#40869=CARTESIAN_POINT ( 'NONE',  ( -9.075511479460001141, 1387.789233278139818, 200.5952413198190243 ) ) ;
#40875=CARTESIAN_POINT ( 'NONE',  ( -9.087937995490110055, 1383.941172989790175, 218.5505186622879989 ) ) ;
#40880=CARTESIAN_POINT ( 'NONE',  ( -109.9515965448952528, 1385.962241300529513, 297.0326770096235691 ) ) ;
#40900=CARTESIAN_POINT ( 'NONE',  ( -109.5348954149999940, 1384.904938781000055, 297.1231113849590315 ) ) ;
#40905=CARTESIAN_POINT ( 'NONE',  ( -108.1829836398146796, 1383.261649930543399, 310.8763756577378672 ) ) ;
#40908=CARTESIAN_POINT ( 'NONE',  ( -109.1320112420000044, 1384.953741877089897, 311.2644403302589353 ) ) ;
#40911=CARTESIAN_POINT ( 'NONE',  ( -12.52644033109999988, 1379.461106441880020, 210.4487255907489782 ) ) ;
#40914=CARTESIAN_POINT ( 'NONE',  ( -59.40129820653180559, 1385.058454097869799, 242.7081510328939942 ) ) ;
#40922=VERTEX_POINT ( 'NONE', #3196 ) ;
#40927=CARTESIAN_POINT ( 'NONE',  ( -109.4864630750000174, 1384.848068253500060, 311.2837400852590122 ) ) ;
#40945=CARTESIAN_POINT ( 'NONE',  ( -68.53014284327269934, 1379.747351453789861, 280.1403612264239769 ) ) ;
#40955=CARTESIAN_POINT ( 'NONE',  ( -106.4534877654000127, 1378.913060387279984, 306.3385543931779580 ) ) ;
#40962=DIRECTION ( 'NONE',  ( 0.01561979272848090620, -2.869309375241887618E-18, 0.9998780035959984325 ) ) ;
#40972=CARTESIAN_POINT ( 'NONE',  ( -12.62383844309999859, 1379.141235998960155, 208.5749163320770094 ) ) ;
#40976=CARTESIAN_POINT ( 'NONE',  ( -10.81163464159999954, 1391.913060620420083, 213.5809022996290025 ) ) ;
#40977=CARTESIAN_POINT ( 'NONE',  ( -84.10394180980790679, 1384.813803161769783, 287.8662587808539683 ) ) ;
#41014=CARTESIAN_POINT ( 'NONE',  ( -109.6203430457589860, 1383.204584676429931, 311.2218735730909884 ) ) ;
#41028=B_SPLINE_CURVE_WITH_KNOTS ( 'NONE', 3,
 ( #15196, #21936, #21393, #13002, #47186, #42083, #50495, #76233, #9019, #93019, #43192, #85171, #17952, #25249, #85722, #9565, #59451, #51589, #49934, #7912, #93562, #67303, #60559, #34223, #67850 ),
 .UNSPECIFIED., .F., .F.,
 ( 4, 3, 3, 3, 3, 3, 3, 3, 4 ),
 ( -15.26428536230000077, -15.04480521863770015, -14.77980626134180042, -14.51062898585870009, -14.40705048899830132, -14.15432204787279957, -13.90085348180759972, -13.66131906363690085, -13.44470525013180051 ),
 .UNSPECIFIED. ) ;
#41029=CARTESIAN_POINT ( 'NONE',  ( -8.158010031739319601, 1387.526404868172904, 218.5023346017954395 ) ) ;
#41042=CARTESIAN_POINT ( 'NONE',  ( -12.21146186157374558, 1377.806055270933484, 210.7083772430368072 ) ) ;
#41047=CARTESIAN_POINT ( 'NONE',  ( -52.45833321412619910, 1384.728393318099961, 266.7659804183330152 ) ) ;
#41055=CARTESIAN_POINT ( 'NONE',  ( -10.43567586334632935, 1379.713673404171232, 202.4914496242319331 ) ) ;
#41077=CARTESIAN_POINT ( 'NONE',  ( -27.44664266310000400, 1376.937662249230016, 217.0346396320790063 ) ) ;
#41080=CARTESIAN_POINT ( 'NONE',  ( -31.42949257678390040, 1379.646779223169915, 219.2469095604439815 ) ) ;
#41081=ORIENTED_EDGE ( 'NONE', *, *, #37412, .F. ) ;
#41108=CARTESIAN_POINT ( 'NONE',  ( -109.0465141062722410, 1387.661433126290603, 310.8477273668624434 ) ) ;
#41113=CARTESIAN_POINT ( 'NONE',  ( 2.578840932191499675E-14, 1375.413060387289988, 208.3364477938620212 ) ) ;
#41126=CARTESIAN_POINT ( 'NONE',  ( -54.14955217329999471, 1384.412447748920158, 270.3592636482590024 ) ) ;
#41141=CARTESIAN_POINT ( 'NONE',  ( -62.07030651009999644, 1385.055139444880069, 284.7661505247589844 ) ) ;
#41143=CARTESIAN_POINT ( 'NONE',  ( -47.91919660017039462, 1385.134697410870103, 257.4398826552600212 ) ) ;
#41157=CARTESIAN_POINT ( 'NONE',  ( -8.022767810159999513, 1384.891328718069872, 218.7875262018289959 ) ) ;
#41175=CARTESIAN_POINT ( 'NONE',  ( -108.4333501240000004, 1387.441885140250179, 297.7992663317590427 ) ) ;
#41210=CARTESIAN_POINT ( 'NONE',  ( -12.29038035583180033, 1378.270906290520088, 210.0591904295070265 ) ) ;
#41220=ORIENTED_EDGE ( 'NONE', *, *, #4136, .F. ) ;
#41222=EDGE_CURVE ( 'NONE', #101083, #96085, #6154, .T. ) ;
#41230=CARTESIAN_POINT ( 'NONE',  ( -9.094257307190000361, 1384.874748762100126, 199.9429999480290121 ) ) ;
#41249=CARTESIAN_POINT ( 'NONE',  ( -105.6883447910000058, 1379.461008902830145, 304.2218452742590102 ) ) ;
#41254=CARTESIAN_POINT ( 'NONE',  ( -33.65891623492240115, 1384.565199592660065, 207.7968822506400102 ) ) ;
#41267=CARTESIAN_POINT ( 'NONE',  ( -68.77502866369999879, 1379.747951483830093, 280.1868250462589458 ) ) ;
#41284=DIRECTION ( 'NONE',  ( 1.836970198721029688E-16, 1.000000000000000000, -2.953460612019999929E-19 ) ) ;
#41287=DIRECTION ( 'NONE',  ( 1.000000000000000000, 0.000000000000000000, 0.000000000000000000 ) ) ;
#41313=B_SPLINE_CURVE_WITH_KNOTS ( 'NONE', 3,
 ( #38037, #62733, #29625, #55403, #37486, #29088, #27978, #63273, #98481, #2263, #28534, #96854, #63809 ),
 .UNSPECIFIED., .F., .F.,
 ( 4, 3, 3, 3, 4 ),
 ( 0.9322656447709229965, 0.9706014474725359609, 1.008994579606269815, 1.040095003257240025, 1.047387711740000116 ),
 .UNSPECIFIED. ) ;
#41325=CARTESIAN_POINT ( 'NONE',  ( -55.82031311308629995, 1383.802674022899964, 273.0220194663820052 ) ) ;
#41333=CARTESIAN_POINT ( 'NONE',  ( -67.77685405889999970, 1381.735381056040069, 263.8753344557590026 ) ) ;
#41343=CARTESIAN_POINT ( 'NONE',  ( -104.4199114259999845, 1380.436187834239945, 300.6363748219590093 ) ) ;
#41365=CARTESIAN_POINT ( 'NONE',  ( -105.9905438320000002, 1390.329878123639901, 307.5477013747590149 ) ) ;
#41396=CARTESIAN_POINT ( 'NONE',  ( -58.30576893479999967, 1384.922188666229886, 240.0674386386589845 ) ) ;
#41406=CARTESIAN_POINT ( 'NONE',  ( -10.97729220953150175, 1391.913060387059886, 205.9368150485350100 ) ) ;
#41420=ADVANCED_FACE ( 'NONE', ( #30997 ), #41983, .F. ) ;
#41429=CARTESIAN_POINT ( 'NONE',  ( -12.60774700310000007, 1379.062501030589829, 211.6870459648190206 ) ) ;
#41436=CARTESIAN_POINT ( 'NONE',  ( -10.00419192350000053, 1389.336578153429855, 201.7954106102789922 ) ) ;
#41442=CARTESIAN_POINT ( 'NONE',  ( -8.927662180601840802, 1384.337400639210045, 218.6377081841249890 ) ) ;
#41459=DIRECTION ( 'NONE',  ( 0.03206643377773112091, -0.01102865171324966288, 0.9994248909578780093 ) ) ;
#41472=FACE_BOUND ( 'NONE', #83855, .T. ) ;
#41482=CARTESIAN_POINT ( 'NONE',  ( -58.24912898052569687, 1385.052983837999818, 240.2872141092589970 ) ) ;
#41483=CARTESIAN_POINT ( 'NONE',  ( -11.38914589676969946, 1391.913060387289988, 211.4051490118059746 ) ) ;
#41493=CARTESIAN_POINT ( 'NONE',  ( -109.9783053820000021, 1384.541737252609892, 311.4424107222589555 ) ) ;
#41508=CARTESIAN_POINT ( 'NONE',  ( -68.60958769707259819, 1379.747566127410209, 280.2272292274159895 ) ) ;
#41509=ORIENTED_EDGE ( 'NONE', *, *, #47356, .T. ) ;
#41521=( LENGTH_UNIT ( ) NAMED_UNIT ( * ) SI_UNIT ( .MILLI., .METRE. ) );
#41544=CARTESIAN_POINT ( 'NONE',  ( -71.11512261416528702, 1384.744247007000013, 268.1821084325539459 ) ) ;
#41562=CARTESIAN_POINT ( 'NONE',  ( -62.06866934319999274, 1379.739831236870032, 266.3550163871590257 ) ) ;
#41612=CARTESIAN_POINT ( 'NONE',  ( -52.23114955023309847, 1384.729457832849903, 266.3052987280540265 ) ) ;
#41613=CARTESIAN_POINT ( 'NONE',  ( -106.8192835944930010, 1391.913060387289988, 302.1276685733210456 ) ) ;
#41619=CARTESIAN_POINT ( 'NONE',  ( -11.87852638355199808, 1378.094445099329278, 205.8387931305373684 ) ) ;
#41627=CARTESIAN_POINT ( 'NONE',  ( -12.05861758146710017, 1378.268530118770059, 211.6765750960350090 ) ) ;
#41640=CARTESIAN_POINT ( 'NONE',  ( -43.26295850523789710, 1379.661000266170049, 233.4033348232310061 ) ) ;
#41641=VERTEX_POINT ( 'NONE', #61750 ) ;
#41656=( LENGTH_UNIT ( ) NAMED_UNIT ( * ) SI_UNIT ( .MILLI., .METRE. ) );
#41673=CARTESIAN_POINT ( 'NONE',  ( -3.771520285720000309, 1380.389610323579973, 209.1218458698340044 ) ) ;
#41677=CARTESIAN_POINT ( 'NONE',  ( -104.1969030333949888, 1379.825940447170069, 304.0107167257339711 ) ) ;
#41696=CARTESIAN_POINT ( 'NONE',  ( -59.23393169420000248, 1385.069165163979960, 279.9259648821590645 ) ) ;
#41698=CARTESIAN_POINT ( 'NONE',  ( -43.88791476831470106, 1385.159211288639881, 249.3278255667920007 ) ) ;
#41706=CARTESIAN_POINT ( 'NONE',  ( -8.023003986910000052, 1384.895936019509918, 218.7875326659089978 ) ) ;
#41723=CARTESIAN_POINT ( 'NONE',  ( -109.5401826309999933, 1386.334633747299904, 297.2194470817590286 ) ) ;
#41753=CARTESIAN_POINT ( 'NONE',  ( -12.29890937187139954, 1378.335772002519889, 209.9648712015939793 ) ) ;
#41767=DIRECTION ( 'NONE',  ( -1.000000000000000000, 0.000000000000000000, 0.000000000000000000 ) ) ;
#41773=CARTESIAN_POINT ( 'NONE',  ( -7.978157731919999662, 1384.423773816979974, 199.5156531754190041 ) ) ;
#41796=CARTESIAN_POINT ( 'NONE',  ( -44.07146870577229691, 1384.596160883839957, 217.2312231507009983 ) ) ;
#41799=CARTESIAN_POINT ( 'NONE',  ( -107.1491673510000027, 1387.396471041590075, 310.3410155632590204 ) ) ;
#41806=CARTESIAN_POINT ( 'NONE',  ( -46.04389586920228794, 1379.678237767303244, 238.4312470573368898 ) ) ;
#41811=CARTESIAN_POINT ( 'NONE',  ( -68.30985499899999525, 1379.746831550510251, 279.0972868482590457 ) ) ;
#41841=PRODUCT_DEFINITION ( 'UNKNOWN', '', #94155, #54690 ) ;
#41865=CARTESIAN_POINT ( 'NONE',  ( -113.3764034147090882, 1381.413060387289988, 303.2221243954415968 ) ) ;
#41867=CARTESIAN_POINT ( 'NONE',  ( -66.54748892587809905, 1383.788754390270014, 290.5652759867210193 ) ) ;
#41870=CARTESIAN_POINT ( 'NONE',  ( -8.779116450932770377, 1385.568036331880194, 220.6413991625189794 ) ) ;
#41876=CARTESIAN_POINT ( 'NONE',  ( -49.19940419029999390, 1380.956237859229986, 255.4336207247589527 ) ) ;
#41887=CARTESIAN_POINT ( 'NONE',  ( -107.1082468550000044, 1381.675179291449922, 298.5714521776590118 ) ) ;
#41914=CARTESIAN_POINT ( 'NONE',  ( -105.5049133189999964, 1391.244241388860246, 305.3574306296589498 ) ) ;
#41922=CARTESIAN_POINT ( 'NONE',  ( -9.923943078109999760, 1386.701148096399947, 200.5013422001489687 ) ) ;
#41948=B_SPLINE_SURFACE_WITH_KNOTS ( 'NONE', 5, 5, ( 
 ( #47078, #73928, #99097, #39198, #54932, #56024 ),
 ( #107513, #73375, #30803, #64440, #22375, #108058 ),
 ( #90705, #98556, #72287, #90149, #63888, #29704 ),
 ( #31354, #99644, #22935, #82861, #12346, #13431 ),
 ( #38653, #105881, #6152, #29162, #63350, #97468 ),
 ( #47621, #46537, #98003, #106961, #80671, #21274 ) ),
 .UNSPECIFIED., .F., .F., .F.,
 ( 6, 6 ),
 ( 6, 6 ),
 ( -1.743397922130910115E-05, 7.850533482159220533 ),
 ( -1.743397922130910115E-05, 1.000000000000000000 ),
 .UNSPECIFIED. ) ;
#41964=CARTESIAN_POINT ( 'NONE',  ( -13.36456641330000039, 1385.300820372649923, 218.9430041755990146 ) ) ;
#41969=CIRCLE ( 'NONE', #104553, 1.999999997221749704 ) ;
#41974=CARTESIAN_POINT ( 'NONE',  ( -13.54127076360000004, 1379.893677090969959, 213.5390424406290037 ) ) ;
#41983=B_SPLINE_SURFACE_WITH_KNOTS ( 'NONE', 5, 5, ( 
 ( #97659, #56212, #81384, #38841, #90342, #29888 ),
 ( #55137, #82519, #107713, #99844, #57341, #14189 ),
 ( #4164, #64082, #5250, #14746, #3630, #12552 ),
 ( #80864, #39406, #99287, #72473, #56768, #106603 ),
 ( #98202, #21472, #5817, #89804, #16921, #42163 ),
 ( #75769, #102588, #8546, #74679, #33198, #92547 ),
 ( #48933, #15815, #16374, #84152, #100944, #85247 ),
 ( #59527, #7452, #109919, #50020, #67388, #25331 ),
 ( #24773, #50572, #25888, #75229, #76874, #58970 ) ),
 .UNSPECIFIED., .F., .F., .F.,
 ( 6, 3, 6 ),
 ( 6, 6 ),
 ( 1.461586381270000068, 8.269156193220000617, 13.54897587289999983 ),
 ( 0.000000000000000000, 1.000000000000000000 ),
 .UNSPECIFIED. ) ;
#41984=CARTESIAN_POINT ( 'NONE',  ( -10.51196183719999944, 1389.287104299670091, 202.3467939211689952 ) ) ;
#42003=CARTESIAN_POINT ( 'NONE',  ( -13.77020040508769938, 1383.859715768199976, 219.0313993434459690 ) ) ;
#42010=ORIENTED_EDGE ( 'NONE', *, *, #95410, .F. ) ;
#42016=CARTESIAN_POINT ( 'NONE',  ( -109.7178863559999940, 1384.903230390709950, 297.0861955617589842 ) ) ;
#42018=CARTESIAN_POINT ( 'NONE',  ( -5.931183514203220319, 1391.913060387289988, 203.1296912725950108 ) ) ;
#42028=CARTESIAN_POINT ( 'NONE',  ( -83.30886681774781266, 1385.170142578559989, 287.0534937087779781 ) ) ;
#42029=CARTESIAN_POINT ( 'NONE',  ( -11.66044326631700123, 1391.913060387289988, 209.8209183207389970 ) ) ;
#42053=CARTESIAN_POINT ( 'NONE',  ( -109.1344552622740025, 1384.804943809120005, 311.2633325561420179 ) ) ;
#42055=CARTESIAN_POINT ( 'NONE',  ( -68.71293640201129449, 1379.747782475320037, 280.3108351316460016 ) ) ;
#42069=SURFACE_STYLE_USAGE ( .BOTH. , #101947 ) ;
#42070=CARTESIAN_POINT ( 'NONE',  ( -12.74586014692540026, 1379.133382998009893, 208.7590490476249840 ) ) ;
#42083=CARTESIAN_POINT ( 'NONE',  ( -14.12838654810969885, 1379.942489218340143, 211.2222688814750029 ) ) ;
#42092=CARTESIAN_POINT ( 'NONE',  ( -12.16877406210000068, 1391.738014982129926, 211.0029804830490150 ) ) ;
#42093=CARTESIAN_POINT ( 'NONE',  ( -101.1025779375780047, 1384.877682633120003, 296.4583214505040587 ) ) ;
#42110=CARTESIAN_POINT ( 'NONE',  ( -63.99844030340000245, 1379.735010176050082, 270.2820024461590265 ) ) ;
#42114=CARTESIAN_POINT ( 'NONE',  ( -68.45261304034977456, 1379.747725225361137, 280.0177415625872186 ) ) ;
#42143=CARTESIAN_POINT ( 'NONE',  ( -9.817630982705171760, 1389.998136714420298, 216.6420858646567353 ) ) ;
#42160=CARTESIAN_POINT ( 'NONE',  ( -59.61913777331309916, 1384.697267862580020, 280.3101250345580411 ) ) ;
#42163=CARTESIAN_POINT ( 'NONE',  ( -106.5791719940000064, 1378.913060387289988, 301.6884094550590021 ) ) ;
#42168=CARTESIAN_POINT ( 'NONE',  ( -9.125244859669765063, 1381.433788410652596, 200.7127777233266954 ) ) ;
#42179=CARTESIAN_POINT ( 'NONE',  ( -12.83815065481509876, 1379.340893115409926, 211.5974809773499885 ) ) ;
#42192=CARTESIAN_POINT ( 'NONE',  ( -54.40028651508519886, 1379.725038095049968, 254.0986852477319928 ) ) ;
#42195=VERTEX_POINT ( 'NONE', #92159 ) ;
#42199=CARTESIAN_POINT ( 'NONE',  ( -106.8784014550000023, 1378.913059888100179, 307.4679267909590408 ) ) ;
#42225=CARTESIAN_POINT ( 'NONE',  ( -29.19545364349999872, 1375.228231664269970, 214.3784411298690031 ) ) ;
#42232=CARTESIAN_POINT ( 'NONE',  ( -105.5846808233909968, 1377.935441088430025, 304.0467934059079766 ) ) ;
#42252=CARTESIAN_POINT ( 'NONE',  ( -75.41155982419999759, 1386.723053008149918, 276.7375609186589713 ) ) ;
#42253=ORIENTED_EDGE ( 'NONE', *, *, #87706, .T. ) ;
#42254=CARTESIAN_POINT ( 'NONE',  ( -62.29399749175660617, 1385.055196683239956, 284.7151661488870218 ) ) ;
#42261=CARTESIAN_POINT ( 'NONE',  ( -8.581307216309999930, 1384.896522437119984, 218.6696871011889982 ) ) ;
#42263=CARTESIAN_POINT ( 'NONE',  ( -108.9612952299529951, 1383.599948435660053, 311.0484762934830201 ) ) ;
#42270=CARTESIAN_POINT ( 'NONE',  ( -121.0090375485666527, 1390.939237335599955, 306.1199062271713274 ) ) ;
#42276=CARTESIAN_POINT ( 'NONE',  ( -109.3312173139999999, 1385.266030154929922, 297.1495261968589716 ) ) ;
#42307=CARTESIAN_POINT ( 'NONE',  ( -12.30339481767540022, 1378.359469321360166, 209.9065742530260081 ) ) ;
#42328=DIRECTION ( 'NONE',  ( 1.000000000000000000, 0.000000000000000000, 0.000000000000000000 ) ) ;
#42349=CARTESIAN_POINT ( 'NONE',  ( -43.08576106324490240, 1384.592750897279984, 216.1018319972359905 ) ) ;
#42350=CARTESIAN_POINT ( 'NONE',  ( -14.49786657906220100, 1379.669926966970024, 208.2185517401169932 ) ) ;
#42356=CARTESIAN_POINT ( 'NONE',  ( -58.94826691570873578, 1379.722811456130103, 263.7298695812581855 ) ) ;
#42360=CARTESIAN_POINT ( 'NONE',  ( -68.56117685350000102, 1379.747432481730129, 279.6402102005590109 ) ) ;
#42377=CARTESIAN_POINT ( 'NONE',  ( 2.285841285774699520E-15, 1391.426148861440197, 209.1218459572589836 ) ) ;
#42390=CARTESIAN_POINT ( 'NONE',  ( -105.3229575393603028, 1390.872468168539399, 304.1992835431211120 ) ) ;
#42415=CARTESIAN_POINT ( 'NONE',  ( -61.13138140197489889, 1383.795200718170008, 282.5130783835299439 ) ) ;
#42420=ORIENTED_EDGE ( 'NONE', *, *, #31071, .F. ) ;
#42422=CARTESIAN_POINT ( 'NONE',  ( -55.58170576269999685, 1379.125231693479918, 252.4809319844590334 ) ) ;
#42427=FACE_OUTER_BOUND ( 'NONE', #36570, .T. ) ;
#42433=CARTESIAN_POINT ( 'NONE',  ( -109.4887233469999899, 1383.428478228959875, 297.2448718180590390 ) ) ;
#42436=CARTESIAN_POINT ( 'NONE',  ( 8.013264357029996177, 1375.413060387289988, 209.1218459572589836 ) ) ;
#42455=CARTESIAN_POINT ( 'NONE',  ( -105.2227265700000061, 1389.546011113689929, 307.5960479858590020 ) ) ;
#42486=EDGE_CURVE ( 'NONE', #26498, #107758, #38082, .T. ) ;
#42505=CARTESIAN_POINT ( 'NONE',  ( -8.835575458280001016, 1388.613171834459990, 217.0371058496990031 ) ) ;
#42514=CARTESIAN_POINT ( 'NONE',  ( -12.00629556859999880, 1378.345379175390008, 212.2149338467490054 ) ) ;
#42521=MECHANICAL_DESIGN_GEOMETRIC_PRESENTATION_REPRESENTATION('',(#47889),#6787);
#42522=EDGE_CURVE ( 'NONE', #71158, #82014, #103517, .T. ) ;
#42523=CARTESIAN_POINT ( 'NONE',  ( -12.55964041559999878, 1391.412561036180023, 208.3681481067449965 ) ) ;
#42524=EDGE_CURVE ( 'NONE', #83875, #96052, #34115, .T. ) ;
#42531=CARTESIAN_POINT ( 'NONE',  ( -9.128312996346709340, 1383.866482198609901, 218.5287380008880120 ) ) ;
#42561=CARTESIAN_POINT ( 'NONE',  ( -109.1645122539999875, 1384.901545528990027, 297.1326340414590277 ) ) ;
#42571=CARTESIAN_POINT ( 'NONE',  ( -109.0688921503400763, 1382.192801452487629, 310.8631491596341903 ) ) ;
#42574=CARTESIAN_POINT ( 'NONE',  ( -11.07525038950000074, 1391.808614258399984, 204.6545583908090009 ) ) ;
#42575=CARTESIAN_POINT ( 'NONE',  ( -68.65572861644470493, 1385.105512080379867, 263.0716478229380186 ) ) ;
#42576=CARTESIAN_POINT ( 'NONE',  ( -10.24890398481989884, 1391.913060387289988, 214.0452963765859806 ) ) ;
#42616=CARTESIAN_POINT ( 'NONE',  ( -12.65810595541850070, 1379.039847990219869, 208.8385753629780197 ) ) ;
#42639=CARTESIAN_POINT ( 'NONE',  ( -99.29130229444270128, 1384.871901381209909, 296.1281569486179706 ) ) ;
#42657=CARTESIAN_POINT ( 'NONE',  ( -51.90601367590000592, 1379.692123994150279, 243.6554138731589774 ) ) ;
#42679=DIRECTION ( 'NONE',  ( -1.000000000000000000, 0.000000000000000000, 0.000000000000000000 ) ) ;
#42696=CARTESIAN_POINT ( 'NONE',  ( -9.484515027067567772, 1389.595169172901706, 217.0780171008755701 ) ) ;
#42713=CARTESIAN_POINT ( 'NONE',  ( -11.19935784055662786, 1391.089543242234640, 214.3845051435474716 ) ) ;
#42716=CARTESIAN_POINT ( 'NONE',  ( -79.56500322749430154, 1384.639486651150037, 303.5682780263990139 ) ) ;
#42731=CARTESIAN_POINT ( 'NONE',  ( -9.459903729319998789, 1382.054661141809902, 200.9046470295689915 ) ) ;
#42743=CARTESIAN_POINT ( 'NONE',  ( -54.44063311709999908, 1379.743533640540136, 254.0790799858589821 ) ) ;
#42749=CARTESIAN_POINT ( 'NONE',  ( -107.2899035190000063, 1379.886884136000162, 309.1794862632590366 ) ) ;
#42776=CARTESIAN_POINT ( 'NONE',  ( -47.10178971561379768, 1379.678077506135423, 234.1671279625103637 ) ) ;
#42782=CARTESIAN_POINT ( 'NONE',  ( -105.0405218166850005, 1379.391193415470070, 304.9871214168560414 ) ) ;
#42795=B_SPLINE_SURFACE_WITH_KNOTS ( 'NONE', 5, 5, ( 
 ( #44925, #29196, #26996, #28090, #80148, #105357 ),
 ( #62277, #105917, #61186, #96408, #95303, #46020 ),
 ( #104252, #18563, #63386, #45477, #3469, #19684 ),
 ( #62852, #78505, #20229, #52758, #79620, #86892 ),
 ( #2924, #10186, #28648, #27542, #61725, #95847 ),
 ( #19114, #53317, #59240, #83312, #92813, #31253 ) ),
 .UNSPECIFIED., .F., .F., .F.,
 ( 6, 6 ),
 ( 6, 6 ),
 ( -0.0003633979984830099813, 1.546630684984659831 ),
 ( 0.000000000000000000, 2.000363398052620312 ),
 .UNSPECIFIED. ) ;
#42804=CARTESIAN_POINT ( 'NONE',  ( -43.09011427770000324, 1385.164419251190111, 247.5010251099589880 ) ) ;
#42806=CARTESIAN_POINT ( 'NONE',  ( -67.78301067296590077, 1385.032250548179945, 292.4443811870189620 ) ) ;
#42818=CARTESIAN_POINT ( 'NONE',  ( -108.1388787236599995, 1383.031276538240036, 310.7739520621719862 ) ) ;
#42847=EDGE_CURVE ( 'NONE', #103478, #96085, #23395, .T. ) ;
#42848=EDGE_CURVE ( 'NONE', #101083, #49944, #81920, .T. ) ;
#42870=CARTESIAN_POINT ( 'NONE',  ( -12.30740102227800215, 1378.372698618640015, 209.8468845047000002 ) ) ;
#42890=DIRECTION ( 'NONE',  ( 0.000000000000000000, 0.000000000000000000, 1.000000000000000000 ) ) ;
#42909=CARTESIAN_POINT ( 'NONE',  ( -109.5441724509999943, 1376.937034645699896, 301.4143085365590196 ) ) ;
#42917=CARTESIAN_POINT ( 'NONE',  ( -48.07998102645539973, 1384.611432322939891, 222.4239625009780070 ) ) ;
#42924=CARTESIAN_POINT ( 'NONE',  ( -46.82776862987225996, 1379.681009986248000, 239.8345724582786431 ) ) ;
#42929=CARTESIAN_POINT ( 'NONE',  ( -68.68762034649999748, 1379.747740914639962, 279.9560673389590306 ) ) ;
#42936=CARTESIAN_POINT ( 'NONE',  ( -67.04318418450000649, 1385.033547286170005, 292.1847026260589928 ) ) ;
#42938=CARTESIAN_POINT ( 'NONE',  ( -105.0581303879369983, 1379.236400313860031, 304.0328620142400382 ) ) ;
#42957=CARTESIAN_POINT ( 'NONE',  ( -109.1309839890330124, 1384.924126711810004, 311.2646841801559958 ) ) ;
#42982=CARTESIAN_POINT ( 'NONE',  ( -73.85600498739088948, 1383.781764016229999, 298.7751872343750392 ) ) ;
#42990=CIRCLE ( 'NONE', #44842, 2.500000000000002220 ) ;
#42991=CARTESIAN_POINT ( 'NONE',  ( -64.53155199309999546, 1384.701788983860297, 254.0354793386590018 ) ) ;
#43003=CARTESIAN_POINT ( 'NONE',  ( -108.9897655200000059, 1383.709197802749941, 297.2975670400589934 ) ) ;
#43025=CARTESIAN_POINT ( 'NONE',  ( -105.9466775579999904, 1388.732462752959918, 308.9851393517590168 ) ) ;
#43034=CARTESIAN_POINT ( 'NONE',  ( -9.082734998440001206, 1385.203252519110038, 199.9450228470490174 ) ) ;
#43062=CARTESIAN_POINT ( 'NONE',  ( -11.49929945651590124, 1391.913060387289988, 207.6743836541510007 ) ) ;
#43074=CARTESIAN_POINT ( 'NONE',  ( -7.129176379223929955E-16, 1388.284644706179961, 200.7336192388889913 ) ) ;
#43083=CARTESIAN_POINT ( 'NONE',  ( -10.76474969630000089, 1381.207448912699874, 216.6668544953589901 ) ) ;
#43089=CARTESIAN_POINT ( 'NONE',  ( -11.20926149449999976, 1388.118472602389829, 201.8648932818790058 ) ) ;
#43107=B_SPLINE_CURVE_WITH_KNOTS ( 'NONE', 3,
 ( #107928, #90018, #106279, #54792, #88924, #81071, #21138, #72162, #4915, #31221, #30672, #47488, #90570, #3853, #106816, #3299 ),
 .UNSPECIFIED., .F., .F.,
 ( 4, 3, 3, 3, 3, 4 ),
 ( -5.332638707570000136, -5.312294071160000186, -5.120178322282729511, -4.857691371485320708, -4.648885627528850151, -4.382742598909070253 ),
 .UNSPECIFIED. ) ;
#43119=LINE ( 'NONE', #27404, #23515 ) ;
#43124=CARTESIAN_POINT ( 'NONE',  ( -109.5352543199999928, 1384.892772668599946, 297.1231677395590509 ) ) ;
#43127=CARTESIAN_POINT ( 'NONE',  ( -14.46044090995190068, 1380.092572431659846, 208.8609369278819941 ) ) ;
#43130=EDGE_CURVE ( 'NONE', #60994, #69449, #56734, .T. ) ;
#43132=CARTESIAN_POINT ( 'NONE',  ( -109.6086345746109885, 1383.178240054900016, 311.2147542219479988 ) ) ;
#43135=CARTESIAN_POINT ( 'NONE',  ( -11.67738853530000043, 1391.388800472150251, 205.1463387926490043 ) ) ;
#43136=CARTESIAN_POINT ( 'NONE',  ( -73.46128287683579572, 1385.129171348790123, 272.7076196986540140 ) ) ;
#43144=DIRECTION ( 'NONE',  ( -0.9997613315435491810, 0.000000000000000000, 0.02184673774890954004 ) ) ;
#43178=CARTESIAN_POINT ( 'NONE',  ( -12.31949146158819985, 1378.253793448930082, 209.5105130821430066 ) ) ;
#43191=AXIS2_PLACEMENT_3D ( 'NONE', #58157, #27168, #61352 ) ;
#43192=CARTESIAN_POINT ( 'NONE',  ( -14.17879220992960043, 1380.120661394760191, 210.8840528948799999 ) ) ;
#43198=CARTESIAN_POINT ( 'NONE',  ( -12.43710052089999962, 1391.584050381710085, 209.7498261801929971 ) ) ;
#43200=CARTESIAN_POINT ( 'NONE',  ( -106.7956374490409956, 1384.894787335530054, 297.0320324003700421 ) ) ;
#43205=ORIENTED_EDGE ( 'NONE', *, *, #70155, .T. ) ;
#43220=CARTESIAN_POINT ( 'NONE',  ( -21.09588753150000073, 1379.716440018399908, 209.7902992619769975 ) ) ;
#43244=CARTESIAN_POINT ( 'NONE',  ( -109.5177468959999914, 1385.290589466009806, 297.1412373070589865 ) ) ;
#43273=CARTESIAN_POINT ( 'NONE',  ( -78.73633071742699485, 1384.641256474020111, 302.9908934104659579 ) ) ;
#43274=CARTESIAN_POINT ( 'NONE',  ( -26.53150723579640058, 1384.962365308560038, 203.8867581072389896 ) ) ;
#43292=CARTESIAN_POINT ( 'NONE',  ( -8.755267316439999448, 1383.867798405919984, 200.0220800673290000 ) ) ;
#43305=CARTESIAN_POINT ( 'NONE',  ( -60.17131492770970169, 1379.724567624519977, 265.9736432342079411 ) ) ;
#43314=FACE_OUTER_BOUND ( 'NONE', #60348, .T. ) ;
#43315=DIRECTION ( 'NONE',  ( -0.04204747460233849293, 7.723995777597519186E-18, -0.9991156138703697343 ) ) ;
#43318=AXIS2_PLACEMENT_3D ( 'NONE', #110479, #99855, #109934 ) ;
#43339=EDGE_CURVE ( 'NONE', #46370, #77278, #47539, .T. ) ;
#43341=CARTESIAN_POINT ( 'NONE',  ( -48.76121443664156629, 1379.684058018070345, 237.2045636776436481 ) ) ;
#43343=ORIENTED_EDGE ( 'NONE', *, *, #91070, .F. ) ;
#43346=CARTESIAN_POINT ( 'NONE',  ( -104.5195930981980013, 1379.736861869120048, 305.0059150852220000 ) ) ;
#43355=EDGE_CURVE ( 'NONE', #36205, #61114, #83759, .T. ) ;
#43356=CARTESIAN_POINT ( 'NONE',  ( -102.7392963879999996, 1384.315214695209761, 311.1957061252590506 ) ) ;
#43364=CARTESIAN_POINT ( 'NONE',  ( -121.2674250099716460, 1379.886883438980021, 304.3447484988897145 ) ) ;
#43368=CARTESIAN_POINT ( 'NONE',  ( -78.77145090140000150, 1390.626937550559887, 293.5766517498590247 ) ) ;
#43370=CARTESIAN_POINT ( 'NONE',  ( -62.62830543184530541, 1385.053670896650146, 285.2368784993579993 ) ) ;
#43379=CARTESIAN_POINT ( 'NONE',  ( -109.2945710968669886, 1382.750670875540209, 311.0281563818350037 ) ) ;
#43407=CARTESIAN_POINT ( 'NONE',  ( -12.45123913023140005, 1384.883862109669963, 219.0084378725689760 ) ) ;
#43410=B_SPLINE_CURVE_WITH_KNOTS ( 'NONE', 3,
 ( #78899, #18394, #19511, #60442, #79442, #44187, #28481, #96795, #20065, #37984, #22244, #73238, #48036, #12214, #82174, #56442, #88928, #99512, #106283, #71632, #5474, #39058, #72166 ),
 .UNSPECIFIED., .F., .F.,
 ( 4, 2, 2, 1, 2, 2, 2, 2, 2, 2, 2, 4 ),
 ( 0.000000000000000000, 0.1249999999995614064, 0.1874999999993859079, 0.2187499999992296718, 0.2343749999991104338, 0.2499999999989912236, 0.3749999999990175081, 0.4374999999990306643, 0.4999999999990438759, 0.6249999999993142152, 0.7499999999995846656, 1.000000000000000000 ),
 .UNSPECIFIED. ) ;
#43426=CARTESIAN_POINT ( 'NONE',  ( -109.9711626006150027, 1384.465720048490084, 311.4368156476579657 ) ) ;
#43442=CARTESIAN_POINT ( 'NONE',  ( -8.629930135849999573, 1384.437861499620112, 199.9043374725989963 ) ) ;
#43463=CARTESIAN_POINT ( 'NONE',  ( -105.7600639359999946, 1378.531805229619977, 302.0293825393590055 ) ) ;
#43465=CARTESIAN_POINT ( 'NONE',  ( -106.5231981154489915, 1378.913060387289988, 301.8480351107359638 ) ) ;
#43470=CARTESIAN_POINT ( 'NONE',  ( -68.71261127229999488, 1384.854887445129862, 263.4295281439590326 ) ) ;
#43471=CARTESIAN_POINT ( 'NONE',  ( -56.07122076218969653, 1384.649968191290100, 235.9257209178720132 ) ) ;
#43484=CARTESIAN_POINT ( 'NONE',  ( -68.47455138450000334, 1379.747378330220045, 279.4267273018589890 ) ) ;
#43486=LINE ( 'NONE', #1482, #3868 ) ;
#43492=CARTESIAN_POINT ( 'NONE',  ( -73.55347204870000155, 1384.772439966069896, 298.9553539304589549 ) ) ;
#43509=EDGE_LOOP ( 'NONE', ( #58565, #16121, #28617, #14370, #99889, #46253 ) ) ;
#43536=CARTESIAN_POINT ( 'NONE',  ( -65.85453692722450114, 1383.789513244699947, 289.6320689311420438 ) ) ;
#43543=CARTESIAN_POINT ( 'NONE',  ( -89.15684587290000707, 1384.835666735910081, 292.2581851215589950 ) ) ;
#43553=CARTESIAN_POINT ( 'NONE',  ( -108.4836655010000186, 1381.983168677669937, 297.9253098464590153 ) ) ;
#43569=CARTESIAN_POINT ( 'NONE',  ( -8.862056518773441027, 1384.892951007370129, 218.6851137863439760 ) ) ;
#43575=CARTESIAN_POINT ( 'NONE',  ( -106.2139324000000045, 1390.828638221579922, 307.6609436900590140 ) ) ;
#43582=ORIENTED_EDGE ( 'NONE', *, *, #4893, .T. ) ;
#43626=CARTESIAN_POINT ( 'NONE',  ( -4.265932623502749891E-16, 1391.052076539619975, 208.7094039267549874 ) ) ;
#43635=CARTESIAN_POINT ( 'NONE',  ( -9.949232747880000005, 1381.968568543130004, 217.5033713529390127 ) ) ;
#43640=CARTESIAN_POINT ( 'NONE',  ( -11.15555666070000029, 1388.626024522959824, 202.3683382543690072 ) ) ;
#43660=CARTESIAN_POINT ( 'NONE',  ( -12.94530514837170010, 1383.860467683670095, 218.9034580252159969 ) ) ;
#43669=CARTESIAN_POINT ( 'NONE',  ( -9.851472566700000044, 1384.510545767029953, 199.8981574268189831 ) ) ;
#43676=CARTESIAN_POINT ( 'NONE',  ( -11.89318647318120092, 1391.758398471429928, 212.5295707731389996 ) ) ;
#43680=CARTESIAN_POINT ( 'NONE',  ( -107.8451728718519718, 1380.542607501936118, 309.8189202647981233 ) ) ;
#43682=CARTESIAN_POINT ( 'NONE',  ( -12.91238682329999854, 1379.507757257049889, 211.2365369345390036 ) ) ;
#43683=CARTESIAN_POINT ( 'NONE',  ( -12.30988125380000042, 1391.742651319489823, 209.2308626440040200 ) ) ;
#43684=CARTESIAN_POINT ( 'NONE',  ( -79.74802494709490475, 1385.156543383609915, 282.7772545974189597 ) ) ;
#43686=CARTESIAN_POINT ( 'NONE',  ( -19.04120737539122388, 1379.714756628304485, 209.1757808297589918 ) ) ;
#43721=CARTESIAN_POINT ( 'NONE',  ( -12.38376459812810104, 1378.578895824120082, 209.2319221572759886 ) ) ;
#43738=AXIS2_PLACEMENT_3D ( 'NONE', #6389, #75803, #31579 ) ;
#43745=CARTESIAN_POINT ( 'NONE',  ( -96.21043572509938713, 1384.861607426979845, 295.3416321102220081 ) ) ;
#43749=VERTEX_POINT ( 'NONE', #82928 ) ;
#43760=CARTESIAN_POINT ( 'NONE',  ( -110.0634901748029932, 1384.899971912700039, 296.9512050915229793 ) ) ;
#43762=CARTESIAN_POINT ( 'NONE',  ( -37.86125039060000574, 1379.639043232470158, 220.5631543556590088 ) ) ;
#43766=CARTESIAN_POINT ( 'NONE',  ( -68.77278092737650184, 1379.747928288920093, 280.3133413970129482 ) ) ;
#43817=CARTESIAN_POINT ( 'NONE',  ( -80.39701180146140302, 1384.637746234069937, 304.1167271054749790 ) ) ;
#43824=CARTESIAN_POINT ( 'NONE',  ( -8.156454811679999750, 1384.924237574090057, 199.6468110712790178 ) ) ;
#43837=CARTESIAN_POINT ( 'NONE',  ( -13.48418208170959964, 1379.644826002420132, 211.5188789427980112 ) ) ;
#43849=CARTESIAN_POINT ( 'NONE',  ( -62.66283327366161160, 1379.734827332920077, 270.6325249849410284 ) ) ;
#43857=CARTESIAN_POINT ( 'NONE',  ( -7.791194074889999932, 1385.469146237939867, 218.8820831402890121 ) ) ;
#43882=CARTESIAN_POINT ( 'NONE',  ( -48.22222548969896394, 1379.682101389173340, 236.1980132620304289 ) ) ;
#43887=ORIENTED_EDGE ( 'NONE', *, *, #9792, .F. ) ;
#43898=CARTESIAN_POINT ( 'NONE',  ( -109.9987472819999965, 1383.757409383979848, 311.0847451122589860 ) ) ;
#43912=CARTESIAN_POINT ( 'NONE',  ( -82.03511417020000351, 1389.474284752290032, 290.2139668048590124 ) ) ;
#43922=CARTESIAN_POINT ( 'NONE',  ( -109.0942519332729859, 1382.194178918040052, 310.8938292817809952 ) ) ;
#43954=CARTESIAN_POINT ( 'NONE',  ( -18.21186767409350082, 1384.867739624789920, 220.2868233047339857 ) ) ;
#43960=VERTEX_POINT ( 'NONE', #103445 ) ;
#43978=CARTESIAN_POINT ( 'NONE',  ( -101.6919322582379976, 1379.485316433199841, 304.9628827255460237 ) ) ;
#43993=CARTESIAN_POINT ( 'NONE',  ( -8.389212874609999204, 1384.445125336340197, 199.8059234258990102 ) ) ;
#44013=CARTESIAN_POINT ( 'NONE',  ( -72.27662900180000349, 1379.712643070530021, 284.7775436246590175 ) ) ;
#44020=CARTESIAN_POINT ( 'NONE',  ( -89.15725962140000149, 1385.072235092599840, 292.2573307935589924 ) ) ;
#44021=CARTESIAN_POINT ( 'NONE',  ( -58.46619516613409928, 1384.663721486439954, 240.7616066048800008 ) ) ;
#44028=ADVANCED_FACE ( 'NONE', ( #1573 ), #78410, .T. ) ;
#44031=CARTESIAN_POINT ( 'NONE',  ( -68.54762064409999311, 1379.747581803159846, 279.6462198773589876 ) ) ;
#44039=CARTESIAN_POINT ( 'NONE',  ( -25.94961989419999782, 1385.251886777470190, 224.2307850120589876 ) ) ;
#44041=CARTESIAN_POINT ( 'NONE',  ( -11.90445094143569982, 1385.305240112880028, 218.9163558013920010 ) ) ;
#44089=CARTESIAN_POINT ( 'NONE',  ( -97.16214200120590760, 1383.765811092889862, 310.2586638610929413 ) ) ;
#44096=CARTESIAN_POINT ( 'NONE',  ( -62.63809935099999393, 1382.333481460739904, 284.4251248683589779 ) ) ;
#44110=CARTESIAN_POINT ( 'NONE',  ( -109.4610122139999930, 1384.463034823889984, 297.1307535903590065 ) ) ;
#44141=CARTESIAN_POINT ( 'NONE',  ( -9.216856378879999312, 1385.697103985929971, 200.0334226857090130 ) ) ;
#44170=CARTESIAN_POINT ( 'NONE',  ( -11.67229379317850047, 1391.913060387289988, 209.5769804851749996 ) ) ;
#44174=ORIENTED_EDGE ( 'NONE', *, *, #2886, .T. ) ;
#44182=CARTESIAN_POINT ( 'NONE',  ( -4.649084002151809292E-16, 1389.634744113780243, 202.9789274992690196 ) ) ;
#44187=CARTESIAN_POINT ( 'NONE',  ( -14.04273730155982847, 1379.586150356219150, 211.8481849348019921 ) ) ;
#44190=DIRECTION ( 'NONE',  ( -1.000000000000000000, 0.000000000000000000, 0.000000000000000000 ) ) ;
#44191=CARTESIAN_POINT ( 'NONE',  ( -9.137732587340000379, 1383.146477076719975, 218.2898102310589934 ) ) ;
#44220=CARTESIAN_POINT ( 'NONE',  ( -14.04325441188020207, 1383.859464698529791, 219.0769673503140211 ) ) ;
#44229=CARTESIAN_POINT ( 'NONE',  ( -9.104488441191636028, 1388.370946186080118, 200.6891223300711431 ) ) ;
#44235=CARTESIAN_POINT ( 'NONE',  ( -14.42899799073379974, 1380.189325286879921, 209.0990684340630139 ) ) ;
#44241=CONICAL_SURFACE ( 'NONE', #110411, 12.49999999999999467, 0.02617993877989872875 ) ;
#44243=CARTESIAN_POINT ( 'NONE',  ( -12.46299153120000014, 1391.583714740810137, 209.2286840156340020 ) ) ;
#44244=CARTESIAN_POINT ( 'NONE',  ( -76.82411996085400574, 1385.144362471309933, 278.4876237131520043 ) ) ;
#44247=CARTESIAN_POINT ( 'NONE',  ( -65.30777065759998834, 1379.749275567730137, 273.2377066393590326 ) ) ;
#44306=CARTESIAN_POINT ( 'NONE',  ( -97.97730939973499176, 1384.867588345430022, 295.8314372660599929 ) ) ;
#44312=CARTESIAN_POINT ( 'NONE',  ( -9.129808743239919977, 1383.863787745319996, 218.5279288296370055 ) ) ;
#44321=CARTESIAN_POINT ( 'NONE',  ( -104.3158487040000040, 1389.466353268959892, 300.6607691406589993 ) ) ;
#44324=CARTESIAN_POINT ( 'NONE',  ( -25.92022873519999848, 1379.720561049090065, 211.6907041564289784 ) ) ;
#44329=CARTESIAN_POINT ( 'NONE',  ( -68.66492675561440251, 1379.747814238210822, 280.2579952115759170 ) ) ;
#44347=DIRECTION ( 'NONE',  ( 0.02617694830785712717, 0.9996573249755577040, -1.162479441679614436E-17 ) ) ;
#44357=DIRECTION ( 'NONE',  ( -0.9998780035959983215, 8.712314624148121749E-33, 0.01561979272847786350 ) ) ;
#44368=CARTESIAN_POINT ( 'NONE',  ( -7.686381689219429880, 1383.591223628860007, 218.9353989820789934 ) ) ;
#44382=CARTESIAN_POINT ( 'NONE',  ( -72.88182616411249626, 1384.654869595349965, 298.0902554268950553 ) ) ;
#44383=CARTESIAN_POINT ( 'NONE',  ( -9.094910673856409389, 1384.931050598509955, 199.9427862989620053 ) ) ;
#44401=CARTESIAN_POINT ( 'NONE',  ( -10.73113664029999903, 1382.357287394640252, 201.1356155892590039 ) ) ;
#44413=CARTESIAN_POINT ( 'NONE',  ( -63.24753723578009357, 1379.733506366819938, 271.8172255436770115 ) ) ;
#44420=CARTESIAN_POINT ( 'NONE',  ( -109.8253978320000073, 1384.918090075649843, 311.3807729152589445 ) ) ;
#44443=CARTESIAN_POINT ( 'NONE',  ( -35.41186141649757246, 1379.641460143238646, 218.3720869345321489 ) ) ;
#44472=CARTESIAN_POINT ( 'NONE',  ( -96.71789436439999577, 1389.284422085869892, 307.9725871335590455 ) ) ;
#44483=CARTESIAN_POINT ( 'NONE',  ( -105.7656562948000101, 1380.972838942760063, 308.6606380284670195 ) ) ;
#44500=DIRECTION ( 'NONE',  ( 1.000000000000000000, 0.000000000000000000, 0.000000000000000000 ) ) ;
#44509=CARTESIAN_POINT ( 'NONE',  ( -14.54449344532160104, 1384.878238794750132, 219.3450228996460112 ) ) ;
#44534=CARTESIAN_POINT ( 'NONE',  ( -113.4000000000000057, 1379.413087040579967, 305.1680626132370548 ) ) ;
#44546=CARTESIAN_POINT ( 'NONE',  ( -8.179930528059999872, 1384.351712228729866, 199.6861502166489970 ) ) ;
#44564=CARTESIAN_POINT ( 'NONE',  ( -84.31096497629998510, 1374.600296256690172, 298.0935392271590558 ) ) ;
#44567=EDGE_CURVE ( 'NONE', #67802, #26163, #3327, .T. ) ;
#44573=CARTESIAN_POINT ( 'NONE',  ( -92.78423182619999920, 1385.084188629489972, 294.1460543437590331 ) ) ;
#44575=CARTESIAN_POINT ( 'NONE',  ( -52.84305079022620077, 1384.633012693340106, 229.9587693130270054 ) ) ;
#44582=CARTESIAN_POINT ( 'NONE',  ( -27.74315420650000164, 1383.844892876249787, 225.5041886164589755 ) ) ;
#44587=CARTESIAN_POINT ( 'NONE',  ( -67.63612853559999394, 1379.748709736400087, 277.8550023105590299 ) ) ;
#44588=CARTESIAN_POINT ( 'NONE',  ( -109.9850573467474106, 1384.919979545036085, 311.4561262142244686 ) ) ;
#44593=CARTESIAN_POINT ( 'NONE',  ( -7.965680540240001051, 1384.926148861439970, 199.4891222871690104 ) ) ;
#44596=CARTESIAN_POINT ( 'NONE',  ( -22.68470003930000090, 1385.128694769440017, 222.0359864906590133 ) ) ;
#44598=CARTESIAN_POINT ( 'NONE',  ( -14.01427947078130032, 1385.298181900520149, 219.2221585896700162 ) ) ;
#44616=ORIENTED_EDGE ( 'NONE', *, *, #101505, .F. ) ;
#44647=CARTESIAN_POINT ( 'NONE',  ( -88.89087977607839264, 1383.771024000470106, 308.1318186344960282 ) ) ;
#44648=CARTESIAN_POINT ( 'NONE',  ( -109.3980338099009941, 1384.227017930330021, 311.2250570124659816 ) ) ;
#44650=DIRECTION ( 'NONE',  ( -0.8090169943751894799, 3.009330011589934659E-31, -0.5877852522921398482 ) ) ;
#44656=CARTESIAN_POINT ( 'NONE',  ( -77.33784092209999983, 1381.010457831459917, 299.7574715306590178 ) ) ;
#44667=CARTESIAN_POINT ( 'NONE',  ( -109.0924835130000048, 1382.770673418189972, 297.4849455732589831 ) ) ;
#44733=CARTESIAN_POINT ( 'NONE',  ( -11.67615777976660141, 1391.913060387279984, 209.2633225133189967 ) ) ;
#44743=CARTESIAN_POINT ( 'NONE',  ( -46.14048177419999774, 1390.858208826580039, 234.9404857890590108 ) ) ;
#44752=CARTESIAN_POINT ( 'NONE',  ( -8.270195822719999867, 1382.590927455500150, 218.4495833107989995 ) ) ;
#44781=CARTESIAN_POINT ( 'NONE',  ( -34.81854416728349833, 1383.835731978919966, 233.6493107493720061 ) ) ;
#44789=FACE_OUTER_BOUND ( 'NONE', #78662, .T. ) ;
#44795=CARTESIAN_POINT ( 'NONE',  ( -12.36595038414849945, 1391.700200887409892, 209.7453690616009965 ) ) ;
#44804=CARTESIAN_POINT ( 'NONE',  ( -101.4799880583079954, 1385.224571067029956, 296.5271061909010086 ) ) ;
#44811=CARTESIAN_POINT ( 'NONE',  ( -113.4000000000000057, 1384.913060387289988, 304.2218459572590064 ) ) ;
#44842=AXIS2_PLACEMENT_3D ( 'NONE', #63692, #98359, #79923 ) ;
#44888=CARTESIAN_POINT ( 'NONE',  ( -32.53397683490000247, 1379.726329037039932, 216.1069825312089847 ) ) ;
#44892=CARTESIAN_POINT ( 'NONE',  ( -67.84113287130467995, 1379.747601269228880, 279.1899061518716394 ) ) ;
#44901=CARTESIAN_POINT ( 'NONE',  ( -9.094129269030000629, 1384.954944735329946, 199.9429221374590213 ) ) ;
#44925=CARTESIAN_POINT ( 'NONE',  ( -12.23665942925899941, 1377.661379157180136, 207.7791151321639802 ) ) ;
#44944=CARTESIAN_POINT ( 'NONE',  ( -60.29191067893739842, 1384.694631598589922, 281.4556533462259722 ) ) ;
#44945=CARTESIAN_POINT ( 'NONE',  ( -42.22056685433029344, 1384.995465601839896, 215.1295050435799965 ) ) ;
#44951=CARTESIAN_POINT ( 'NONE',  ( -8.371438403939999162, 1384.922510205190065, 199.7749754636789987 ) ) ;
#44952=CARTESIAN_POINT ( 'NONE',  ( -106.4020496450190052, 1391.913060387289988, 304.2007955189830568 ) ) ;
#44958=CARTESIAN_POINT ( 'NONE',  ( -106.9324727664809984, 1391.913060387289988, 306.5339839144160123 ) ) ;
#44962=CARTESIAN_POINT ( 'NONE',  ( -8.407515995729999858, 1383.335842388670017, 199.9217961407289863 ) ) ;
#44974=CARTESIAN_POINT ( 'NONE',  ( -65.84351248663899980, 1379.744198721029989, 276.1294122088469862 ) ) ;
#44987=CARTESIAN_POINT ( 'NONE',  ( -105.9555828394970121, 1378.913060388860004, 305.1986518409329960 ) ) ;
#45005=CARTESIAN_POINT ( 'NONE',  ( -8.862244220539999162, 1384.927755921120252, 218.6851219245690174 ) ) ;
#45007=AXIS2_PLACEMENT_3D ( 'NONE', #11987, #37195, #87605 ) ;
#45008=CARTESIAN_POINT ( 'NONE',  ( -12.34597541399999976, 1378.750906298520249, 209.0838709649310090 ) ) ;
#45009=CARTESIAN_POINT ( 'NONE',  ( -16.42994098213877052, 1379.596574317858085, 208.1847039279784610 ) ) ;
#45011=ADVANCED_FACE ( 'NONE', ( #43314 ), #3441, .F. ) ;
#45022=CARTESIAN_POINT ( 'NONE',  ( -58.33642492515414091, 1379.720901747983589, 262.5133912307817923 ) ) ;
#45041=CARTESIAN_POINT ( 'NONE',  ( -98.33257935689999840, 1389.446463678290229, 299.1634636375590048 ) ) ;
#45053=CARTESIAN_POINT ( 'NONE',  ( -104.0132077409040079, 1379.986693862269931, 305.5692602416439740 ) ) ;
#45079=CARTESIAN_POINT ( 'NONE',  ( -19.79605902738999745, 1384.862938669949926, 220.8639557539960094 ) ) ;
#45104=CARTESIAN_POINT ( 'NONE',  ( -105.6573924705229928, 1379.461035556120123, 305.1680620773340138 ) ) ;
#45133=CARTESIAN_POINT ( 'NONE',  ( -68.69226509189999774, 1374.746858117589909, 280.5557816734590233 ) ) ;
#45146=CARTESIAN_POINT ( 'NONE',  ( -5.958828918610000080, 1384.900097640590047, 218.5255276338789940 ) ) ;
#45152=CARTESIAN_POINT ( 'NONE',  ( -67.42914565080000955, 1379.745493734729962, 277.3807740811590179 ) ) ;
#45160=CARTESIAN_POINT ( 'NONE',  ( -27.62871390899999824, 1385.108881161949967, 225.6286099116589980 ) ) ;
#45162=CARTESIAN_POINT ( 'NONE',  ( -19.80402451206670023, 1385.277035965169944, 220.8433670724960223 ) ) ;
#45204=CARTESIAN_POINT ( 'NONE',  ( -78.94690149131609758, 1383.777751329849934, 302.9268705869330347 ) ) ;
#45207=DIRECTION ( 'NONE',  ( 1.836970198721029688E-16, 1.000000000000000000, 0.000000000000000000 ) ) ;
#45213=CARTESIAN_POINT ( 'NONE',  ( -67.18675499840000498, 1383.787653363379832, 292.0788269227589922 ) ) ;
#45267=ADVANCED_FACE ( 'NONE', ( #73134 ), #92099, .T. ) ;
#45285=CARTESIAN_POINT ( 'NONE',  ( -11.67285302236730082, 1391.913060387249971, 209.1401477369450106 ) ) ;
#45293=B_SPLINE_CURVE_WITH_KNOTS ( 'NONE', 3,
 ( #105891, #29172, #63361, #91684, #52463, #101167, #60304, #67609, #92784, #16059, #86593, #17143, #78192, #9885, #101719, #94424, #35086, #102282, #32871, #58650, #76537, #9342 ),
 .UNSPECIFIED., .F., .F.,
 ( 4, 3, 3, 3, 3, 3, 3, 4 ),
 ( 10.04884080650000122, 10.05925814240000093, 10.16601929647930014, 10.29502131698899881, 10.44078577034700039, 10.52123097808229879, 10.70418225783430088, 10.99321056540000008 ),
 .UNSPECIFIED. ) ;
#45296=CARTESIAN_POINT ( 'NONE',  ( -37.19866254769999614, 1386.636863995749991, 210.1929157112890039 ) ) ;
#45306=CARTESIAN_POINT ( 'NONE',  ( -8.700971975899999933, 1381.863705729429967, 218.0542239465389969 ) ) ;
#45336=CARTESIAN_POINT ( 'NONE',  ( -29.80992411920399832, 1383.842315663000136, 227.6115284750150067 ) ) ;
#45337=EDGE_CURVE ( 'NONE', #71158, #107758, #67374, .T. ) ;
#45346=CARTESIAN_POINT ( 'NONE',  ( -8.337699078158452792, 1386.911661598467845, 199.8791641365267822 ) ) ;
#45352=CARTESIAN_POINT ( 'NONE',  ( -12.49220237150879953, 1391.410446187260050, 209.7523967365880253 ) ) ;
#45362=CARTESIAN_POINT ( 'NONE',  ( -103.0445127499399831, 1385.228392731539770, 296.7348340301609824 ) ) ;
#45388=CARTESIAN_POINT ( 'NONE',  ( -104.4199114259999845, 1380.436187834239945, 300.6363748219590093 ) ) ;
#45420=CARTESIAN_POINT ( 'NONE',  ( -108.0465155092619938, 1384.898365638199948, 297.0924029035859348 ) ) ;
#45433=CARTESIAN_POINT ( 'NONE',  ( -105.3239982070000025, 1388.772974685380177, 299.3169349243589750 ) ) ;
#45436=CARTESIAN_POINT ( 'NONE',  ( -32.71421740720000315, 1379.624840865300030, 215.8883633175389889 ) ) ;
#45441=CARTESIAN_POINT ( 'NONE',  ( -59.67093331520844401, 1379.746016655268022, 264.7494437571154435 ) ) ;
#45449=CARTESIAN_POINT ( 'NONE',  ( -73.28822514871049520, 1385.013224671080025, 298.4902431103309937 ) ) ;
#45452=CARTESIAN_POINT ( 'NONE',  ( -8.060900218429999597, 1384.928187126620060, 199.5679324677990110 ) ) ;
#45477=CARTESIAN_POINT ( 'NONE',  ( -13.05809432774470125, 1379.371362203710078, 208.0847928999789929 ) ) ;
#45479=DIRECTION ( 'NONE',  ( 0.07268319384289673168, 0.1273111294819405659, 0.9891961532693243075 ) ) ;
#45500=CARTESIAN_POINT ( 'NONE',  ( -86.43903678570190152, 1384.625844868130116, 307.3438020039649814 ) ) ;
#45501=CARTESIAN_POINT ( 'NONE',  ( -48.09174099008450298, 1385.012596446669932, 222.4136726372699968 ) ) ;
#45508=CARTESIAN_POINT ( 'NONE',  ( -7.965887108789999616, 1384.923044073590063, 199.4891954346890088 ) ) ;
#45519=CARTESIAN_POINT ( 'NONE',  ( -12.23669308090000030, 1377.661331661229951, 207.7794332492889851 ) ) ;
#45533=CARTESIAN_POINT ( 'NONE',  ( -61.38583038131619674, 1379.728379092859768, 268.3198502261870431 ) ) ;
#45560=CARTESIAN_POINT ( 'NONE',  ( -7.544889814560000296, 1384.926148861729871, 219.0875907562389955 ) ) ;
#45562=CARTESIAN_POINT ( 'NONE',  ( -13.87256047439999840, 1379.747987721680147, 208.2173326269899860 ) ) ;
#45563=CARTESIAN_POINT ( 'NONE',  ( -67.76017963322829019, 1379.745894740751737, 277.9423129414287246 ) ) ;
#45574=CARTESIAN_POINT ( 'NONE',  ( -40.62152722268042027, 1379.659798262793174, 229.8373908348060866 ) ) ;
#45591=DIRECTION ( 'NONE',  ( 0.02939029866724141363, 0.9995213403039945321, 0.009659224666439003917 ) ) ;
#45592=CARTESIAN_POINT ( 'NONE',  ( -76.12965060780000215, 1386.571707002160110, 301.1838123932589610 ) ) ;
#45601=TOROIDAL_SURFACE ( 'NONE', #108140, 8.432239102140000497, 0.5000000000000000000 ) ;
#45605=CARTESIAN_POINT ( 'NONE',  ( -107.3840465399999999, 1380.275172143389909, 309.3291178842590057 ) ) ;
#45634=CARTESIAN_POINT ( 'NONE',  ( -33.44809598507389836, 1384.815296568380063, 232.0972948743769848 ) ) ;
#45658=CARTESIAN_POINT ( 'NONE',  ( -48.01530467240000633, 1376.719512341220025, 243.5457403057590113 ) ) ;
#45668=CARTESIAN_POINT ( 'NONE',  ( -8.984772871429999697, 1384.158943888290196, 218.6060625040090031 ) ) ;
#45690=CARTESIAN_POINT ( 'NONE',  ( -85.89269277900000077, 1377.100296256970068, 295.7491691192589656 ) ) ;
#45692=CARTESIAN_POINT ( 'NONE',  ( -106.5776706074079954, 1378.913060387289988, 301.7608484320570028 ) ) ;
#45703=CARTESIAN_POINT ( 'NONE',  ( -22.76979002380000239, 1383.850662563309925, 221.8906633995589743 ) ) ;
#45707=CARTESIAN_POINT ( 'NONE',  ( -67.88240010660000223, 1379.747289793479922, 278.3094642168589985 ) ) ;
#45716=CARTESIAN_POINT ( 'NONE',  ( -76.09441500830000393, 1384.885120960920176, 301.2261972959589684 ) ) ;
#45718=CARTESIAN_POINT ( 'NONE',  ( -29.06065178196929821, 1385.237911838130003, 227.0774918126679722 ) ) ;
#45721=CIRCLE ( 'NONE', #52907, 2.500000000000002220 ) ;
#45762=CARTESIAN_POINT ( 'NONE',  ( -83.03943510906880476, 1383.774858932900088, 305.4843309025330313 ) ) ;
#45765=CARTESIAN_POINT ( 'NONE',  ( -108.6615217476129942, 1383.758151187970270, 311.0749416052580045 ) ) ;
#45770=CARTESIAN_POINT ( 'NONE',  ( -62.73150586050000044, 1380.013960346400154, 278.0159453995589729 ) ) ;
#45776=CARTESIAN_POINT ( 'NONE',  ( -109.1650303699999967, 1384.945461312639964, 297.1327159909589568 ) ) ;
#45846=CARTESIAN_POINT ( 'NONE',  ( -33.87858360229999732, 1390.927706345010165, 218.8447143792689928 ) ) ;
#45847=CARTESIAN_POINT ( 'NONE',  ( -9.775687243024277606, 1386.869824447039491, 218.1688999378142455 ) ) ;
#45881=CARTESIAN_POINT ( 'NONE',  ( -21.58355234741789985, 1383.851891895520112, 221.4751650834180055 ) ) ;
#45884=CARTESIAN_POINT ( 'NONE',  ( 3.555115653736739510E-15, 1384.926148861439970, 209.1218459572589836 ) ) ;
#45889=CARTESIAN_POINT ( 'NONE',  ( -10.21949078822098933, 1389.864309992940434, 202.1513456453452022 ) ) ;
#45896=CARTESIAN_POINT ( 'NONE',  ( -8.873922351719999213, 1388.797700485470159, 217.8009811287190018 ) ) ;
#45904=CARTESIAN_POINT ( 'NONE',  ( -97.29371455280750070, 1385.213827748320227, 295.6673445477299538 ) ) ;
#45923=CARTESIAN_POINT ( 'NONE',  ( -8.296072169000000329, 1384.982551824029997, 218.7029005622489990 ) ) ;
#45924=DIRECTION ( 'NONE',  ( 1.835183309750130004E-16, 1.000000000000000000, 1.599799320660000123E-19 ) ) ;
#45927=CARTESIAN_POINT ( 'NONE',  ( -104.8261132509999953, 1380.717247260959994, 300.0167969450589567 ) ) ;
#45957=CARTESIAN_POINT ( 'NONE',  ( -108.9757583731840072, 1384.900984196950048, 297.1264776970670027 ) ) ;
#45980=ADVANCED_FACE ( 'NONE', ( #58043 ), #109098, .T. ) ;
#45983=CARTESIAN_POINT ( 'NONE',  ( -36.56818187795897757, 1379.727990715524356, 223.6839165922986297 ) ) ;
#45990=CARTESIAN_POINT ( 'NONE',  ( -63.63727237520100743, 1385.049170780109989, 286.7708433928359568 ) ) ;
#45991=DIRECTION ( 'NONE',  ( -1.000000000000000000, 0.000000000000000000, 0.000000000000000000 ) ) ;
#46020=CARTESIAN_POINT ( 'NONE',  ( -14.25010227119279982, 1379.583597535630133, 207.8942344209849864 ) ) ;
#46037=VECTOR ( 'NONE', #48616, 1000.000000000000000 ) ;
#46043=CARTESIAN_POINT ( 'NONE',  ( -43.65248483671320656, 1384.999294573369980, 216.7159599902390141 ) ) ;
#46044=CARTESIAN_POINT ( 'NONE',  ( -5.329878543928120216, 1374.946430637010053, 214.8576637461130190 ) ) ;
#46051=CARTESIAN_POINT ( 'NONE',  ( -8.156249721700000066, 1384.928229602200190, 199.6467685838189823 ) ) ;
#46058=CARTESIAN_POINT ( 'NONE',  ( -106.5125067552479976, 1391.913060387289988, 305.2240569073479719 ) ) ;
#46062=CARTESIAN_POINT ( 'NONE',  ( -12.00444414999999942, 1381.312822588570043, 202.5161199644090289 ) ) ;
#46076=CARTESIAN_POINT ( 'NONE',  ( -68.06332100059638890, 1379.746517069849915, 279.5343399889710554 ) ) ;
#46081=CARTESIAN_POINT ( 'NONE',  ( -105.6951163859999951, 1378.913064648980026, 305.0952293404590137 ) ) ;
#46088=CARTESIAN_POINT ( 'NONE',  ( -105.7995319784910038, 1378.913060387259975, 304.3206059282480282 ) ) ;
#46107=CARTESIAN_POINT ( 'NONE',  ( -8.581520137690000993, 1384.906045364150032, 218.6697283336690134 ) ) ;
#46109=CARTESIAN_POINT ( 'NONE',  ( -12.64088754379999990, 1379.240986521519744, 208.6656973887710080 ) ) ;
#46110=CARTESIAN_POINT ( 'NONE',  ( -66.32605177295688748, 1379.742644928997834, 275.0426332078492351 ) ) ;
#46146=CARTESIAN_POINT ( 'NONE',  ( -106.4193208100000021, 1384.931129459059775, 311.3263713972589812 ) ) ;
#46157=CARTESIAN_POINT ( 'NONE',  ( -106.3587827582539944, 1381.411344002460055, 309.3065060124769730 ) ) ;
#46167=( BOUNDED_CURVE ( )  B_SPLINE_CURVE ( 3, ( #80131, #53871, #96948, #88545 ),
 .UNSPECIFIED., .F., .T. ) 
 B_SPLINE_CURVE_WITH_KNOTS ( ( 4, 4 ),
 ( 1.037086443313566031, 2.104505668239319949 ),
 .UNSPECIFIED. ) 
 CURVE ( )  GEOMETRIC_REPRESENTATION_ITEM ( )  RATIONAL_B_SPLINE_CURVE ( ( 1.000000000000000000, 0.9072838702658839738, 0.9072838702658839738, 1.000000000000000000 ) ) 
 REPRESENTATION_ITEM ( '' )  );
#46183=CARTESIAN_POINT ( 'NONE',  ( -39.05830609401130005, 1384.791778035780226, 240.5085568879630102 ) ) ;
#46204=CARTESIAN_POINT ( 'NONE',  ( -82.97477735809999899, 1376.309726841469910, 300.0739800579590337 ) ) ;
#46214=CARTESIAN_POINT ( 'NONE',  ( -8.579897891159999901, 1384.651925423579996, 218.6623841843989737 ) ) ;
#46239=B_SPLINE_CURVE_WITH_KNOTS ( 'NONE', 3,
 ( #13869, #73819, #107394, #83301, #100103, #65980, #57022, #21713, #58117, #6043 ),
 .UNSPECIFIED., .F., .F.,
 ( 4, 3, 3, 4 ),
 ( 9.225465320329998775, 9.476690767968960927, 9.821219881794329254, 10.07010780362520030 ),
 .UNSPECIFIED. ) ;
#46242=CARTESIAN_POINT ( 'NONE',  ( -87.79856897099999458, 1379.577971547980042, 299.2711673883590038 ) ) ;
#46251=EDGE_CURVE ( 'NONE', #41641, #46650, #68556, .T. ) ;
#46253=ORIENTED_EDGE ( 'NONE', *, *, #50873, .T. ) ;
#46256=CARTESIAN_POINT ( 'NONE',  ( -5.958828918900000104, 1384.553407673830179, 218.5245230306490214 ) ) ;
#46262=CARTESIAN_POINT ( 'NONE',  ( -65.35196250319999933, 1379.741131604200064, 273.2162891523590247 ) ) ;
#46275=CARTESIAN_POINT ( 'NONE',  ( -23.86417894507290072, 1385.260624856700133, 222.9263582714870040 ) ) ;
#46279=MANIFOLD_SOLID_BREP ( 'Stock-MAS-682-1', #105696 ) ;
#46284=CARTESIAN_POINT ( 'NONE',  ( -7.965810688893188996, 1384.899971919800009, 199.4892299149449855 ) ) ;
#46301=CARTESIAN_POINT ( 'NONE',  ( -105.5067336309999888, 1391.271052109320181, 304.2081839319590131 ) ) ;
#46320=CARTESIAN_POINT ( 'NONE',  ( -76.80923957048339901, 1383.779367511659984, 301.3284849630780400 ) ) ;
#46322=CARTESIAN_POINT ( 'NONE',  ( -109.7747990662900008, 1384.235278760439996, 311.3356848936479651 ) ) ;
#46342=CARTESIAN_POINT ( 'NONE',  ( -68.77278092737650184, 1379.747928288920093, 280.3133413970129482 ) ) ;
#46346=VERTEX_POINT ( 'NONE', #66607 ) ;
#46370=VERTEX_POINT ( 'NONE', #17796 ) ;
#46401=ORIENTED_EDGE ( 'NONE', *, *, #24991, .F. ) ;
#46427=CARTESIAN_POINT ( 'NONE',  ( -110.0664121069999908, 1385.015438621219801, 296.9524368094589590 ) ) ;
#46438=CARTESIAN_POINT ( 'NONE',  ( -24.95503619787630356, 1383.848126923009886, 223.4623740270739916 ) ) ;
#46447=CARTESIAN_POINT ( 'NONE',  ( -46.07807520840000137, 1384.601971911739838, 219.0368719419589922 ) ) ;
#46453=CARTESIAN_POINT ( 'NONE',  ( -13.29669657483730205, 1389.765376659109961, 214.2158769609019942 ) ) ;
#46462=CARTESIAN_POINT ( 'NONE',  ( -95.64499328508460962, 1385.209349391769820, 295.1734178191939577 ) ) ;
#46464=CARTESIAN_POINT ( 'NONE',  ( -68.53407989799998745, 1379.748277114789971, 279.6522222015589705 ) ) ;
#46484=CARTESIAN_POINT ( 'NONE',  ( -8.580821470709999232, 1384.944142111179872, 218.6694750710489927 ) ) ;
#46485=B_SPLINE_SURFACE_WITH_KNOTS ( 'NONE', 5, 5, ( 
 ( #40558, #23194, #99342, #31600, #47313, #6412 ),
 ( #108316, #82574, #48433, #5304, #5866, #73634 ),
 ( #106653, #38890, #14799, #12607, #55186, #29944 ),
 ( #65231, #74732, #90957, #48985, #65779, #64136 ),
 ( #90395, #30501, #22617, #56821, #31049, #73072 ),
 ( #72524, #40007, #83118, #108866, #74185, #38345 ),
 ( #46787, #64690, #107213, #14244, #99896, #98257 ),
 ( #98808, #107765, #57393, #80917, #4215, #63592 ),
 ( #97709, #39462, #21526, #55738, #89860, #13129 ) ),
 .UNSPECIFIED., .F., .F., .F.,
 ( 6, 3, 6 ),
 ( 6, 6 ),
 ( 135.0843208316090056, 135.9934071210000184, 136.9024933901449970 ),
 ( 0.000000000000000000, 2.000049861391349992 ),
 .UNSPECIFIED. ) ;
#46505=ORIENTED_EDGE ( 'NONE', *, *, #110315, .F. ) ;
#46516=CARTESIAN_POINT ( 'NONE',  ( -109.0700388966839967, 1384.901248464930177, 297.1296046054879980 ) ) ;
#46537=CARTESIAN_POINT ( 'NONE',  ( -105.5460946514699998, 1391.484849259569955, 304.2071873224919614 ) ) ;
#46545=CARTESIAN_POINT ( 'NONE',  ( -88.01291097481920644, 1384.974171169579904, 308.0014400498420173 ) ) ;
#46558=DIRECTION ( 'NONE',  ( 0.8090169943747140824, -7.703825410061002683E-33, 0.5877852522927943246 ) ) ;
#46578=CARTESIAN_POINT ( 'NONE',  ( -7.749623004274919680, 1383.351629194430188, 218.8775256501539843 ) ) ;
#46592=CARTESIAN_POINT ( 'NONE',  ( -100.5338213842030086, 1384.599842449589914, 310.8803881067170209 ) ) ;
#46593=CARTESIAN_POINT ( 'NONE',  ( -42.80917332632159855, 1384.997012664380009, 215.7662912984700085 ) ) ;
#46600=CARTESIAN_POINT ( 'NONE',  ( -109.4843783879999961, 1384.890515631779863, 311.2841057952589949 ) ) ;
#46609=ADVANCED_FACE ( 'NONE', ( #90959 ), #37187, .T. ) ;
#46626=CARTESIAN_POINT ( 'NONE',  ( -68.18010506664271020, 1379.746744738860116, 279.6916017517709747 ) ) ;
#46631=CARTESIAN_POINT ( 'NONE',  ( -105.7844069010000112, 1378.913060387289988, 304.5472711634590155 ) ) ;
#46632=CARTESIAN_POINT ( 'NONE',  ( -109.8260976820000110, 1384.930814608760102, 311.3808200542590043 ) ) ;
#46650=VERTEX_POINT ( 'NONE', #25946 ) ;
#46657=CARTESIAN_POINT ( 'NONE',  ( -7.545178787140000232, 1384.911017756160163, 219.0875996242590134 ) ) ;
#46659=CARTESIAN_POINT ( 'NONE',  ( -62.44511414011146400, 1379.732285075670234, 266.8351904209325198 ) ) ;
#46663=CARTESIAN_POINT ( 'NONE',  ( -64.86421170961099847, 1384.704012963549985, 254.7553430863480060 ) ) ;
#46664=ORIENTED_EDGE ( 'NONE', *, *, #41222, .F. ) ;
#46666=VERTEX_POINT ( 'NONE', #63470 ) ;
#46691=CARTESIAN_POINT ( 'NONE',  ( -109.9987473089999952, 1389.430187130500144, 300.0861861933589694 ) ) ;
#46703=CARTESIAN_POINT ( 'NONE',  ( -104.5730503306040049, 1380.111946902090040, 306.5319961363489369 ) ) ;
#46729=CARTESIAN_POINT ( 'NONE',  ( -40.37520412227119948, 1384.785868538820068, 242.7915335778529879 ) ) ;
#46733=ADVANCED_FACE ( 'NONE', ( #87548 ), #24133, .F. ) ;
#46755=CARTESIAN_POINT ( 'NONE',  ( -60.58607047561810077, 1378.469422833939916, 271.2016459589009969 ) ) ;
#46759=CARTESIAN_POINT ( 'NONE',  ( -21.77664080601369889, 1379.664485263579991, 213.4127619154490105 ) ) ;
#46766=CARTESIAN_POINT ( 'NONE',  ( -8.591590428069999064, 1384.539102583910108, 218.6519172601589958 ) ) ;
#46787=CARTESIAN_POINT ( 'NONE',  ( -12.31367108914779962, 1378.373004075840072, 209.7324437289769890 ) ) ;
#46788=( GEOMETRIC_REPRESENTATION_CONTEXT ( 3 ) GLOBAL_UNCERTAINTY_ASSIGNED_CONTEXT ( ( #9894 ) ) GLOBAL_UNIT_ASSIGNED_CONTEXT ( ( #22054, #6938, #7494 ) ) REPRESENTATION_CONTEXT ( 'NONE', 'WORKASPACE' ) );
#46791=CARTESIAN_POINT ( 'NONE',  ( -46.19755678469999793, 1379.154583033749986, 231.0255711761590192 ) ) ;
#46802=CARTESIAN_POINT ( 'NONE',  ( -8.753528060440000758, 1383.864184473070054, 218.4105340633189769 ) ) ;
#46807=CARTESIAN_POINT ( 'NONE',  ( -68.17091063920000238, 1379.746761204979975, 278.7818561045589831 ) ) ;
#46816=CARTESIAN_POINT ( 'NONE',  ( -73.55519582189999994, 1385.011955127469946, 298.9534985252589649 ) ) ;
#46818=CARTESIAN_POINT ( 'NONE',  ( -27.83627237203649685, 1385.243440311610129, 225.9367174611259941 ) ) ;
#46822=CARTESIAN_POINT ( 'NONE',  ( -106.4049156021218465, 1391.248059910561551, 307.7491788416908776 ) ) ;
#46846=CARTESIAN_POINT ( 'NONE',  ( -106.7279299509999930, 1391.913060387289988, 302.2165404876590173 ) ) ;
#46863=CARTESIAN_POINT ( 'NONE',  ( -109.4664803445590024, 1384.534987613060139, 311.2654761184969630 ) ) ;
#46918=AXIS2_PLACEMENT_3D ( 'NONE', #59892, #58778, #69406 ) ;
#46925=CARTESIAN_POINT ( 'NONE',  ( -20.72234375626489822, 1384.535007408160027, 201.8751713657979963 ) ) ;
#46976=DIRECTION ( 'NONE',  ( -1.836970198721029688E-16, -1.000000000000000000, 0.000000000000000000 ) ) ;
#46982=CARTESIAN_POINT ( 'NONE',  ( -43.29541590384620520, 1383.822952073729994, 247.8268964491909685 ) ) ;
#46990=CARTESIAN_POINT ( 'NONE',  ( -26.04564454490000003, 1383.846902489159902, 224.1106665064590118 ) ) ;
#46997=CARTESIAN_POINT ( 'NONE',  ( -8.317554072875960713, 1387.933845735730074, 218.3619299428229965 ) ) ;
#47005=CARTESIAN_POINT ( 'NONE',  ( -95.05608304844369627, 1385.207712179709915, 294.9719338976229892 ) ) ;
#47019=CARTESIAN_POINT ( 'NONE',  ( -109.9058460539999942, 1384.928481735109926, 311.4185263572589975 ) ) ;
#47028=CARTESIAN_POINT ( 'NONE',  ( -7.543627442569999175, 1385.104043808209781, 219.0827038849589883 ) ) ;
#47078=CARTESIAN_POINT ( 'NONE',  ( -106.3976924294359918, 1390.939209247700092, 307.7528211820909974 ) ) ;
#47083=ORIENTED_EDGE ( 'NONE', *, *, #84419, .F. ) ;
#47086=CARTESIAN_POINT ( 'NONE',  ( -79.14188242860410583, 1384.996239183999933, 303.2876060637049704 ) ) ;
#47087=CARTESIAN_POINT ( 'NONE',  ( -9.699806184529998987, 1388.369311790329903, 201.2298857673789882 ) ) ;
#47112=DIRECTION ( 'NONE',  ( -1.000000000000000000, 0.000000000000000000, 0.000000000000000000 ) ) ;
#47129=CARTESIAN_POINT ( 'NONE',  ( -85.23413153088101524, 1384.628137661299888, 306.7983909476229769 ) ) ;
#47131=CARTESIAN_POINT ( 'NONE',  ( -32.91460356916239505, 1384.974432874500053, 207.2804400437590004 ) ) ;
#47150=CARTESIAN_POINT ( 'NONE',  ( -14.05078142410000019, 1379.708754511839743, 206.9026084073089748 ) ) ;
#47161=CARTESIAN_POINT ( 'NONE',  ( -68.39393351552520528, 1379.747380541330131, 279.9548358144079998 ) ) ;
#47172=CARTESIAN_POINT ( 'NONE',  ( -106.5595845979900105, 1378.913060387289988, 306.5187700427659934 ) ) ;
#47179=CARTESIAN_POINT ( 'NONE',  ( -10.25368860849440011, 1391.913060387289988, 204.2726074216130030 ) ) ;
#47186=CARTESIAN_POINT ( 'NONE',  ( -14.11750138697139789, 1379.894919723800058, 211.2943169131719969 ) ) ;
#47191=CARTESIAN_POINT ( 'NONE',  ( -68.61568296326619532, 1379.747656804948974, 279.7483219046964678 ) ) ;
#47195=CARTESIAN_POINT ( 'NONE',  ( -55.20091899711550099, 1384.645211897679928, 234.2512433511650158 ) ) ;
#47251=CIRCLE ( 'NONE', #108055, 11.26398391340000060 ) ;
#47258=CARTESIAN_POINT ( 'NONE',  ( -39.59684760391189684, 1384.789378137079893, 241.4292011553590100 ) ) ;
#47282=CARTESIAN_POINT ( 'NONE',  ( -52.72375982305769782, 1377.543534630760178, 254.3719140001319943 ) ) ;
#47293=CARTESIAN_POINT ( 'NONE',  ( -8.022767810259999521, 1384.891328718040086, 218.7875262017990110 ) ) ;
#47313=CARTESIAN_POINT ( 'NONE',  ( -13.88306073332670110, 1379.761802596040070, 208.2296390988570067 ) ) ;
#47317=CARTESIAN_POINT ( 'NONE',  ( -58.56722971349999796, 1374.895658628189949, 258.8926058799589782 ) ) ;
#47325=EDGE_LOOP ( 'NONE', ( #14659, #34118, #51111, #60767 ) ) ;
#47329=CARTESIAN_POINT ( 'NONE',  ( -38.49145949329999894, 1384.794605546870116, 239.3122526757589981 ) ) ;
#47334=CARTESIAN_POINT ( 'NONE',  ( -65.09292129899999679, 1379.738243665130085, 272.5656652546590522 ) ) ;
#47346=CARTESIAN_POINT ( 'NONE',  ( -24.11259409631230000, 1385.259584648939835, 223.0827457712539967 ) ) ;
#47356=EDGE_CURVE ( 'NONE', #13762, #49801, #21153, .T. ) ;
#47364=ORIENTED_EDGE ( 'NONE', *, *, #89465, .F. ) ;
#47369=CARTESIAN_POINT ( 'NONE',  ( -119.4674887953348872, 1384.913060387289988, 299.8135573092559412 ) ) ;
#47376=CARTESIAN_POINT ( 'NONE',  ( -104.3158487040000040, 1389.466353268959892, 300.6607691406589993 ) ) ;
#47378=CARTESIAN_POINT ( 'NONE',  ( -105.9112875430000145, 1391.839465932129997, 303.4711480509590160 ) ) ;
#47403=EDGE_LOOP ( 'NONE', ( #53557, #104542, #54089, #48427, #16334 ) ) ;
#47404=CARTESIAN_POINT ( 'NONE',  ( -113.4000000000000057, 1382.004344128540197, 297.9600760927590386 ) ) ;
#47410=CARTESIAN_POINT ( 'NONE',  ( -8.393274306154939524, 1382.788095255750022, 199.9340640290776321 ) ) ;
#47452=VERTEX_POINT ( 'NONE', #34101 ) ;
#47459=CARTESIAN_POINT ( 'NONE',  ( -26.52518363774159837, 1384.548060173010072, 203.9081812816960166 ) ) ;
#47473=CARTESIAN_POINT ( 'NONE',  ( -68.77805555110001023, 1379.747954593040049, 280.2446631412590250 ) ) ;
#47488=CARTESIAN_POINT ( 'NONE',  ( -9.094202543475169875, 1384.745265098430082, 199.9473045631640105 ) ) ;
#47523=CARTESIAN_POINT ( 'NONE',  ( -50.96332219156189325, 1383.810333793590189, 263.3241036801269956 ) ) ;
#47532=CARTESIAN_POINT ( 'NONE',  ( -13.47003478659999942, 1382.321222797600058, 218.2872753327090152 ) ) ;
#47539=B_SPLINE_CURVE_WITH_KNOTS ( 'NONE', 3,
 ( #102053, #15821, #75773, #24778, #41619, #16925, #84156, #73158, #33748, #84703, #38981, #30030, #49478, #23697, #8003, #109384, #93643, #50025, #64784, #58425, #93108, #41055, #75234, #51127, #58977, #100948, #15286, #50576, #33203, #7456, #109923, #6900, #32661, #16378, #66838, #25336, #42168, #64224, #67393, #98347, #21620, #101491, #55825, #83602, #76321, #24243, #110471, #72612, #47410, #85251, #57882, #8551, #106743, #98894, #89945, #13220 ),
 .UNSPECIFIED., .F., .F.,
 ( 4, 2, 2, 2, 2, 2, 2, 2, 2, 1, 1, 2, 2, 2, 1, 1, 1, 2, 2, 2, 2, 1, 1, 2, 2, 2, 2, 1, 1, 1, 2, 2, 4 ),
 ( 0.000000000000000000, 0.1250000000005362932, 0.1875000000008112955, 0.2187500000009487966, 0.2500000000010862977, 0.3125000000013673507, 0.3437500000014971357, 0.3750000000016269763, 0.4375000000018683943, 0.4687500000019733659, 0.4843750000020397573, 0.4921875000020562441, 0.5000000000020726754, 0.5625000000021440627, 0.5937500000021798119, 0.6093750000022118973, 0.6171875000022302160, 0.6210937500022218893, 0.6250000000022134516, 0.6875000000020528024, 0.7187500000019703128, 0.7343750000019292345, 0.7421875000019292345, 0.7460937500019085844, 0.7500000000018879343, 0.8125000000017519319, 0.8437500000016620039, 0.8593750000016184831, 0.8671875000016213697, 0.8710937500016240342, 0.8730468750016000534, 0.8750000000015760726, 1.000000000000000000 ),
 .UNSPECIFIED. ) ;
#47540=CARTESIAN_POINT ( 'NONE',  ( -11.49982667903889855, 1391.068238042669918, 213.8785252920860103 ) ) ;
#47542=CARTESIAN_POINT ( 'NONE',  ( -8.751716459555160199, 1384.978504587089901, 220.6816886054729991 ) ) ;
#47560=CARTESIAN_POINT ( 'NONE',  ( -109.3311711570000000, 1386.522315934440030, 311.1006615362589969 ) ) ;
#47569=CARTESIAN_POINT ( 'NONE',  ( -8.021685169730000453, 1385.080864991280123, 218.7833935487189763 ) ) ;
#47576=VECTOR ( 'NONE', #96596, 999.9999999999998863 ) ;
#47590=FACE_OUTER_BOUND ( 'NONE', #54910, .T. ) ;
#47607=ORIENTED_EDGE ( 'NONE', *, *, #85697, .T. ) ;
#47617=CARTESIAN_POINT ( 'NONE',  ( -108.3228733452354504, 1380.963783207329016, 298.1737543167551507 ) ) ;
#47621=CARTESIAN_POINT ( 'NONE',  ( -105.4624875116129914, 1391.255303400100047, 304.2078100440970161 ) ) ;
#47628=CARTESIAN_POINT ( 'NONE',  ( -93.64869092343039370, 1384.961098842790079, 309.7453634167209771 ) ) ;
#47630=CARTESIAN_POINT ( 'NONE',  ( -9.963621752110000784, 1388.075463991820016, 201.3019539889990028 ) ) ;
#47642=CARTESIAN_POINT ( 'NONE',  ( -110.0482597500069915, 1385.373319905469771, 296.9711118272649628 ) ) ;
#47675=CARTESIAN_POINT ( 'NONE',  ( -13.69967938769999982, 1380.327631092480033, 209.8719513141080029 ) ) ;
#47676=CARTESIAN_POINT ( 'NONE',  ( -103.9238620277660061, 1384.593426725770087, 311.1343658853500642 ) ) ;
#47677=CARTESIAN_POINT ( 'NONE',  ( -56.36773401075790701, 1385.044407682810061, 236.4819119073529805 ) ) ;
#47689=CARTESIAN_POINT ( 'NONE',  ( -109.1343026320000007, 1384.783638055820120, 311.2626717992590102 ) ) ;
#47697=CARTESIAN_POINT ( 'NONE',  ( -13.83438311809999810, 1379.888128081619925, 206.0089139935990090 ) ) ;
#47705=ORIENTED_EDGE ( 'NONE', *, *, #87675, .F. ) ;
#47708=CARTESIAN_POINT ( 'NONE',  ( -67.09039466822581232, 1379.744314274860017, 278.2050095193470156 ) ) ;
#47728=EDGE_LOOP ( 'NONE', ( #374, #25362, #3016 ) ) ;
#47734=CIRCLE ( 'NONE', #54861, 2.000051271460090430 ) ;
#47736=CARTESIAN_POINT ( 'NONE',  ( -63.85514023855817811, 1379.736301226116211, 269.8882248764738847 ) ) ;
#47740=CARTESIAN_POINT ( 'NONE',  ( -73.46068911739270391, 1384.758501831970079, 272.7067926322189919 ) ) ;
#47807=CARTESIAN_POINT ( 'NONE',  ( -24.34705444099909855, 1384.848287400760228, 223.2598029039740197 ) ) ;
#47809=AXIS2_PLACEMENT_3D ( 'NONE', #42436, #92286, #15009 ) ;
#47817=EDGE_LOOP ( 'NONE', ( #34766, #6119, #110183, #10953, #32440, #75869, #108722 ) ) ;
#47832=CARTESIAN_POINT ( 'NONE',  ( -75.41334994439999662, 1376.365900248229991, 294.0916975056589990 ) ) ;
#47834=CARTESIAN_POINT ( 'NONE',  ( -14.07256126937990004, 1379.709109777840013, 211.5290051616560163 ) ) ;
#47843=CARTESIAN_POINT ( 'NONE',  ( -104.1991585039999961, 1389.999238680429926, 304.1793527667589956 ) ) ;
#47867=CARTESIAN_POINT ( 'NONE',  ( -46.72344042710000878, 1377.583786706710043, 230.7048910953589882 ) ) ;
#47880=CARTESIAN_POINT ( 'NONE',  ( -89.71137825399999599, 1383.770488589559818, 308.5740051020589476 ) ) ;
#47884=CARTESIAN_POINT ( 'NONE',  ( -47.55875411400000274, 1379.740588162619815, 235.3895649973590025 ) ) ;
#47889=STYLED_ITEM ( 'NONE', ( #59438 ), #46279 ) ;
#47894=CARTESIAN_POINT ( 'NONE',  ( -106.4193208199999958, 1384.816937872099970, 311.3271286962590239 ) ) ;
#47895=CARTESIAN_POINT ( 'NONE',  ( -31.92467753469999892, 1384.972130813700005, 206.3032401593790155 ) ) ;
#47897=CARTESIAN_POINT ( 'NONE',  ( -54.15112835251079559, 1385.097464586390061, 270.1434570728429776 ) ) ;
#47902=CARTESIAN_POINT ( 'NONE',  ( -107.0144515918482284, 1391.913060387290216, 307.4418155938021187 ) ) ;
#47923=CARTESIAN_POINT ( 'NONE',  ( -106.1649378089999942, 1391.047127029819876, 300.9392596058589788 ) ) ;
#47925=CARTESIAN_POINT ( 'NONE',  ( -105.9134739529999933, 1391.838461175369957, 304.2044424958590412 ) ) ;
#47941=CARTESIAN_POINT ( 'NONE',  ( -7.965810688893188996, 1384.899971919800009, 199.4892299149449855 ) ) ;
#47947=CARTESIAN_POINT ( 'NONE',  ( -106.7189926970000187, 1380.782700635500078, 299.4006339732590050 ) ) ;
#47981=CARTESIAN_POINT ( 'NONE',  ( -9.092273600540000444, 1384.801544621870107, 199.9443845869589893 ) ) ;
#48020=CARTESIAN_POINT ( 'NONE',  ( -68.75214133429999208, 1379.747884264789946, 280.1338633208590068 ) ) ;
#48036=CARTESIAN_POINT ( 'NONE',  ( -14.06834915342731485, 1379.597580802498896, 211.7528822239692659 ) ) ;
#48041=CARTESIAN_POINT ( 'NONE',  ( -113.4000000000000057, 1391.913060387289988, 304.2218459572590064 ) ) ;
#48073=CARTESIAN_POINT ( 'NONE',  ( -36.57638826848899782, 1383.833252621880092, 236.1977204853059789 ) ) ;
#48074=( BOUNDED_CURVE ( )  B_SPLINE_CURVE ( 3, ( #62049, #77720, #26755, #18888 ),
 .UNSPECIFIED., .F., .F. ) 
 B_SPLINE_CURVE_WITH_KNOTS ( ( 4, 4 ),
 ( 0.1582411938933160067, 0.2197467457803065072 ),
 .UNSPECIFIED. ) 
 CURVE ( )  GEOMETRIC_REPRESENTATION_ITEM ( )  RATIONAL_B_SPLINE_CURVE ( ( 1.000000000000000000, 0.9996847804345658783, 0.9996847804345658783, 1.000000000000000000 ) ) 
 REPRESENTATION_ITEM ( '' )  );
#48083=CARTESIAN_POINT ( 'NONE',  ( -28.08746868569999933, 1382.324033938389903, 225.1301489039589967 ) ) ;
#48089=CARTESIAN_POINT ( 'NONE',  ( -10.43842217732019861, 1388.008184915300035, 217.2398969709649919 ) ) ;
#48091=DIRECTION ( 'NONE',  ( 1.000000000000000000, 0.000000000000000000, 0.000000000000000000 ) ) ;
#48093=CARTESIAN_POINT ( 'NONE',  ( -106.3207909569999998, 1379.688851738430003, 300.3888801278590108 ) ) ;
#48114=CARTESIAN_POINT ( 'NONE',  ( -108.6094801609999934, 1386.676297506519859, 310.8587284262589492 ) ) ;
#48143=CARTESIAN_POINT ( 'NONE',  ( 2.140036995326180090E-16, 1390.913060387289988, 209.1218459572589836 ) ) ;
#48149=CARTESIAN_POINT ( 'NONE',  ( -23.00023858420000167, 1384.678484070659806, 202.3918768682790130 ) ) ;
#48175=CARTESIAN_POINT ( 'NONE',  ( -109.2435801578418619, 1382.302282213249782, 297.4663600009405968 ) ) ;
#48187=CARTESIAN_POINT ( 'NONE',  ( -80.39083381333070122, 1384.992927882670074, 304.1219082020649580 ) ) ;
#48189=CARTESIAN_POINT ( 'NONE',  ( -9.123030677640000974, 1385.451960981700040, 199.9749920654289781 ) ) ;
#48199=B_SPLINE_SURFACE_WITH_KNOTS ( 'NONE', 5, 5, ( 
 ( #103979, #79346, #62014, #46863, #36232, #27275 ),
 ( #12683, #61458, #53049, #63134, #78790, #95584 ),
 ( #106193, #46322, #71539, #37342, #2659, #2106 ),
 ( #104537, #36785, #80993, #44648, #88844, #70978 ),
 ( #80450, #3763, #105094, #88293, #105660, #37897 ),
 ( #63670, #96134, #29475, #72079, #28945, #97235 ),
 ( #70419, #79900, #27834, #28384, #4299, #19413 ),
 ( #62585, #53614, #97781, #21058, #96702, #11587 ),
 ( #55263, #87756, #89394, #20508, #54167, #45765 ) ),
 .UNSPECIFIED., .F., .F., .F.,
 ( 6, 3, 6 ),
 ( 6, 6 ),
 ( 4.283793212480669688, 5.549035871040000067, 6.814275327763410495 ),
 ( -0.0004314831893375249629, 2.000000000000000000 ),
 .UNSPECIFIED. ) ;
#48202=CARTESIAN_POINT ( 'NONE',  ( -109.4000724753198170, 1387.258595658028071, 297.3646005980954783 ) ) ;
#48228=CARTESIAN_POINT ( 'NONE',  ( -103.5788295108265231, 1379.883385647208115, 304.1094550558439664 ) ) ;
#48236=CARTESIAN_POINT ( 'NONE',  ( -64.28120925927808571, 1385.082940760139991, 253.4381211720830436 ) ) ;
#48243=CARTESIAN_POINT ( 'NONE',  ( -109.8253977639999874, 1384.918085983840001, 311.3807728672589406 ) ) ;
#48246=CARTESIAN_POINT ( 'NONE',  ( -109.8216762179999932, 1384.604528214259744, 311.3701024542589835 ) ) ;
#48261=CARTESIAN_POINT ( 'NONE',  ( -5.439576477476709471, 1374.913517049739994, 203.3383520319619890 ) ) ;
#48268=CARTESIAN_POINT ( 'NONE',  ( -68.29419003885790573, 1379.746815713430124, 279.8507461170009947 ) ) ;
#48272=CARTESIAN_POINT ( 'NONE',  ( -8.214667976841889541, 1382.175473383424332, 218.4482751763555370 ) ) ;
#48273=VERTEX_POINT ( 'NONE', #10727 ) ;
#48279=CARTESIAN_POINT ( 'NONE',  ( -107.0358864074350009, 1378.913060387289988, 307.2354898942079444 ) ) ;
#48287=CIRCLE ( 'NONE', #62627, 7.999657266239995401 ) ;
#48304=CARTESIAN_POINT ( 'NONE',  ( -81.95025445411960163, 1384.803819859970190, 285.5341702218789806 ) ) ;
#48314=CARTESIAN_POINT ( 'NONE',  ( -109.0682564771375098, 1384.413434012951711, 311.2315974213690311 ) ) ;
#48362=B_SPLINE_CURVE_WITH_KNOTS ( 'NONE', 5,
 ( #1799, #35936, #70121, #63903, #39783, #99112 ),
 .UNSPECIFIED., .F., .F.,
 ( 6, 6 ),
 ( 0.4226397637529890061, 0.4682762820520000036 ),
 .UNSPECIFIED. ) ;
#48371=CARTESIAN_POINT ( 'NONE',  ( -42.31304661141189882, 1384.776936385030012, 246.3345890605239958 ) ) ;
#48372=CARTESIAN_POINT ( 'NONE',  ( -106.5026996092109925, 1391.913060387289988, 303.1716863602470085 ) ) ;
#48388=CARTESIAN_POINT ( 'NONE',  ( -12.16190383725469992, 1378.259213814440045, 211.1523455089300114 ) ) ;
#48398=CARTESIAN_POINT ( 'NONE',  ( -18.76552339101630196, 1380.296266887499996, 210.4014709065379805 ) ) ;
#48400=CARTESIAN_POINT ( 'NONE',  ( -21.79878488383639734, 1379.715451835960039, 213.3535203440429768 ) ) ;
#48412=CIRCLE ( 'NONE', #105633, 2.000015520878148934 ) ;
#48427=ORIENTED_EDGE ( 'NONE', *, *, #74340, .F. ) ;
#48430=CARTESIAN_POINT ( 'NONE',  ( -108.4919463386471818, 1388.455631213034849, 310.4216145322829448 ) ) ;
#48433=CARTESIAN_POINT ( 'NONE',  ( -12.63851992163809967, 1379.319802075649932, 208.7650603020850042 ) ) ;
#48437=CARTESIAN_POINT ( 'NONE',  ( -41.40570855549999862, 1380.117442312619914, 227.6002677670589947 ) ) ;
#48452=CARTESIAN_POINT ( 'NONE',  ( -43.08084643290000315, 1384.773678278489797, 247.5054735941590138 ) ) ;
#48465=CARTESIAN_POINT ( 'NONE',  ( -39.09877692349999734, 1389.679302472760128, 233.5893560917589866 ) ) ;
#48467=CARTESIAN_POINT ( 'NONE',  ( -42.32708834505060480, 1385.168503165180255, 246.3381990889729991 ) ) ;
#48479=ORIENTED_EDGE ( 'NONE', *, *, #106358, .T. ) ;
#48493=CARTESIAN_POINT ( 'NONE',  ( -107.7927744079999997, 1388.954798810650118, 298.5901260703590196 ) ) ;
#48495=CARTESIAN_POINT ( 'NONE',  ( -105.8185464679999939, 1391.163751785419890, 301.8501960914589972 ) ) ;
#48498=CARTESIAN_POINT ( 'NONE',  ( -103.5801441629999857, 1379.883084196419986, 303.9981228830590112 ) ) ;
#48514=CARTESIAN_POINT ( 'NONE',  ( -103.7373262539999956, 1383.424473230740205, 296.9348076431590471 ) ) ;
#48582=AXIS2_PLACEMENT_3D ( 'NONE', #95127, #18389, #54255 ) ;
#48616=DIRECTION ( 'NONE',  ( 0.000000000000000000, 0.000000000000000000, -1.000000000000000000 ) ) ;
#48620=CARTESIAN_POINT ( 'NONE',  ( -105.0711645279999971, 1379.235653477059941, 303.4121855584589866 ) ) ;
#48638=CARTESIAN_POINT ( 'NONE',  ( -44.80631001358410259, 1383.820492996369921, 250.7713395079869656 ) ) ;
#48647=TOROIDAL_SURFACE ( 'NONE', #379, 8.013264357029999729, 0.5000000000000000000 ) ;
#48648=CARTESIAN_POINT ( 'NONE',  ( -19.95507914119999526, 1380.898749975469855, 218.5439484314190111 ) ) ;
#48658=CARTESIAN_POINT ( 'NONE',  ( -105.4616672789999967, 1378.899769895130021, 302.9954926620590072 ) ) ;
#48677=CARTESIAN_POINT ( 'NONE',  ( -109.1897705290000005, 1387.438473340760083, 310.9485453702590121 ) ) ;
#48686=CARTESIAN_POINT ( 'NONE',  ( -14.32246179293609778, 1379.592251131270132, 207.9805893340429748 ) ) ;
#48699=CARTESIAN_POINT ( 'NONE',  ( -107.3712700886850087, 1378.913060387339783, 300.6990228053219312 ) ) ;
#48700=DIRECTION ( 'NONE',  ( 0.9991156138703696232, -3.961952592064073292E-33, -0.04204747460233797945 ) ) ;
#48705=CARTESIAN_POINT ( 'NONE',  ( -64.53155199309999546, 1384.701788983860297, 254.0354793386590018 ) ) ;
#48744=CARTESIAN_POINT ( 'NONE',  ( -100.5300167084300114, 1384.945107703380017, 310.8927782480189990 ) ) ;
#48746=CARTESIAN_POINT ( 'NONE',  ( -8.973420627790000381, 1387.914350804760033, 200.5228873143890098 ) ) ;
#48777=DIRECTION ( 'NONE',  ( -0.9998780014336184907, 0.000000000000000000, 0.01561993114942984012 ) ) ;
#48786=CARTESIAN_POINT ( 'NONE',  ( -105.1938507991023783, 1381.037482386520196, 308.6129917943122791 ) ) ;
#48793=CARTESIAN_POINT ( 'NONE',  ( -12.93896584940000061, 1379.674138171649929, 211.0424427186889886 ) ) ;
#48795=CARTESIAN_POINT ( 'NONE',  ( -57.23345819662650058, 1385.048296059559789, 238.2082995797720173 ) ) ;
#48806=CARTESIAN_POINT ( 'NONE',  ( -109.3108433829999910, 1384.813040219950153, 311.2635926062589533 ) ) ;
#48814=CARTESIAN_POINT ( 'NONE',  ( -9.959589622450000235, 1382.751681251990021, 218.0704319110489848 ) ) ;
#48821=VERTEX_POINT ( 'NONE', #109730 ) ;
#48822=CARTESIAN_POINT ( 'NONE',  ( -109.1310292459999829, 1384.726238503300010, 311.2600142160089831 ) ) ;
#48824=CARTESIAN_POINT ( 'NONE',  ( -68.54407940739999106, 1379.747756885790068, 280.1275194418589649 ) ) ;
#48828=CARTESIAN_POINT ( 'NONE',  ( -9.188021672635125370, 1380.611693761624338, 217.4304852955527281 ) ) ;
#48837=B_SPLINE_CURVE_WITH_KNOTS ( 'NONE', 3,
 ( #99597, #57646, #49235, #5001, #101239, #56527, #83358, #32420, #24539, #48686, #66599, #65487, #5565, #22880, #6103, #100703 ),
 .UNSPECIFIED., .F., .F.,
 ( 4, 3, 3, 3, 3, 4 ),
 ( -1.546267078793030159, -1.336910296889620042, -1.002126681165210087, -0.6673763298341559569, -0.3329907222668331279, 0.000000000000000000 ),
 .UNSPECIFIED. ) ;
#48838=CARTESIAN_POINT ( 'NONE',  ( -107.9127952440289988, 1378.913060387289988, 308.3607811453639442 ) ) ;
#48861=CARTESIAN_POINT ( 'NONE',  ( -83.83778724580230346, 1384.812601443120002, 287.5995587299269687 ) ) ;
#48872=CARTESIAN_POINT ( 'NONE',  ( -10.22326110114815556, 1375.913060387289988, 213.8507217284212345 ) ) ;
#48913=CARTESIAN_POINT ( 'NONE',  ( -8.107194294532323653, 1387.417305483015980, 218.5499404544749211 ) ) ;
#48930=CARTESIAN_POINT ( 'NONE',  ( -55.04194086205259850, 1384.716586501660004, 271.8950046832100043 ) ) ;
#48931=CARTESIAN_POINT ( 'NONE',  ( -106.6599773620300056, 1391.913060387289988, 302.5710412761980024 ) ) ;
#48933=CARTESIAN_POINT ( 'NONE',  ( -106.7897227899999990, 1379.694571751269905, 299.8550812676590454 ) ) ;
#48944=CARTESIAN_POINT ( 'NONE',  ( -13.44545695640730010, 1379.581665062349884, 211.7224066084869776 ) ) ;
#48954=CARTESIAN_POINT ( 'NONE',  ( -3.771520277320000503, 1377.099040908540019, 211.4935541149690152 ) ) ;
#48956=CARTESIAN_POINT ( 'NONE',  ( -43.47249194799999827, 1379.734446420929999, 233.2730947026589661 ) ) ;
#48983=CARTESIAN_POINT ( 'NONE',  ( -107.4005018563592273, 1389.804008732182183, 309.3201767723587068 ) ) ;
#48985=CARTESIAN_POINT ( 'NONE',  ( -13.17437943089760033, 1379.876859876259914, 208.7616546775940094 ) ) ;
#48989=CARTESIAN_POINT ( 'NONE',  ( -59.84652512769999788, 1375.824862300619998, 258.3077303912590423 ) ) ;
#49002=CARTESIAN_POINT ( 'NONE',  ( -81.27653993580000247, 1383.775959360260003, 304.8043613862590746 ) ) ;
#49014=CARTESIAN_POINT ( 'NONE',  ( -77.04812550189998888, 1389.484839475800072, 284.7597100018589913 ) ) ;
#49016=CARTESIAN_POINT ( 'NONE',  ( -41.13573424065770467, 1385.175475063010026, 244.1333310952810223 ) ) ;
#49044=CARTESIAN_POINT ( 'NONE',  ( -104.4016991209999929, 1389.881826709800180, 301.9201043558590527 ) ) ;
#49060=CARTESIAN_POINT ( 'NONE',  ( -106.4346700481279981, 1383.759796027640050, 311.0497744043260013 ) ) ;
#49086=VERTEX_POINT ( 'NONE', #82742 ) ;
#49107=CARTESIAN_POINT ( 'NONE',  ( -108.3070719650000058, 1383.318204079829911, 297.4475841893589632 ) ) ;
#49114=EDGE_LOOP ( 'NONE', ( #27409, #16634, #55143, #47607 ) ) ;
#49119=CARTESIAN_POINT ( 'NONE',  ( -18.95489208017639982, 1384.531068566690010, 201.4205921255219778 ) ) ;
#49133=CARTESIAN_POINT ( 'NONE',  ( -68.77190080519999071, 1379.747925807450201, 280.3125203366930123 ) ) ;
#49186=CARTESIAN_POINT ( 'NONE',  ( -52.84872043374259931, 1383.807289815149943, 267.1640630856880421 ) ) ;
#49196=CARTESIAN_POINT ( 'NONE',  ( -68.61981551019999870, 1383.223412842329935, 263.4739815647590149 ) ) ;
#49200=CARTESIAN_POINT ( 'NONE',  ( -8.105405351571780770, 1386.750627257020142, 218.6043960686319849 ) ) ;
#49205=CARTESIAN_POINT ( 'NONE',  ( -105.0671882769999996, 1380.670236109440111, 300.1379999032590149 ) ) ;
#49223=CARTESIAN_POINT ( 'NONE',  ( -109.2341786859999928, 1385.225129184130083, 311.2612912872589845 ) ) ;
#49235=CARTESIAN_POINT ( 'NONE',  ( -14.45214300844910227, 1379.635521336690090, 208.1492130568690015 ) ) ;
#49255=CARTESIAN_POINT ( 'NONE',  ( -79.49669931849999216, 1385.035068832460183, 282.9465538581589499 ) ) ;
#49283=CARTESIAN_POINT ( 'NONE',  ( -13.73096378239999993, 1379.766844552289967, 213.0184681208289987 ) ) ;
#49290=CARTESIAN_POINT ( 'NONE',  ( -8.598235764689999172, 1385.896259083729774, 199.9307053391690090 ) ) ;
#49321=CARTESIAN_POINT ( 'NONE',  ( -109.7179933470000037, 1384.899991331759793, 297.0862032941589632 ) ) ;
#49325=CARTESIAN_POINT ( 'NONE',  ( -105.2493395317690954, 1381.076302546985289, 308.6808743251384044 ) ) ;
#49331=CARTESIAN_POINT ( 'NONE',  ( -12.48493277280000058, 1379.220736522750030, 210.8106142036189965 ) ) ;
#49333=CARTESIAN_POINT ( 'NONE',  ( -59.64316829561520450, 1385.059617650149903, 243.2224340318209670 ) ) ;
#49338=AXIS2_PLACEMENT_3D ( 'NONE', #55199, #104469, #2594 ) ;
#49345=CARTESIAN_POINT ( 'NONE',  ( -109.8262402379999969, 1384.894770817870040, 311.3808756572590255 ) ) ;
#49357=CARTESIAN_POINT ( 'NONE',  ( -109.1287995176789991, 1384.695877130179952, 311.2584553912229808 ) ) ;
#49359=CARTESIAN_POINT ( 'NONE',  ( -68.59216743310000197, 1379.747776907659954, 280.1820150773590399 ) ) ;
#49361=CARTESIAN_POINT ( 'NONE',  ( -8.820749743162084044, 1381.135727412223105, 217.8385779988905142 ) ) ;
#49372=CARTESIAN_POINT ( 'NONE',  ( -106.3019370990619876, 1378.913060387450059, 306.0560277516660221 ) ) ;
#49396=CARTESIAN_POINT ( 'NONE',  ( -11.24942739399999958, 1391.648629103060102, 213.8067856546890084 ) ) ;
#49398=CARTESIAN_POINT ( 'NONE',  ( -80.38025116429729167, 1384.796184643460037, 283.6024437732969545 ) ) ;
#49438=CARTESIAN_POINT ( 'NONE',  ( -109.8677307403279997, 1383.889131247379964, 311.3700200510110108 ) ) ;
#49454=CARTESIAN_POINT ( 'NONE',  ( -8.890791467111871071, 1388.784675205049780, 217.7635828254234696 ) ) ;
#49471=CARTESIAN_POINT ( 'NONE',  ( -58.94955636626019668, 1384.699952765490025, 279.1418893135149801 ) ) ;
#49472=CARTESIAN_POINT ( 'NONE',  ( -107.3094561203379982, 1391.913060387289988, 301.0960456400809448 ) ) ;
#49478=CARTESIAN_POINT ( 'NONE',  ( -11.24213639542480436, 1378.800280137626714, 204.0324849010276580 ) ) ;
#49489=CARTESIAN_POINT ( 'NONE',  ( -12.39029767569030049, 1378.874140544039847, 211.3238570842829915 ) ) ;
#49499=CARTESIAN_POINT ( 'NONE',  ( -27.71065821358619985, 1379.782896911970056, 216.6336370555119970 ) ) ;
#49502=CARTESIAN_POINT ( 'NONE',  ( -40.71370360497250118, 1379.670045600320009, 229.2404297411889900 ) ) ;
#49531=CARTESIAN_POINT ( 'NONE',  ( -109.8668234651519242, 1385.921405704401877, 311.3699157048114898 ) ) ;
#49538=CARTESIAN_POINT ( 'NONE',  ( -7.611657828410000270, 1379.436956584469954, 206.9293838566389923 ) ) ;
#49547=ORIENTED_EDGE ( 'NONE', *, *, #60651, .F. ) ;
#49550=CARTESIAN_POINT ( 'NONE',  ( -73.57334958110000400, 1384.359832552789840, 298.9349810372589786 ) ) ;
#49563=CARTESIAN_POINT ( 'NONE',  ( -61.45118310290000352, 1388.282453012750011, 249.7659151349589877 ) ) ;
#49565=CARTESIAN_POINT ( 'NONE',  ( -45.48467309282600013, 1385.149558475349977, 252.4883491809910083 ) ) ;
#49581=CIRCLE ( 'NONE', #35248, 7.513435694540000043 ) ;
#49591=CARTESIAN_POINT ( 'NONE',  ( -105.0165902910000000, 1390.482592109759935, 303.1217258594589907 ) ) ;
#49648=ADVANCED_FACE ( 'NONE', ( #12919 ), #19777, .T. ) ;
#49652=VECTOR ( 'NONE', #154, 999.9999999999998863 ) ;
#49669=CARTESIAN_POINT ( 'NONE',  ( -44.90400487128380291, 1384.599132857919813, 218.2254928299460062 ) ) ;
#49684=CARTESIAN_POINT ( 'NONE',  ( -68.77199811340000224, 1379.747924854809980, 280.1875869621590027 ) ) ;
#49700=DIRECTION ( 'NONE',  ( -1.000000000000000000, 0.000000000000000000, 0.000000000000000000 ) ) ;
#49735=CARTESIAN_POINT ( 'NONE',  ( -66.20371065853919390, 1383.789130863189939, 290.1023055280760445 ) ) ;
#49744=CARTESIAN_POINT ( 'NONE',  ( -42.16437246579999254, 1379.922095110709961, 237.2117980744589829 ) ) ;
#49753=CARTESIAN_POINT ( 'NONE',  ( -106.2456710219999962, 1378.874444167599904, 300.8956198461589793 ) ) ;
#49772=CARTESIAN_POINT ( 'NONE',  ( -105.5817487570000139, 1391.853821388999904, 305.4363301085589910 ) ) ;
#49792=EDGE_CURVE ( 'NONE', #26950, #23648, #30624, .T. ) ;
#49801=VERTEX_POINT ( 'NONE', #14570 ) ;
#49803=CARTESIAN_POINT ( 'NONE',  ( -53.46943927250000428, 1384.767240279849830, 230.7494116872589984 ) ) ;
#49815=CARTESIAN_POINT ( 'NONE',  ( -10.74720057723740041, 1391.913060387210180, 205.3639615661770108 ) ) ;
#49835=CIRCLE ( 'NONE', #69517, 7.932410439649999923 ) ;
#49836=CARTESIAN_POINT ( 'NONE',  ( -11.08791805799999963, 1380.264457071439892, 215.5269815452789999 ) ) ;
#49842=CARTESIAN_POINT ( 'NONE',  ( -12.29865477999999968, 1392.006778701819940, 209.7413185055909821 ) ) ;
#49852=CARTESIAN_POINT ( 'NONE',  ( -107.1210572734698729, 1390.321908692038505, 299.4947318525922810 ) ) ;
#49872=CARTESIAN_POINT ( 'NONE',  ( -109.5350879309999925, 1384.896829517670085, 297.1231432122589808 ) ) ;
#49873=ORIENTED_EDGE ( 'NONE', *, *, #31699, .F. ) ;
#49885=CARTESIAN_POINT ( 'NONE',  ( -51.93884728859359967, 1385.026165428789909, 228.3837409096330191 ) ) ;
#49886=CARTESIAN_POINT ( 'NONE',  ( -10.44852243557409999, 1391.913060387289988, 213.6776970188900009 ) ) ;
#49897=CARTESIAN_POINT ( 'NONE',  ( -109.8277101070000015, 1384.853340824010047, 311.3803954542589736 ) ) ;
#49912=CARTESIAN_POINT ( 'NONE',  ( -68.57748934099369365, 1379.747497746340287, 280.1964141449130352 ) ) ;
#49914=CARTESIAN_POINT ( 'NONE',  ( -8.926802433111017621, 1380.976221376709873, 217.7251549208844494 ) ) ;
#49934=CARTESIAN_POINT ( 'NONE',  ( -14.25663218980999858, 1380.283631336060125, 210.3482944585310008 ) ) ;
#49938=CARTESIAN_POINT ( 'NONE',  ( -12.33252012460000024, 1378.517259988440173, 208.8147234668570036 ) ) ;
#49943=CARTESIAN_POINT ( 'NONE',  ( -79.02094512940820437, 1384.789308648159931, 281.7664325557580014 ) ) ;
#49944=VERTEX_POINT ( 'NONE', #67758 ) ;
#49960=CARTESIAN_POINT ( 'NONE',  ( -57.97118228820000496, 1379.732619669730184, 257.2286833013590126 ) ) ;
#49983=FACE_OUTER_BOUND ( 'NONE', #66788, .T. ) ;
#50011=CARTESIAN_POINT ( 'NONE',  ( -12.20132663145084351, 1377.775742761213451, 210.7787750133890086 ) ) ;
#50016=CARTESIAN_POINT ( 'NONE',  ( -51.04490180185960213, 1384.735057055360130, 263.8868331049799849 ) ) ;
#50017=CARTESIAN_POINT ( 'NONE',  ( -106.4061662575890068, 1391.913060387279984, 303.9266446755360676 ) ) ;
#50020=CARTESIAN_POINT ( 'NONE',  ( -107.4284469309999963, 1379.017123567839917, 299.7421770867589998 ) ) ;
#50025=CARTESIAN_POINT ( 'NONE',  ( -10.68354539818558457, 1379.426651953353030, 202.9127243954700646 ) ) ;
#50033=EDGE_CURVE ( 'NONE', #33676, #99683, #105395, .T. ) ;
#50049=CARTESIAN_POINT ( 'NONE',  ( -27.28088378283840143, 1377.835389488949886, 217.2864041108829838 ) ) ;
#50052=CARTESIAN_POINT ( 'NONE',  ( -21.69319346089070066, 1379.597678304780175, 213.6345187343300154 ) ) ;
#50068=FILL_AREA_STYLE ('',( #77470 ) ) ;
#50080=CARTESIAN_POINT ( 'NONE',  ( -106.3976693117229928, 1390.939243848519936, 307.7527733253859878 ) ) ;
#50087=CARTESIAN_POINT ( 'NONE',  ( -26.37171023209999987, 1375.557882964970077, 211.7994354413090150 ) ) ;
#50100=CARTESIAN_POINT ( 'NONE',  ( -109.9987472809999929, 1384.581606379090090, 311.2589846932590376 ) ) ;
#50114=CARTESIAN_POINT ( 'NONE',  ( -67.70705029779999506, 1388.282036916160223, 263.9074574844589733 ) ) ;
#50116=CARTESIAN_POINT ( 'NONE',  ( -47.51462801197750707, 1385.137171588540014, 256.6091612487379621 ) ) ;
#50127=CARTESIAN_POINT ( 'NONE',  ( -8.581225640119999554, 1384.892862025920067, 218.6696712321190148 ) ) ;
#50133=CIRCLE ( 'NONE', #103749, 0.5000000000000029976 ) ;
#50146=CARTESIAN_POINT ( 'NONE',  ( -109.2771419979999905, 1386.778010587349854, 297.3694738813589993 ) ) ;
#50180=CARTESIAN_POINT ( 'NONE',  ( -12.29868253919850041, 1378.334373735910049, 209.9676400962160301 ) ) ;
#50191=VERTEX_POINT ( 'NONE', #38354 ) ;
#50200=CARTESIAN_POINT ( 'NONE',  ( -7.967089726150001106, 1384.601477608269988, 199.5004311937889838 ) ) ;
#50220=CARTESIAN_POINT ( 'NONE',  ( -105.7397520800000166, 1374.768546414190041, 302.6503159984590070 ) ) ;
#50223=CARTESIAN_POINT ( 'NONE',  ( -43.91345046917300010, 1384.595606055820099, 217.0465566091490075 ) ) ;
#50238=CARTESIAN_POINT ( 'NONE',  ( -68.62428177750000202, 1379.748209670530059, 279.8484656398590005 ) ) ;
#50270=CARTESIAN_POINT ( 'NONE',  ( -7.545095448910339897, 1384.908268029229930, 219.0876225167260145 ) ) ;
#50275=EDGE_CURVE ( 'NONE', #74400, #76524, #71700, .T. ) ;
#50295=CARTESIAN_POINT ( 'NONE',  ( -75.11158180925109207, 1383.780721093889952, 299.9085192912519915 ) ) ;
#50303=CARTESIAN_POINT ( 'NONE',  ( -39.07702096660000279, 1382.326711360479976, 238.9772120006589944 ) ) ;
#50307=CARTESIAN_POINT ( 'NONE',  ( -9.102552902454579709, 1386.249080320570101, 218.4336176387340061 ) ) ;
#50313=CARTESIAN_POINT ( 'NONE',  ( -107.8363875370000073, 1380.933530015289989, 298.5630966836590119 ) ) ;
#50336=CARTESIAN_POINT ( 'NONE',  ( -107.2920023509999936, 1387.482252157660241, 310.2753093912590430 ) ) ;
#50391=CARTESIAN_POINT ( 'NONE',  ( -12.11621817370000009, 1378.266527857250139, 211.6883570098989935 ) ) ;
#50397=CARTESIAN_POINT ( 'NONE',  ( -12.77874876509999957, 1390.744078294579822, 206.9966459296790049 ) ) ;
#50405=CARTESIAN_POINT ( 'NONE',  ( -8.883323636877099361, 1384.529732085800106, 218.6638821885779862 ) ) ;
#50420=CARTESIAN_POINT ( 'NONE',  ( -15.13920057018590093, 1383.858439105669959, 219.2872454811189868 ) ) ;
#50433=CARTESIAN_POINT ( 'NONE',  ( -109.1646014829999984, 1384.895722584660007, 297.1326616210590146 ) ) ;
#50437=CARTESIAN_POINT ( 'NONE',  ( -103.5985846424588601, 1379.901892699559312, 304.5993904023399068 ) ) ;
#50441=CARTESIAN_POINT ( 'NONE',  ( -4.145978979534980458E-15, 1375.413060387289988, 209.1218459572589836 ) ) ;
#50444=CARTESIAN_POINT ( 'NONE',  ( -84.36119002024280178, 1385.173936778570123, 288.1322194500510250 ) ) ;
#50446=CARTESIAN_POINT ( 'NONE',  ( -10.88252683822419975, 1391.913060387289988, 212.7915775323999981 ) ) ;
#50470=CARTESIAN_POINT ( 'NONE',  ( -68.58336172453009283, 1379.747483509290078, 280.1906536643289769 ) ) ;
#50495=CARTESIAN_POINT ( 'NONE',  ( -14.13953454557050016, 1379.986141950590081, 211.1479330773270249 ) ) ;
#50503=CARTESIAN_POINT ( 'NONE',  ( -12.41968314810000074, 1391.384630209019861, 211.0556431170890050 ) ) ;
#50504=CARTESIAN_POINT ( 'NONE',  ( -89.28715904204869958, 1384.835856820089930, 292.1171647776239979 ) ) ;
#50511=EDGE_LOOP ( 'NONE', ( #27466, #80734, #60864, #95726 ) ) ;
#50520=CARTESIAN_POINT ( 'NONE',  ( -58.01117002480000195, 1379.721643371590289, 257.2111322587590507 ) ) ;
#50552=CARTESIAN_POINT ( 'NONE',  ( -8.082394523001108055, 1387.362642507876217, 218.5730659734533390 ) ) ;
#50569=CARTESIAN_POINT ( 'NONE',  ( -51.99793925633279912, 1384.730550586590198, 265.8323962730830203 ) ) ;
#50572=CARTESIAN_POINT ( 'NONE',  ( -107.4538559780000071, 1379.578066771490057, 299.0810615966589694 ) ) ;
#50576=CARTESIAN_POINT ( 'NONE',  ( -9.803547299931144821, 1380.487226564378943, 201.5547637714570328 ) ) ;
#50593=CARTESIAN_POINT ( 'NONE',  ( -7.463281564165999526, 1379.014324719059914, 211.6703187352700013 ) ) ;
#50595=CARTESIAN_POINT ( 'NONE',  ( -40.60195937901799823, 1379.651450217159891, 229.3176569930949995 ) ) ;
#50626=CARTESIAN_POINT ( 'NONE',  ( 2.285812126927549962E-14, 1380.413060387289988, 208.3364477938620212 ) ) ;
#50632=CARTESIAN_POINT ( 'NONE',  ( -105.5086933517860075, 1378.552678757879903, 304.0434870558410125 ) ) ;
#50643=CARTESIAN_POINT ( 'NONE',  ( -109.2093473777249955, 1385.425682697149796, 295.1563182021879470 ) ) ;
#50654=CARTESIAN_POINT ( 'NONE',  ( -47.49417614000000043, 1386.750003725609986, 256.2226892774589828 ) ) ;
#50656=CARTESIAN_POINT ( 'NONE',  ( -59.28183620200640291, 1385.069713019159963, 279.7253289016610438 ) ) ;
#50663=CARTESIAN_POINT ( 'NONE',  ( -8.580842993890000159, 1384.881883552430054, 218.6695867492290120 ) ) ;
#50664=DIRECTION ( 'NONE',  ( 1.836970198721029688E-16, 1.000000000000000000, -2.953460612019999929E-19 ) ) ;
#50665=CARTESIAN_POINT ( 'NONE',  ( -107.6465574917919952, 1382.804371864389850, 310.6282975730970293 ) ) ;
#50701=CARTESIAN_POINT ( 'NONE',  ( -13.12553473323018416, 1379.406084055735619, 211.7521813457520636 ) ) ;
#50711=CARTESIAN_POINT ( 'NONE',  ( -12.29845482411220026, 1378.332941950110126, 209.9703957929920080 ) ) ;
#50725=CARTESIAN_POINT ( 'NONE',  ( -110.0628831554700042, 1384.910109443090050, 296.9513044379630173 ) ) ;
#50737=ORIENTED_EDGE ( 'NONE', *, *, #74658, .T. ) ;
#50745=CARTESIAN_POINT ( 'NONE',  ( -109.5441724430000079, 1374.437034645689891, 303.4364478832590066 ) ) ;
#50754=CARTESIAN_POINT ( 'NONE',  ( -35.92330893652459878, 1384.571147577790043, 209.4208511670099995 ) ) ;
#50762=CARTESIAN_POINT ( 'NONE',  ( -68.39223289816457907, 1379.747175533331301, 280.0421571237133094 ) ) ;
#50767=CARTESIAN_POINT ( 'NONE',  ( -68.75005492889998493, 1379.747908384619905, 280.1011935185590005 ) ) ;
#50768=CIRCLE ( 'NONE', #29342, 7.842199003069996621 ) ;
#50782=EDGE_CURVE ( 'NONE', #17951, #26163, #48412, .T. ) ;
#50794=CARTESIAN_POINT ( 'NONE',  ( 2.283436972078669822E-15, 1391.413060387289988, 209.1218459572589836 ) ) ;
#50825=CARTESIAN_POINT ( 'NONE',  ( -63.13574013807390628, 1383.792676540780121, 285.6932720343630194 ) ) ;
#50833=CARTESIAN_POINT ( 'NONE',  ( -38.64161925439999834, 1383.830331748989920, 239.2263113910589993 ) ) ;
#50844=CARTESIAN_POINT ( 'NONE',  ( -109.5297118039999873, 1383.965857270459992, 297.1689209028589858 ) ) ;
#50846=CARTESIAN_POINT ( 'NONE',  ( -109.1656546792999904, 1384.956445601399992, 297.1328575267269798 ) ) ;
#50868=CARTESIAN_POINT ( 'NONE',  ( -107.9182817679999857, 1387.176265556199951, 310.5436438242589929 ) ) ;
#50873=EDGE_CURVE ( 'NONE', #40166, #103332, #12740, .T. ) ;
#50877=CARTESIAN_POINT ( 'NONE',  ( -12.85016526419999927, 1389.184315283510159, 203.6059765727289914 ) ) ;
#50916=VERTEX_POINT ( 'NONE', #77389 ) ;
#50931=FACE_OUTER_BOUND ( 'NONE', #13958, .T. ) ;
#50940=CARTESIAN_POINT ( 'NONE',  ( -106.4480417398009848, 1384.930840067430154, 311.2385799845050087 ) ) ;
#50942=CARTESIAN_POINT ( 'NONE',  ( -10.10234689610000203, 1389.151301037549956, 201.8686386834390305 ) ) ;
#50947=CARTESIAN_POINT ( 'NONE',  ( -8.874427328269188564, 1384.581418649760053, 218.6695361999740044 ) ) ;
#50973=CARTESIAN_POINT ( 'NONE',  ( -110.0630399400000101, 1384.905426682000098, 296.9512818274590131 ) ) ;
#50982=CARTESIAN_POINT ( 'NONE',  ( -108.4664300161794586, 1381.328991949513011, 310.3998206309821057 ) ) ;
#50985=CARTESIAN_POINT ( 'NONE',  ( -11.90322536250000063, 1391.913060490810039, 209.2366397656629999 ) ) ;
#50986=CARTESIAN_POINT ( 'NONE',  ( -77.18387175459460536, 1385.145919355859860, 279.0577792721099968 ) ) ;
#50987=CARTESIAN_POINT ( 'NONE',  ( -11.13475278476130015, 1391.913060387289988, 212.1805052186929856 ) ) ;
#51030=EDGE_CURVE ( 'NONE', #35724, #47452, #32404, .T. ) ;
#51032=ORIENTED_EDGE ( 'NONE', *, *, #78217, .F. ) ;
#51044=CARTESIAN_POINT ( 'NONE',  ( -9.123736379228210680, 1384.508619151900120, 199.9712811155520171 ) ) ;
#51046=CARTESIAN_POINT ( 'NONE',  ( -12.27558643790000126, 1391.355947405540064, 211.6931146936589982 ) ) ;
#51047=CARTESIAN_POINT ( 'NONE',  ( -93.07309726766789026, 1384.850428360820160, 294.1733350510500031 ) ) ;
#51066=CARTESIAN_POINT ( 'NONE',  ( -51.76145802239999938, 1379.744278086280019, 243.7243931585590246 ) ) ;
#51111=ORIENTED_EDGE ( 'NONE', *, *, #44567, .F. ) ;
#51115=CARTESIAN_POINT ( 'NONE',  ( -12.08843586217701827, 1377.632273357547774, 211.4485156452657861 ) ) ;
#51120=CARTESIAN_POINT ( 'NONE',  ( -72.47816579847129503, 1384.655904266999869, 297.6885493325589778 ) ) ;
#51127=CARTESIAN_POINT ( 'NONE',  ( -10.29023455615431537, 1379.884657259707410, 202.2562532116602085 ) ) ;
#51136=CARTESIAN_POINT ( 'NONE',  ( -11.00370989719999848, 1381.644652005500120, 201.9116486243489987 ) ) ;
#51147=CARTESIAN_POINT ( 'NONE',  ( -56.86315681117869758, 1379.712756814529939, 259.5172876196859875 ) ) ;
#51153=CARTESIAN_POINT ( 'NONE',  ( -107.0879710039999964, 1379.224539023319949, 308.6385636590589456 ) ) ;
#51182=CARTESIAN_POINT ( 'NONE',  ( -105.5653050470969987, 1378.245869374329914, 304.5467815922049795 ) ) ;
#51203=CARTESIAN_POINT ( 'NONE',  ( -67.88104421250000087, 1388.175118100200052, 291.5606887542589902 ) ) ;
#51205=CARTESIAN_POINT ( 'NONE',  ( -72.06849244676079991, 1385.017144407860087, 297.2881297217280121 ) ) ;
#51215=CARTESIAN_POINT ( 'NONE',  ( -109.4369740319060185, 1383.303469659739903, 311.1345803559980254 ) ) ;
#51227=CARTESIAN_POINT ( 'NONE',  ( -109.1483069509999950, 1386.118696371760052, 297.2762669758590164 ) ) ;
#51260=CARTESIAN_POINT ( 'NONE',  ( -12.30432296583530061, 1378.363065960840231, 209.8932745738640051 ) ) ;
#51265=CARTESIAN_POINT ( 'NONE',  ( -105.6883471066019951, 1379.461008901829928, 304.2217744859839854 ) ) ;
#51278=CARTESIAN_POINT ( 'NONE',  ( -9.123736304069998582, 1384.508619150859886, 199.9712811105490289 ) ) ;
#51299=CARTESIAN_POINT ( 'NONE',  ( -30.86955864515919856, 1384.558263882109941, 206.0685599762870197 ) ) ;
#51306=CARTESIAN_POINT ( 'NONE',  ( -33.52629754523064065, 1379.638293383748078, 221.4617334473517190 ) ) ;
#51311=CARTESIAN_POINT ( 'NONE',  ( -68.70865610920000677, 1379.748126065489942, 280.0489821606589658 ) ) ;
#51319=CARTESIAN_POINT ( 'NONE',  ( -3.078458293570000226, 1385.048553955020225, 218.5738910584090036 ) ) ;
#51367=CARTESIAN_POINT ( 'NONE',  ( -54.11663967002189679, 1383.805289491930125, 269.6990428264840034 ) ) ;
#51378=CARTESIAN_POINT ( 'NONE',  ( -36.68365415889999781, 1382.326063136570156, 235.1111881889589768 ) ) ;
#51385=LINE ( 'NONE', #85517, #24214 ) ;
#51391=CARTESIAN_POINT ( 'NONE',  ( -108.5373427389999961, 1383.177762179680030, 297.5067995922590285 ) ) ;
#51414=CARTESIAN_POINT ( 'NONE',  ( -104.9846310909999971, 1389.412964589189869, 307.6627679757589817 ) ) ;
#51475=CARTESIAN_POINT ( 'NONE',  ( -11.46268780760000006, 1379.176763712969887, 214.2011949338190107 ) ) ;
#51484=CARTESIAN_POINT ( 'NONE',  ( -13.85278479829999831, 1390.202287805009973, 206.8926036963289903 ) ) ;
#51518=CARTESIAN_POINT ( 'NONE',  ( -109.1649475050000007, 1384.884072125880039, 297.1327577457590223 ) ) ;
#51521=CARTESIAN_POINT ( 'NONE',  ( -12.24215919237970063, 1392.317484695480061, 210.7023522567849909 ) ) ;
#51527=CARTESIAN_POINT ( 'NONE',  ( -107.6245944317399506, 1380.278007003908897, 309.5812188244966023 ) ) ;
#51529=CARTESIAN_POINT ( 'NONE',  ( -12.47575469030000050, 1379.153285202859934, 210.8825669665690157 ) ) ;
#51530=CARTESIAN_POINT ( 'NONE',  ( -12.55604107059999919, 1391.387401865550146, 208.6966032511679714 ) ) ;
#51531=CARTESIAN_POINT ( 'NONE',  ( -72.30449149428240219, 1385.123662558519982, 270.5213631660990359 ) ) ;
#51532=CARTESIAN_POINT ( 'NONE',  ( -11.54851213157500212, 1391.913060387289988, 210.7248915062780270 ) ) ;
#51561=CARTESIAN_POINT ( 'NONE',  ( -68.77190087506669158, 1379.747925807530009, 280.3125204381590265 ) ) ;
#51589=CARTESIAN_POINT ( 'NONE',  ( -14.24503472313680064, 1380.268785586849845, 210.4293653685249978 ) ) ;
#51597=CARTESIAN_POINT ( 'NONE',  ( -86.96400225606849688, 1384.826294148989973, 290.4385014204809750 ) ) ;
#51615=CARTESIAN_POINT ( 'NONE',  ( -25.98205113330000060, 1379.634954421569773, 211.5700168387090230 ) ) ;
#51628=ORIENTED_EDGE ( 'NONE', *, *, #22691, .F. ) ;
#51635=CARTESIAN_POINT ( 'NONE',  ( -12.51034970659999956, 1378.851356593469973, 207.9031378000489951 ) ) ;
#51639=CARTESIAN_POINT ( 'NONE',  ( -110.0662890209999887, 1385.104992454720104, 296.9550740769589652 ) ) ;
#51642=VERTEX_POINT ( 'NONE', #101604 ) ;
#51671=CARTESIAN_POINT ( 'NONE',  ( -63.30236682719129959, 1384.683505265780013, 286.2651546391219881 ) ) ;
#51672=CARTESIAN_POINT ( 'NONE',  ( -9.094129269030000629, 1384.954944735329946, 199.9429221374590213 ) ) ;
#51688=CARTESIAN_POINT ( 'NONE',  ( -9.528525097359999307, 1381.369362415970045, 201.1489852242889924 ) ) ;
#51703=CARTESIAN_POINT ( 'NONE',  ( -65.35806189339839989, 1379.740364976560159, 275.4909032779769973 ) ) ;
#51711=CARTESIAN_POINT ( 'NONE',  ( -7.785551154210000213, 1385.415854725780036, 218.8883729281390060 ) ) ;
#51722=SURFACE_STYLE_FILL_AREA ( #50068 ) ;
#51740=CARTESIAN_POINT ( 'NONE',  ( -35.62143398542752237, 1379.642029864801543, 218.5761008737005398 ) ) ;
#51741=CARTESIAN_POINT ( 'NONE',  ( -3.771520288500000539, 1375.389610323599982, 208.3364477064349956 ) ) ;
#51755=CARTESIAN_POINT ( 'NONE',  ( -106.4197298790000019, 1384.588767362379940, 311.3121942672589739 ) ) ;
#51767=CARTESIAN_POINT ( 'NONE',  ( -85.78494180500000255, 1386.745275533519816, 289.7710778616590233 ) ) ;
#51769=CARTESIAN_POINT ( 'NONE',  ( -63.98031756861389852, 1385.047684693189922, 287.2751599999480163 ) ) ;
#51779=CARTESIAN_POINT ( 'NONE',  ( -106.9567297613849917, 1382.281980269420046, 310.2341151030279320 ) ) ;
#51807=CARTESIAN_POINT ( 'NONE',  ( -12.99960798169789911, 1384.882413778849923, 219.0844187336040250 ) ) ;
#51829=CARTESIAN_POINT ( 'NONE',  ( -109.9698195215979979, 1384.452562162210143, 311.4357956501490321 ) ) ;
#51836=ORIENTED_EDGE ( 'NONE', *, *, #74750, .F. ) ;
#51871=CARTESIAN_POINT ( 'NONE',  ( -31.92565964530000144, 1384.834792386509889, 206.3014967088990090 ) ) ;
#51872=CARTESIAN_POINT ( 'NONE',  ( -63.95720680553800008, 1384.698108589110234, 252.7292494320779781 ) ) ;
#51884=CARTESIAN_POINT ( 'NONE',  ( -68.44345568869999852, 1379.747786969579920, 279.4410717829589430 ) ) ;
#51891=CARTESIAN_POINT ( 'NONE',  ( -17.47467951480000181, 1385.286067972039973, 219.9356668727590147 ) ) ;
#51893=CARTESIAN_POINT ( 'NONE',  ( -16.22920744153299921, 1385.290408393959979, 219.6908716482870148 ) ) ;
#51901=VECTOR ( 'NONE', #40488, 1000.000000000000000 ) ;
#51916=AXIS2_PLACEMENT_3D ( 'NONE', #11751, #26904, #78411 ) ;
#51935=CARTESIAN_POINT ( 'NONE',  ( -56.13545839238830126, 1383.802202486730039, 273.6217168716430024 ) ) ;
#51937=CARTESIAN_POINT ( 'NONE',  ( -107.5501839752090234, 1379.272371746452563, 299.1643430017058449 ) ) ;
#51943=CARTESIAN_POINT ( 'NONE',  ( -73.20427770220000241, 1380.595915926100133, 278.0678802370590006 ) ) ;
#51944=DIRECTION ( 'NONE',  ( -1.000000000000000000, 1.836970198721029688E-16, 0.000000000000000000 ) ) ;
#51955=CARTESIAN_POINT ( 'NONE',  ( -110.0634902310000030, 1384.899971913130003, 296.9512050679589947 ) ) ;
#51966=ORIENTED_EDGE ( 'NONE', *, *, #74064, .F. ) ;
#51977=CARTESIAN_POINT ( 'NONE',  ( -106.7877995600000105, 1387.660326901150029, 310.1072176132589675 ) ) ;
#52030=ADVANCED_FACE ( 'NONE', ( #31529, #57323 ), #72460, .T. ) ;
#52032=CARTESIAN_POINT ( 'NONE',  ( -8.757904425059999554, 1386.987225607769915, 218.3429050645090115 ) ) ;
#52041=CARTESIAN_POINT ( 'NONE',  ( -8.401610822820000379, 1382.692138962740046, 218.3897665777690236 ) ) ;
#52048=CARTESIAN_POINT ( 'NONE',  ( -13.97245352320000045, 1390.368340403819957, 209.8294132315500349 ) ) ;
#52053=CARTESIAN_POINT ( 'NONE',  ( -8.921303631935559864, 1384.360432746769902, 218.6413268481589967 ) ) ;
#52069=CARTESIAN_POINT ( 'NONE',  ( -10.89134688618890046, 1383.862286347570034, 218.6605473698739956 ) ) ;
#52086=CARTESIAN_POINT ( 'NONE',  ( -13.62718107187109950, 1390.427313303139954, 210.7651432677700143 ) ) ;
#52093=CARTESIAN_POINT ( 'NONE',  ( -10.25368835369999942, 1391.913060387289988, 204.2726076338790051 ) ) ;
#52094=CARTESIAN_POINT ( 'NONE',  ( -81.68439207092418997, 1385.164090965520018, 285.2251458109799955 ) ) ;
#52123=B_SPLINE_CURVE_WITH_KNOTS ( 'NONE', 3,
 ( #30880, #55020, #74009, #108141, #99174, #56656, #90790, #14072, #48261, #82405, #31433, #65615 ),
 .UNSPECIFIED., .F., .F.,
 ( 4, 2, 2, 2, 2, 4 ),
 ( -0.08222331866850060567, -0.06445908733047370220, -0.04475466563503439910, -0.02302985374697249371, 0.000000000000000000, 0.0003446917825884465714 ),
 .UNSPECIFIED. ) ;
#52134=CARTESIAN_POINT ( 'NONE',  ( -12.42519068387639969, 1378.686196775090139, 209.1401553900249723 ) ) ;
#52156=CARTESIAN_POINT ( 'NONE',  ( -91.57517030605119146, 1384.844808691319940, 293.4524694912760197 ) ) ;
#52176=CARTESIAN_POINT ( 'NONE',  ( -14.15052379810000005, 1379.587026329759965, 207.9895299807990057 ) ) ;
#52232=CARTESIAN_POINT ( 'NONE',  ( -64.65996261591139671, 1384.678844644059836, 288.2602538484970296 ) ) ;
#52239=CARTESIAN_POINT ( 'NONE',  ( -7.545064063707340729, 1384.907232462019920, 219.0876311385090105 ) ) ;
#52253=CARTESIAN_POINT ( 'NONE',  ( -8.029416465979998918, 1383.927159441839876, 199.5752583396389923 ) ) ;
#52268=CARTESIAN_POINT ( 'NONE',  ( -66.42203761300000053, 1379.747445253800151, 277.0326445461590197 ) ) ;
#52274=CARTESIAN_POINT ( 'NONE',  ( -106.6765851849999933, 1378.991158695870126, 307.6173790219590387 ) ) ;
#52301=CARTESIAN_POINT ( 'NONE',  ( -24.68953382638999372, 1379.615025458047285, 210.8754759576296181 ) ) ;
#52311=VERTEX_POINT ( 'NONE', #2248 ) ;
#52321=EDGE_CURVE ( 'NONE', #82812, #103332, #43119, .T. ) ;
#52332=CARTESIAN_POINT ( 'NONE',  ( -81.69295930340000211, 1388.108283263359908, 304.1383302712590080 ) ) ;
#52344=CARTESIAN_POINT ( 'NONE',  ( -108.0278876277179876, 1382.536111722130045, 310.5170612373680115 ) ) ;
#52373=CARTESIAN_POINT ( 'NONE',  ( -19.06115223335860165, 1384.865189719420187, 220.5788536041530108 ) ) ;
#52396=CARTESIAN_POINT ( 'NONE',  ( -105.6009733815480018, 1377.068166733269891, 306.8927961940029832 ) ) ;
#52422=B_SPLINE_SURFACE_WITH_KNOTS ( 'NONE', 5, 5, ( 
 ( #47834, #38317, #5274, #71975, #89281, #73041 ),
 ( #54610, #30472, #3658, #63566, #39430, #97681 ),
 ( #107735, #31020, #20955, #56791, #90928, #55159 ),
 ( #48400, #46759, #14215, #59006, #50052, #101514 ),
 ( #58448, #85273, #33226, #57365, #16945, #8024 ),
 ( #15309, #15846, #75257, #83627, #6923, #110493 ),
 ( #14770, #67969, #41080, #212, #8573, #76905 ),
 ( #92037, #67415, #23717, #99866, #84180, #92575 ),
 ( #57903, #33773, #49502, #7479, #50595, #109406 ),
 ( #48956, #32682, #109947, #65749, #41640, #75796 ),
 ( #83087, #24801, #93133, #76344, #40528, #32132 ),
 ( #91490, #16401, #23165, #24267, #84727, #66862 ),
 ( #42743, #42192, #100971, #6380, #108835, #74704 ),
 ( #102077, #25360, #59552, #93666, #51147, #66317 ),
 ( #100435, #26476, #104303, #60671, #756, #61240 ),
 ( #62334, #68515, #70197, #43305, #53939, #25914 ),
 ( #9681, #103174, #9142, #45533, #10804, #102614 ),
 ( #19163, #94798, #43849, #77454, #87515, #86945 ),
 ( #88074, #34337, #34884, #18614, #44413, #94230 ),
 ( #60112, #10237, #79672, #103752, #78554, #18073 ),
 ( #11361, #1871, #35442, #17504, #69073, #51703 ),
 ( #69630, #44974, #2430, #77996, #19739, #27594 ),
 ( #52268, #86392, #61778, #1302, #27054, #95354 ),
 ( #96459, #85843, #95902, #52814, #36004, #53369 ),
 ( #79122, #36546, #70743, #104855, #28144, #47708 ),
 ( #63440, #89153, #21910, #105972, #56106, #98092 ),
 ( #38193, #72914, #20831, #107053, #88621, #29249 ),
 ( #21365, #38737, #73469, #54485, #81289, #107603 ),
 ( #13520, #80760, #14079, #12441, #3525, #81837 ),
 ( #56662, #22461, #62908, #2977, #11901, #30338 ),
 ( #90797, #72375, #46076, #105411, #55573, #98643 ),
 ( #97557, #63982, #46626, #55026, #4068, #5141 ),
 ( #97019, #39297, #106504, #48268, #37096, #71297 ),
 ( #29793, #4603, #71855, #28703, #89697, #12978 ),
 ( #80207, #47161, #64529, #20280, #90238, #30886 ),
 ( #65066, #99182, #37650, #57229, #93537, #58862 ),
 ( #16268, #67277, #108703, #57778, #14639, #24661 ),
 ( #84046, #101934, #82413, #82948, #66729, #92434 ),
 ( #48824, #74014, #24122, #16808, #40945, #15710 ),
 ( #6240, #25221, #58312, #83488, #65622, #40390 ),
 ( #49359, #74567, #59425, #50470, #92992, #49912 ),
 ( #110351, #108149, #109270, #67822, #7345, #41508 ),
 ( #75122, #109810, #75667, #31995, #5706, #100303 ),
 ( #100833, #66183, #23587, #33090, #84594, #7885 ),
 ( #76206, #31438, #32554, #101371, #91896, #39852 ),
 ( #99735, #6783, #23027, #42055, #91359, #33628 ),
 ( #15173, #69487, #86806, #10665, #102488, #18473 ),
 ( #103036, #61630, #17923, #62189, #60529, #51561 ) ),
 .UNSPECIFIED., .F., .F., .F.,
 ( 6, 3, 3, 3, 3, 3, 3, 3, 3, 3, 3, 3, 3, 3, 3, 6 ),
 ( 6, 6 ),
 ( 51.34180956679009711, 70.71758386339999447, 85.59913247730000307, 120.0240483330000103, 152.6368677490000039, 161.9753697619999855, 171.3110621919999801, 176.9610724089999962, 178.9129053279999937, 179.8972017420000213, 180.8814981559999922, 181.2916321369999935, 181.4966991269999994, 181.7017661169999769, 181.8155171619999919, 182.0375288639999951 ),
 ( 0.000000000000000000, 0.5002064398120489308 ),
 .UNSPECIFIED. ) ;
#52424=CARTESIAN_POINT ( 'NONE',  ( -70.04184978290001595, 1375.054395627170152, 279.7464857826589650 ) ) ;
#52430=CARTESIAN_POINT ( 'NONE',  ( -85.86509717699999555, 1384.940999761789953, 289.6770174195589789 ) ) ;
#52431=CARTESIAN_POINT ( 'NONE',  ( -50.04736368845490091, 1384.619862122030099, 225.3512856688030297 ) ) ;
#52435=ORIENTED_EDGE ( 'NONE', *, *, #56465, .F. ) ;
#52442=CARTESIAN_POINT ( 'NONE',  ( -68.37764721770000165, 1379.747183406850127, 279.2177063942590394 ) ) ;
#52451=CARTESIAN_POINT ( 'NONE',  ( -25.93734973360000140, 1384.843007074499837, 224.2459728783589981 ) ) ;
#52453=CARTESIAN_POINT ( 'NONE',  ( -11.00028806098080025, 1385.308172297210149, 218.8195870429669867 ) ) ;
#52463=CARTESIAN_POINT ( 'NONE',  ( -8.885472218384601106, 1385.297170050430168, 218.6625727627470042 ) ) ;
#52495=CARTESIAN_POINT ( 'NONE',  ( -81.92975575952578993, 1383.775620875610002, 304.8532181189869448 ) ) ;
#52496=CARTESIAN_POINT ( 'NONE',  ( -107.9702631612849046, 1378.913060387289988, 299.5275268628465710 ) ) ;
#52502=CARTESIAN_POINT ( 'NONE',  ( -87.83602971100000900, 1380.693317143970035, 294.3638560435589966 ) ) ;
#52512=CARTESIAN_POINT ( 'NONE',  ( -108.4220066540000005, 1383.250329722910010, 297.4825366361590113 ) ) ;
#52526=DIRECTION ( 'NONE',  ( -1.076084536626781954E-17, -1.000000000000000000, -4.313860721084074369E-17 ) ) ;
#52563=ORIENTED_EDGE ( 'NONE', *, *, #61205, .F. ) ;
#52586=CARTESIAN_POINT ( 'NONE',  ( -5.964141498479999193, 1386.998390782689967, 218.2806129090890011 ) ) ;
#52595=CARTESIAN_POINT ( 'NONE',  ( -9.622416126109998302, 1382.582223343250007, 217.9576506642389973 ) ) ;
#52618=CIRCLE ( 'NONE', #75872, 2.500000000000002220 ) ;
#52621=CARTESIAN_POINT ( 'NONE',  ( -10.57073115472060110, 1383.862563487480202, 218.6316618481800162 ) ) ;
#52629=CARTESIAN_POINT ( 'NONE',  ( -9.839360847350000938, 1382.942182113030185, 200.0986700951989974 ) ) ;
#52636=CARTESIAN_POINT ( 'NONE',  ( -13.20168566553750011, 1390.473793852909921, 211.6634096005309971 ) ) ;
#52644=CARTESIAN_POINT ( 'NONE',  ( -74.96301731579400496, 1385.136118946299803, 275.4036379574320108 ) ) ;
#52646=CARTESIAN_POINT ( 'NONE',  ( -50.59433295680000242, 1379.743302990699931, 241.3342481622590014 ) ) ;
#52651=CARTESIAN_POINT ( 'NONE',  ( -9.239957267063561019, 1384.847616872940080, 197.9484498896830189 ) ) ;
#52684=CARTESIAN_POINT ( 'NONE',  ( -12.40250920638250065, 1378.632933055699823, 209.1856888407239978 ) ) ;
#52702=AXIS2_PLACEMENT_3D ( 'NONE', #104267, #52772, #86910 ) ;
#52707=CARTESIAN_POINT ( 'NONE',  ( -89.81305537822530027, 1384.837953921539793, 292.4503084444569936 ) ) ;
#52724=CARTESIAN_POINT ( 'NONE',  ( -32.66522595970000253, 1379.629515683599948, 215.9478188136090182 ) ) ;
#52745=CARTESIAN_POINT ( 'NONE',  ( -14.17772861730700207, 1379.591530685439920, 207.8208986668599891 ) ) ;
#52758=CARTESIAN_POINT ( 'NONE',  ( -13.09309660601929970, 1379.413120505010056, 208.1547604687910109 ) ) ;
#52768=DIRECTION ( 'NONE',  ( -0.05489692781948048161, 0.01152269768267543196, -0.9984255379116142581 ) ) ;
#52772=DIRECTION ( 'NONE',  ( -1.836970198721029688E-16, -1.000000000000000000, 0.000000000000000000 ) ) ;
#52778=CARTESIAN_POINT ( 'NONE',  ( -68.46353614679770772, 1384.666907584059800, 293.2737738776249898 ) ) ;
#52779=CARTESIAN_POINT ( 'NONE',  ( -25.34732223421400121, 1384.960228105589977, 203.3983496752080100 ) ) ;
#52799=CARTESIAN_POINT ( 'NONE',  ( -7.567241880450000124, 1385.515695150829970, 219.0512258816089854 ) ) ;
#52801=CARTESIAN_POINT ( 'NONE',  ( -9.362782585499999755, 1381.058213305800109, 200.9707292486589836 ) ) ;
#52814=CARTESIAN_POINT ( 'NONE',  ( -66.96278127175379780, 1379.743653987389962, 277.9592658266520289 ) ) ;
#52821=AXIS2_PLACEMENT_3D ( 'NONE', #48872, #82998, #58358 ) ;
#52851=CARTESIAN_POINT ( 'NONE',  ( -49.19594470377145257, 1379.685644944692058, 238.0301645601815892 ) ) ;
#52879=CARTESIAN_POINT ( 'NONE',  ( -89.95656494280000004, 1388.077005338320077, 307.8707420459589912 ) ) ;
#52890=CARTESIAN_POINT ( 'NONE',  ( -108.6040716729050075, 1381.990087626129935, 310.5709923410640272 ) ) ;
#52907=AXIS2_PLACEMENT_3D ( 'NONE', #38087, #29679, #73350 ) ;
#52908=CARTESIAN_POINT ( 'NONE',  ( -113.4000000000000057, 1384.899971913130003, 304.2218459572590064 ) ) ;
#52917=CARTESIAN_POINT ( 'NONE',  ( -13.73849276585309909, 1384.880433421959879, 219.2007748097859690 ) ) ;
#52927=ORIENTED_EDGE ( 'NONE', *, *, #35715, .F. ) ;
#52974=B_SPLINE_CURVE_WITH_KNOTS ( 'NONE', 5,
 ( #38235, #38783, #98137, #106550, #29838, #22503, #48314, #37695, #90840 ),
 .UNSPECIFIED., .F., .F.,
 ( 6, 3, 6 ),
 ( 0.000000000000000000, 0.4999997632602161679, 1.000000000000000000 ),
 .UNSPECIFIED. ) ;
#52976=CARTESIAN_POINT ( 'NONE',  ( -95.07903399769999453, 1377.031630663760097, 300.1294849942590304 ) ) ;
#52977=CARTESIAN_POINT ( 'NONE',  ( -106.1512004960610085, 1378.913060387289988, 302.5374961247920282 ) ) ;
#52982=CARTESIAN_POINT ( 'NONE',  ( -57.22511502587629906, 1384.656476375839929, 238.2158304579979813 ) ) ;
#52994=CARTESIAN_POINT ( 'NONE',  ( -66.90724276829999440, 1379.748944712210005, 276.4281807783590352 ) ) ;
#53003=CARTESIAN_POINT ( 'NONE',  ( -13.36175619390000158, 1385.161385112729931, 218.9601252273889997 ) ) ;
#53005=CARTESIAN_POINT ( 'NONE',  ( -17.52406974176239629, 1385.285689121970108, 220.0437453706010160 ) ) ;
#53048=CARTESIAN_POINT ( 'NONE',  ( -101.2580338645349940, 1383.763198325070107, 310.7707653970629735 ) ) ;
#53049=CARTESIAN_POINT ( 'NONE',  ( -109.6263796463910012, 1384.395362625620010, 311.2927007664749794 ) ) ;
#53055=CARTESIAN_POINT ( 'NONE',  ( -76.26096196870000199, 1380.057134384339861, 296.1664118935590295 ) ) ;
#53057=CARTESIAN_POINT ( 'NONE',  ( -1.102182119232619883E-15, 1378.913060387289988, 209.1218459572589836 ) ) ;
#53065=CARTESIAN_POINT ( 'NONE',  ( 9.708065270058002127, 1384.913060387289988, 216.1751682406138571 ) ) ;
#53066=CARTESIAN_POINT ( 'NONE',  ( -107.7002785469999964, 1382.621911665969947, 297.8537995400589580 ) ) ;
#53139=CARTESIAN_POINT ( 'NONE',  ( -6.165516677240000298, 1391.030806526970082, 208.7341617952090189 ) ) ;
#53161=CARTESIAN_POINT ( 'NONE',  ( -12.31743044086090144, 1378.338386037660030, 209.6284750056420023 ) ) ;
#53175=CARTESIAN_POINT ( 'NONE',  ( -27.96151500746649887, 1383.844585648530028, 225.8420327614329892 ) ) ;
#53183=CARTESIAN_POINT ( 'NONE',  ( -9.258223055952665703, 1388.601410234513878, 200.8677487422715728 ) ) ;
#53190=CARTESIAN_POINT ( 'NONE',  ( -12.29865557582230018, 1392.006777630620036, 209.7412721249799858 ) ) ;
#53199=CARTESIAN_POINT ( 'NONE',  ( -12.06041275870000185, 1391.852782912460043, 208.2296565975740066 ) ) ;
#53200=CARTESIAN_POINT ( 'NONE',  ( -94.11294163072489027, 1385.205045773489928, 294.6186134169249726 ) ) ;
#53207=ORIENTED_EDGE ( 'NONE', *, *, #34372, .F. ) ;
#53242=CARTESIAN_POINT ( 'NONE',  ( -14.01094583181789943, 1379.700363488999983, 208.2836208941100153 ) ) ;
#53280=CARTESIAN_POINT ( 'NONE',  ( -109.7922251892066043, 1383.411727247472299, 297.1256090396871627 ) ) ;
#53282=CARTESIAN_POINT ( 'NONE',  ( -21.19337473369999714, 1379.596559222110045, 209.5042946936439989 ) ) ;
#53317=CARTESIAN_POINT ( 'NONE',  ( -12.33253358726570070, 1378.517501885649835, 208.8148673690130011 ) ) ;
#53334=AXIS2_PLACEMENT_3D ( 'NONE', #4834, #107303, #30596 ) ;
#53337=CARTESIAN_POINT ( 'NONE',  ( -77.49021889145849684, 1384.643977683190087, 302.0747173313980056 ) ) ;
#53338=CARTESIAN_POINT ( 'NONE',  ( -44.91689487631180100, 1385.002850385320016, 218.2146715890750102 ) ) ;
#53345=CARTESIAN_POINT ( 'NONE',  ( -7.965967244980000750, 1384.921491711900217, 199.4892246039989914 ) ) ;
#53353=CARTESIAN_POINT ( 'NONE',  ( -106.9545585610730001, 1391.913060387289988, 306.5861216815010266 ) ) ;
#53357=CARTESIAN_POINT ( 'NONE',  ( -8.108123535929999903, 1383.554056671639955, 199.6539754186189839 ) ) ;
#53369=CARTESIAN_POINT ( 'NONE',  ( -66.93736618710819641, 1379.743976683229903, 277.9760783128850221 ) ) ;
#53370=VERTEX_POINT ( 'NONE', #69120 ) ;
#53371=ORIENTED_EDGE ( 'NONE', *, *, #84635, .F. ) ;
#53381=CARTESIAN_POINT ( 'NONE',  ( -105.9085581613829845, 1378.913060388459826, 305.0251771309630158 ) ) ;
#53386=DIRECTION ( 'NONE',  ( 6.332794898383918850E-17, 1.000000000000000000, -8.716344404180429969E-17 ) ) ;
#53396=CARTESIAN_POINT ( 'NONE',  ( -7.769230765519999693, 1384.924143725650083, 218.9178332174689956 ) ) ;
#53399=CARTESIAN_POINT ( 'NONE',  ( -53.93365159477244219, 1379.703206717382272, 247.7545238405864438 ) ) ;
#53410=CARTESIAN_POINT ( 'NONE',  ( -59.34479193474174963, 1379.724027908502649, 264.5115275510683546 ) ) ;
#53433=CARTESIAN_POINT ( 'NONE',  ( -88.00931505469999649, 1389.318458636940022, 305.2260502545590271 ) ) ;
#53447=CARTESIAN_POINT ( 'NONE',  ( -105.0172044093909989, 1380.697436583209765, 308.0009267516720115 ) ) ;
#53474=CARTESIAN_POINT ( 'NONE',  ( -22.40689292945249989, 1384.854677225240039, 222.0968912656800001 ) ) ;
#53497=CARTESIAN_POINT ( 'NONE',  ( -105.6107621120000033, 1376.170439489020055, 306.5935537603590433 ) ) ;
#53533=CARTESIAN_POINT ( 'NONE',  ( -84.31096497809998880, 1379.600296256509864, 298.0935392271590558 ) ) ;
#53545=CARTESIAN_POINT ( 'NONE',  ( -17.51956951369999871, 1383.856177979750100, 219.7926916635590260 ) ) ;
#53551=CARTESIAN_POINT ( 'NONE',  ( -67.67522575920000349, 1379.745358396210122, 277.8355432199589927 ) ) ;
#53553=DIRECTION ( 'NONE',  ( 1.836970198721029688E-16, 1.000000000000000000, -1.262177448353620010E-31 ) ) ;
#53557=ORIENTED_EDGE ( 'NONE', *, *, #102340, .T. ) ;
#53560=CARTESIAN_POINT ( 'NONE',  ( -49.58302355399999328, 1384.869362640140025, 260.9124492692590138 ) ) ;
#53575=CARTESIAN_POINT ( 'NONE',  ( -5.931183514203220319, 1391.913060387289988, 215.1140006419229849 ) ) ;
#53613=CARTESIAN_POINT ( 'NONE',  ( -77.70051540026119596, 1383.778684295149787, 302.0161327210769855 ) ) ;
#53614=CARTESIAN_POINT ( 'NONE',  ( -109.4951920581290068, 1383.413356185199973, 311.1619299154190230 ) ) ;
#53621=CARTESIAN_POINT ( 'NONE',  ( -59.81489691519999496, 1382.332781621870026, 279.6089507563589791 ) ) ;
#53622=FACE_OUTER_BOUND ( 'NONE', #40110, .T. ) ;
#53675=EDGE_CURVE ( 'NONE', #110163, #56949, #55764, .T. ) ;
#53697=CARTESIAN_POINT ( 'NONE',  ( -11.64901520891459974, 1391.913060387140149, 208.7065094566399921 ) ) ;
#53709=CARTESIAN_POINT ( 'NONE',  ( -35.17158829440000289, 1389.591391915819941, 212.7234995045390065 ) ) ;
#53719=CARTESIAN_POINT ( 'NONE',  ( -8.148860876500000572, 1382.487756853370001, 218.5247792508289990 ) ) ;
#53727=DIRECTION ( 'NONE',  ( -1.000000000000000000, 0.000000000000000000, 0.000000000000000000 ) ) ;
#53741=CARTESIAN_POINT ( 'NONE',  ( -105.4624709189999834, 1391.255327103129957, 304.2078109453590287 ) ) ;
#53752=CARTESIAN_POINT ( 'NONE',  ( -28.88780438494880087, 1383.843457635159893, 226.6985655709949867 ) ) ;
#53757=ORIENTED_EDGE ( 'NONE', *, *, #35568, .T. ) ;
#53759=CARTESIAN_POINT ( 'NONE',  ( -3.078458307820000073, 1379.815171990729823, 214.0599463573090020 ) ) ;
#53765=CARTESIAN_POINT ( 'NONE',  ( -14.50876837679670039, 1379.873341110849879, 208.4861929993290062 ) ) ;
#53773=CARTESIAN_POINT ( 'NONE',  ( -93.78740748285459006, 1385.204112366519894, 294.4874550187400359 ) ) ;
#53786=CARTESIAN_POINT ( 'NONE',  ( -115.5939564047259296, 1379.913060387289988, 305.4204098037694735 ) ) ;
#53846=CARTESIAN_POINT ( 'NONE',  ( -108.5296511849999916, 1386.299881632349980, 297.3615022879590128 ) ) ;
#53849=CARTESIAN_POINT ( 'NONE',  ( -16.49045045709999968, 1379.616809272110004, 208.4493337902689802 ) ) ;
#53860=CARTESIAN_POINT ( 'NONE',  ( -72.87732534374360682, 1385.014528329849782, 298.0934590963260007 ) ) ;
#53871=CARTESIAN_POINT ( 'NONE',  ( -12.03882787510478991, 1391.913092977432598, 209.7302847345281407 ) ) ;
#53896=CARTESIAN_POINT ( 'NONE',  ( -7.542953837611409362, 1384.718779688529821, 219.0831055481480121 ) ) ;
#53909=CARTESIAN_POINT ( 'NONE',  ( -107.6419135281290096, 1384.586188811220154, 311.2437287102239907 ) ) ;
#53910=CARTESIAN_POINT ( 'NONE',  ( -30.87778110501150408, 1384.970453077349930, 206.0489399718400136 ) ) ;
#53923=CARTESIAN_POINT ( 'NONE',  ( -106.8632684893990046, 1391.913060387289988, 306.3664403480210012 ) ) ;
#53927=CARTESIAN_POINT ( 'NONE',  ( -11.25209998319999904, 1378.783920428300007, 203.9551270864290302 ) ) ;
#53939=CARTESIAN_POINT ( 'NONE',  ( -60.13904085021329848, 1379.723828619409915, 265.9902606016499931 ) ) ;
#53945=CARTESIAN_POINT ( 'NONE',  ( -109.4841057800000073, 1384.929175104179876, 311.2840925992589973 ) ) ;
#53971=CARTESIAN_POINT ( 'NONE',  ( -13.19353006659999927, 1379.589451595169976, 208.3384645246609921 ) ) ;
#53972=CARTESIAN_POINT ( 'NONE',  ( -28.30903825226335613, 1379.623442209230689, 212.7910287074695646 ) ) ;
#53983=CARTESIAN_POINT ( 'NONE',  ( -61.23078504541961564, 1379.729633516930562, 268.1594380621943969 ) ) ;
#53989=DIRECTION ( 'NONE',  ( -0.9998780035959983215, 8.712314624148121749E-33, 0.01561979272847786350 ) ) ;
#54003=CARTESIAN_POINT ( 'NONE',  ( -92.33864210410000339, 1388.280693857359893, 295.1786243173589810 ) ) ;
#54016=CARTESIAN_POINT ( 'NONE',  ( -104.4920613472269935, 1380.551098421130064, 307.6454722610029648 ) ) ;
#54041=CARTESIAN_POINT ( 'NONE',  ( -23.12467871438520461, 1384.852336965640006, 222.5014426972579997 ) ) ;
#54063=CARTESIAN_POINT ( 'NONE',  ( -68.69232588285649399, 1379.746858116560134, 280.5557452193770587 ) ) ;
#54073=CARTESIAN_POINT ( 'NONE',  ( -7.870791249149999835, 1383.842518133449857, 218.8008077258490118 ) ) ;
#54089=ORIENTED_EDGE ( 'NONE', *, *, #24203, .T. ) ;
#54096=CARTESIAN_POINT ( 'NONE',  ( -71.62432532130000595, 1379.712643070030026, 285.2199721836589674 ) ) ;
#54112=CARTESIAN_POINT ( 'NONE',  ( -67.89413382450000256, 1379.746388715500188, 278.3036684585590024 ) ) ;
#54120=CARTESIAN_POINT ( 'NONE',  ( -67.03985474800001043, 1384.791062983040092, 292.1873690184589805 ) ) ;
#54122=CARTESIAN_POINT ( 'NONE',  ( -27.55265326522230040, 1385.244708163680116, 225.6838886635030121 ) ) ;
#54127=CARTESIAN_POINT ( 'NONE',  ( 10.22326110114815201, 1375.913060387289988, 204.3929701860967896 ) ) ;
#54166=CARTESIAN_POINT ( 'NONE',  ( -90.49287011937269654, 1383.770007548130025, 308.6794120424070229 ) ) ;
#54167=CARTESIAN_POINT ( 'NONE',  ( -108.8617172214759989, 1383.656556793380105, 311.0417015030730568 ) ) ;
#54172=CARTESIAN_POINT ( 'NONE',  ( -94.23475628420000305, 1381.920488750169852, 295.6479955697590185 ) ) ;
#54182=CARTESIAN_POINT ( 'NONE',  ( -109.3504515160000068, 1384.878600923439990, 297.1334136532590264 ) ) ;
#54189=CARTESIAN_POINT ( 'NONE',  ( -107.2951360021110645, 1379.629536132615613, 309.1752404442335660 ) ) ;
#54254=CARTESIAN_POINT ( 'NONE',  ( -46.09131934240000561, 1385.005100670120100, 219.0267588369590044 ) ) ;
#54255=DIRECTION ( 'NONE',  ( 1.000000000000000000, 0.000000000000000000, 0.000000000000000000 ) ) ;
#54261=CARTESIAN_POINT ( 'NONE',  ( -9.902446976249999366, 1380.336055740079928, 216.6871926996190041 ) ) ;
#54279=CARTESIAN_POINT ( 'NONE',  ( -110.0482600249999905, 1385.373320011429996, 296.9711117020590336 ) ) ;
#54292=CARTESIAN_POINT ( 'NONE',  ( -17.57918762556300152, 1383.856065982129849, 219.9043076063699971 ) ) ;
#54300=CARTESIAN_POINT ( 'NONE',  ( -9.251598888397834841, 1388.591673295162082, 200.8599406664134506 ) ) ;
#54306=CARTESIAN_POINT ( 'NONE',  ( -10.06453687412319908, 1387.658551857550037, 217.5792455951880129 ) ) ;
#54316=CARTESIAN_POINT ( 'NONE',  ( -103.4461152369070049, 1385.229357875270125, 296.7794697699490030 ) ) ;
#54318=CARTESIAN_POINT ( 'NONE',  ( -25.99322061230196113, 1379.720623260343245, 211.7359130857557545 ) ) ;
#54336=CARTESIAN_POINT ( 'NONE',  ( -8.861482052969998691, 1384.950957082100103, 218.6848127019790127 ) ) ;
#54342=CARTESIAN_POINT ( 'NONE',  ( -103.5847285859999971, 1379.882004272549921, 303.6035322816589996 ) ) ;
#54361=CARTESIAN_POINT ( 'NONE',  ( -22.99522306489999579, 1384.540050732020063, 202.4077213122689898 ) ) ;
#54371=ORIENTED_EDGE ( 'NONE', *, *, #81578, .T. ) ;
#54396=CARTESIAN_POINT ( 'NONE',  ( -26.04447212934309164, 1379.718901743828837, 215.2627710545450839 ) ) ;
#54403=CARTESIAN_POINT ( 'NONE',  ( -55.04432150766159992, 1385.092390689839931, 271.8936798544510225 ) ) ;
#54438=CARTESIAN_POINT ( 'NONE',  ( -7.582807648377508869, 1384.152347710639788, 219.0341480461830201 ) ) ;
#54441=ORIENTED_EDGE ( 'NONE', *, *, #85625, .T. ) ;
#54451=CARTESIAN_POINT ( 'NONE',  ( -84.08298741828620848, 1384.630359715449913, 306.2334057474649853 ) ) ;
#54452=CARTESIAN_POINT ( 'NONE',  ( -43.92410954080200014, 1385.000048749679991, 217.0325689943980194 ) ) ;
#54466=CARTESIAN_POINT ( 'NONE',  ( -106.5689870562550112, 1391.913060387289988, 305.4639128772769823 ) ) ;
#54470=CARTESIAN_POINT ( 'NONE',  ( -10.66583685980000062, 1379.443864687059886, 202.8590315047190131 ) ) ;
#54485=CARTESIAN_POINT ( 'NONE',  ( -67.65809801332019902, 1379.745325822590075, 278.9855928749340137 ) ) ;
#54491=CARTESIAN_POINT ( 'NONE',  ( -105.3072927039999911, 1379.015832552830034, 304.0377861886589699 ) ) ;
#54492=CARTESIAN_POINT ( 'NONE',  ( -109.4847723999999971, 1384.941599254929997, 311.2840177552590717 ) ) ;
#54508=ORIENTED_EDGE ( 'NONE', *, *, #97224, .T. ) ;
#54518=CARTESIAN_POINT ( 'NONE',  ( -68.02398329241702868, 1379.746453776986527, 278.4801873761143725 ) ) ;
#54520=EDGE_CURVE ( 'NONE', #108323, #55409, #46167, .T. ) ;
#54531=CARTESIAN_POINT ( 'NONE',  ( -22.14212065537508778, 1379.609184651877058, 213.9947383123216014 ) ) ;
#54549=CARTESIAN_POINT ( 'NONE',  ( -109.9987473150000028, 1388.279950299490110, 298.2983701788589883 ) ) ;
#54561=CARTESIAN_POINT ( 'NONE',  ( -104.0127261669699976, 1380.213078394089962, 306.6829892870579783 ) ) ;
#54584=CARTESIAN_POINT ( 'NONE',  ( -38.78333047650129828, 1384.792994315660053, 240.0455148828049801 ) ) ;
#54601=CARTESIAN_POINT ( 'NONE',  ( -13.07882001760000179, 1380.090973434839952, 209.8378495415080067 ) ) ;
#54603=CARTESIAN_POINT ( 'NONE',  ( -109.9877442644620089, 1384.809409080889964, 311.4546249735340098 ) ) ;
#54608=CARTESIAN_POINT ( 'NONE',  ( -93.86205675402460713, 1379.086295911220077, 304.7318000099389792 ) ) ;
#54610=CARTESIAN_POINT ( 'NONE',  ( -16.70762542998109978, 1379.711292899869932, 211.9326756087270098 ) ) ;
#54618=CARTESIAN_POINT ( 'NONE',  ( -105.0196309849999921, 1390.463858102760014, 304.1900860135590392 ) ) ;
#54628=ORIENTED_EDGE ( 'NONE', *, *, #50782, .F. ) ;
#54641=CARTESIAN_POINT ( 'NONE',  ( -72.92954128540000625, 1379.405105560169886, 284.3347022608589896 ) ) ;
#54649=CARTESIAN_POINT ( 'NONE',  ( -109.9987473190000031, 1384.904025801279886, 297.1695833602590255 ) ) ;
#54660=CARTESIAN_POINT ( 'NONE',  ( -67.64911565900000312, 1379.747065449480033, 277.8485390883590185 ) ) ;
#54669=( BOUNDED_CURVE ( )  B_SPLINE_CURVE ( 3, ( #7047, #14330, #65870, #32251 ),
 .UNSPECIFIED., .F., .F. ) 
 B_SPLINE_CURVE_WITH_KNOTS ( ( 4, 4 ),
 ( 6.239037601373940589, 6.281338949178555175 ),
 .UNSPECIFIED. ) 
 CURVE ( )  GEOMETRIC_REPRESENTATION_ITEM ( )  RATIONAL_B_SPLINE_CURVE ( ( 1.000000000000000000, 0.9998508885567132243, 0.9998508885567132243, 1.000000000000000000 ) ) 
 REPRESENTATION_ITEM ( '' )  );
#54672=CARTESIAN_POINT ( 'NONE',  ( -28.75295618251070096, 1385.239309608959957, 226.7833509653069939 ) ) ;
#54690=PRODUCT_DEFINITION_CONTEXT ( 'detailed design', #104952, 'design' ) ;
#54702=CARTESIAN_POINT ( 'NONE',  ( -105.6234263439999950, 1377.955790496569762, 303.2972783946590312 ) ) ;
#54711=DIRECTION ( 'NONE',  ( 1.836970198721029688E-16, 1.000000000000000000, 0.000000000000000000 ) ) ;
#54715=CARTESIAN_POINT ( 'NONE',  ( -86.90971335866299796, 1383.772295304499949, 307.3582144528240292 ) ) ;
#54721=CARTESIAN_POINT ( 'NONE',  ( -98.86569637809999733, 1383.405061561229786, 296.2692300583589713 ) ) ;
#54792=CARTESIAN_POINT ( 'NONE',  ( -9.122186852882011365, 1384.516432268700100, 199.9701712313529924 ) ) ;
#54816=EDGE_CURVE ( 'NONE', #107758, #67300, #32897, .T. ) ;
#54821=CARTESIAN_POINT ( 'NONE',  ( -109.5386125330000056, 1385.082371152899896, 297.1260739345589741 ) ) ;
#54833=CARTESIAN_POINT ( 'NONE',  ( -22.35747404037720187, 1383.851046513379970, 221.8738471675100072 ) ) ;
#54836=EDGE_CURVE ( 'NONE', #89045, #52311, #16810, .T. ) ;
#54842=CARTESIAN_POINT ( 'NONE',  ( -10.25244544798204949, 1389.903864462993852, 202.2017625968174741 ) ) ;
#54849=CARTESIAN_POINT ( 'NONE',  ( -11.78173983558050075, 1389.131401572190043, 215.6488607812810017 ) ) ;
#54852=EDGE_CURVE ( 'NONE', #91726, #70768, #46239, .T. ) ;
#54858=CARTESIAN_POINT ( 'NONE',  ( -107.6301326754700085, 1385.239087081850130, 297.0876625113839395 ) ) ;
#54861=AXIS2_PLACEMENT_3D ( 'NONE', #70692, #1817, #45479 ) ;
#54865=CARTESIAN_POINT ( 'NONE',  ( -109.1656546792999904, 1384.956445601399992, 297.1328575267269798 ) ) ;
#54882=CARTESIAN_POINT ( 'NONE',  ( -108.7852627620000021, 1383.811234508949838, 297.2705451043590301 ) ) ;
#54910=EDGE_LOOP ( 'NONE', ( #88712, #60714, #7718, #63279, #72934, #85047 ) ) ;
#54923=CIRCLE ( 'NONE', #35237, 6.842541678089994583 ) ;
#54932=CARTESIAN_POINT ( 'NONE',  ( -107.0144454107080065, 1391.913060387289988, 307.4418187106899722 ) ) ;
#54933=CARTESIAN_POINT ( 'NONE',  ( -68.39881485713311804, 1379.747709036739025, 279.9507912017972444 ) ) ;
#54941=CARTESIAN_POINT ( 'NONE',  ( -84.45939852480390186, 1384.982670101519943, 306.4352233390739570 ) ) ;
#54944=CARTESIAN_POINT ( 'NONE',  ( -8.491041205600000197, 1384.938468836829998, 199.8127951144290080 ) ) ;
#54946=CARTESIAN_POINT ( 'NONE',  ( -113.4000000000000057, 1378.913060387289988, 304.2218459572590064 ) ) ;
#54979=CARTESIAN_POINT ( 'NONE',  ( -7.734417504676620148, 1383.405642709869880, 218.8913851597439759 ) ) ;
#54994=ADVANCED_FACE ( 'NONE', ( #34549 ), #48647, .T. ) ;
#54996=CARTESIAN_POINT ( 'NONE',  ( -91.63069530043399880, 1384.616216363609965, 309.2058898380819869 ) ) ;
#54997=CARTESIAN_POINT ( 'NONE',  ( -40.96489448099129760, 1384.992258638779958, 213.8259286978779983 ) ) ;
#55020=CARTESIAN_POINT ( 'NONE',  ( -5.013263847643504967, 1375.354125225655480, 203.5257469810366899 ) ) ;
#55026=CARTESIAN_POINT ( 'NONE',  ( -68.17361118975399847, 1379.746536065940063, 279.6965955867630100 ) ) ;
#55056=CARTESIAN_POINT ( 'NONE',  ( -12.31987546760000107, 1378.182896874270000, 209.4394672709660199 ) ) ;
#55057=CARTESIAN_POINT ( 'NONE',  ( -67.87117022811392530, 1379.746131644044226, 278.1675811678725267 ) ) ;
#55061=CARTESIAN_POINT ( 'NONE',  ( -59.16060917409809861, 1384.667876448820152, 242.2189909261509797 ) ) ;
#55068=ORIENTED_EDGE ( 'NONE', *, *, #94509, .T. ) ;
#55081=CARTESIAN_POINT ( 'NONE',  ( -103.5806803890000083, 1389.940350142260058, 304.1776731731589507 ) ) ;
#55090=CARTESIAN_POINT ( 'NONE',  ( -109.9987472819999965, 1388.002180556429948, 310.4334137642590008 ) ) ;
#55105=CARTESIAN_POINT ( 'NONE',  ( -106.2761447790000062, 1378.746492803760020, 307.5519750587589556 ) ) ;
#55134=CARTESIAN_POINT ( 'NONE',  ( -30.71459829396640018, 1384.825797510230132, 228.8220148752180023 ) ) ;
#55137=CARTESIAN_POINT ( 'NONE',  ( -105.0711645279999971, 1379.235653477059941, 303.4121855584589866 ) ) ;
#55143=ORIENTED_EDGE ( 'NONE', *, *, #43130, .T. ) ;
#55157=CARTESIAN_POINT ( 'NONE',  ( -77.18529333353220068, 1379.656469662269956, 292.4663616554850023 ) ) ;
#55159=CARTESIAN_POINT ( 'NONE',  ( -19.18445155381639822, 1379.602224620720108, 212.8959267389929835 ) ) ;
#55160=ORIENTED_EDGE ( 'NONE', *, *, #7895, .T. ) ;
#55166=CARTESIAN_POINT ( 'NONE',  ( -8.856807571699999215, 1384.768264595860046, 218.6834643707789780 ) ) ;
#55180=AXIS2_PLACEMENT_3D ( 'NONE', #6307, #57833, #137 ) ;
#55186=CARTESIAN_POINT ( 'NONE',  ( -13.85438721787440031, 1379.977881741410101, 208.5176583983199805 ) ) ;
#55187=CIRCLE ( 'NONE', #33627, 2.500000000000002220 ) ;
#55190=CARTESIAN_POINT ( 'NONE',  ( -59.28197579180000076, 1375.203196137529858, 258.5658342392590043 ) ) ;
#55199=CARTESIAN_POINT ( 'NONE',  ( -113.4000000000000057, 1391.913060387289988, 304.2218459572590064 ) ) ;
#55201=CARTESIAN_POINT ( 'NONE',  ( -3.078458293520000222, 1384.558481699660206, 218.5731838834990128 ) ) ;
#55205=CARTESIAN_POINT ( 'NONE',  ( -65.84461506920000318, 1379.745083454579799, 274.2711187272589655 ) ) ;
#55213=CARTESIAN_POINT ( 'NONE',  ( -96.24084593199999915, 1384.955172021569979, 310.5859090792589541 ) ) ;
#55216=CARTESIAN_POINT ( 'NONE',  ( -22.41728899266079722, 1385.266610229700063, 222.0786659537150172 ) ) ;
#55217=DIRECTION ( 'NONE',  ( -1.836970198721029688E-16, -1.000000000000000000, 0.000000000000000000 ) ) ;
#55245=ORIENTED_EDGE ( 'NONE', *, *, #4296, .T. ) ;
#55263=CARTESIAN_POINT ( 'NONE',  ( -109.6087247409329848, 1383.177901426799963, 311.2147930400129781 ) ) ;
#55267=ORIENTED_EDGE ( 'NONE', *, *, #31835, .T. ) ;
#55268=CARTESIAN_POINT ( 'NONE',  ( -103.6840079290000034, 1381.964784448540058, 297.7019806198590004 ) ) ;
#55274=CARTESIAN_POINT ( 'NONE',  ( -109.8948246550000079, 1384.907839483040107, 297.0284603415590254 ) ) ;
#55302=ORIENTED_EDGE ( 'NONE', *, *, #90209, .T. ) ;
#55312=B_SPLINE_SURFACE_WITH_KNOTS ( 'NONE', 5, 3, ( 
 ( #75976, #93861, #15494, #33401 ),
 ( #17129, #51319, #66508, #101704 ),
 ( #59199, #16580, #92223, #68161 ),
 ( #85455, #65948, #40720, #100074 ),
 ( #74892, #32327, #53003, #77635 ),
 ( #104487, #102805, #26101, #51891 ),
 ( #86580, #9872, #28336, #27780 ),
 ( #26662, #18255, #44596, #34521 ),
 ( #52451, #68700, #8753, #44039 ),
 ( #78178, #60863, #45160, #70931 ),
 ( #78740, #79300, #87136, #69253 ),
 ( #95535, #103360, #61970, #69816 ),
 ( #94987, #2055, #1489, #62529 ),
 ( #35072, #35620, #36736, #61412 ),
 ( #103933, #19359, #70372, #2611 ),
 ( #105047, #53560, #86028, #77094 ),
 ( #27232, #87707, #96651, #947 ),
 ( #60290, #9329, #94409, #18808 ),
 ( #19920, #96084, #10426, #36188 ),
 ( #10986, #54120, #17685, #42936 ),
 ( #404, #43492, #89887, #46816 ),
 ( #88248, #29975, #45716, #64167 ),
 ( #97740, #98285, #80945, #4244 ),
 ( #63088, #4775, #37844, #63624 ),
 ( #80400, #21011, #21562, #55772 ),
 ( #107797, #71487, #106684, #55213 ),
 ( #38379, #72031, #3164, #105608 ),
 ( #81472, #82030, #47894, #98840 ),
 ( #12079, #106147, #89342, #5334 ),
 ( #28892, #31082, #97186, #72554 ) ),
 .UNSPECIFIED., .F., .F., .F.,
 ( 6, 3, 3, 3, 3, 3, 3, 3, 3, 6 ),
 ( 4, 4 ),
 ( 0.000000000000000000, 15.39383910899999997, 27.58084801740000103, 41.39509552349999666, 65.53909258059999843, 90.91108773649999364, 117.6367619669999982, 132.4493970709999928, 144.8160795070000120, 161.8240513320000105 ),
 ( 68.11858234059999972, 68.97209088700000734 ),
 .UNSPECIFIED. ) ;
#55318=CARTESIAN_POINT ( 'NONE',  ( -16.95855574732879845, 1384.526604847959788, 200.9892168643340256 ) ) ;
#55324=VERTEX_POINT ( 'NONE', #100777 ) ;
#55338=ORIENTED_EDGE ( 'NONE', *, *, #74340, .T. ) ;
#55369=CARTESIAN_POINT ( 'NONE',  ( -109.3535611529999869, 1385.012954933069977, 297.1394016240590759 ) ) ;
#55379=CARTESIAN_POINT ( 'NONE',  ( -17.93185251124669932, 1383.855712211560103, 220.0128206254979943 ) ) ;
#55389=CARTESIAN_POINT ( 'NONE',  ( -8.753528060440000758, 1383.864184473070054, 218.4105340633189769 ) ) ;
#55395=CARTESIAN_POINT ( 'NONE',  ( -10.04612998989999895, 1389.631361075330005, 216.4686791083889830 ) ) ;
#55403=CARTESIAN_POINT ( 'NONE',  ( -7.966091435999130610, 1384.906085766829847, 199.4893022481589924 ) ) ;
#55404=CARTESIAN_POINT ( 'NONE',  ( -99.99640236783429259, 1385.220859795530032, 296.2804087198049956 ) ) ;
#55406=CARTESIAN_POINT ( 'NONE',  ( -67.25967724030000738, 1379.748837366600128, 277.1187736907589851 ) ) ;
#55409=VERTEX_POINT ( 'NONE', #65009 ) ;
#55416=CARTESIAN_POINT ( 'NONE',  ( -109.4004660420000050, 1385.924158871910095, 311.2011470452590061 ) ) ;
#55426=CARTESIAN_POINT ( 'NONE',  ( -8.600120389129999765, 1385.305366698150010, 218.6461194263490029 ) ) ;
#55480=CARTESIAN_POINT ( 'NONE',  ( -119.8718586775642478, 1384.926148861439970, 299.5197653927720580 ) ) ;
#55484=CARTESIAN_POINT ( 'NONE',  ( -67.00076415386901374, 1379.747503662026475, 277.9341329112440349 ) ) ;
#55491=CARTESIAN_POINT ( 'NONE',  ( -94.45576590239029713, 1384.959238494370084, 309.9322998303119903 ) ) ;
#55492=CARTESIAN_POINT ( 'NONE',  ( -9.582177284329999267, 1388.523135097040040, 201.1746843562989966 ) ) ;
#55539=CARTESIAN_POINT ( 'NONE',  ( -102.5927908494250005, 1384.595964578270241, 311.0546370185200544 ) ) ;
#55540=CARTESIAN_POINT ( 'NONE',  ( -32.53064427015559801, 1384.973673283899871, 207.0391211637609956 ) ) ;
#55560=CARTESIAN_POINT ( 'NONE',  ( -12.88669223129999963, 1379.421126886189995, 207.0600552223190221 ) ) ;
#55573=CARTESIAN_POINT ( 'NONE',  ( -68.04880748148440262, 1379.746211451220006, 279.5452075350660266 ) ) ;
#55607=CARTESIAN_POINT ( 'NONE',  ( -66.61252592013686069, 1379.743324869505159, 275.6254950077977242 ) ) ;
#55612=CARTESIAN_POINT ( 'NONE',  ( -60.11345111107429773, 1384.673691186940005, 244.2542627049520263 ) ) ;
#55653=CARTESIAN_POINT ( 'NONE',  ( -12.47575420717869932, 1379.153280478169791, 210.8825727293119883 ) ) ;
#55668=CARTESIAN_POINT ( 'NONE',  ( -105.4624709189999834, 1391.255327103129957, 304.2078109453590287 ) ) ;
#55680=CARTESIAN_POINT ( 'NONE',  ( -37.03571219771700385, 1384.800574037690012, 237.2200498466380054 ) ) ;
#55705=CARTESIAN_POINT ( 'NONE',  ( -86.17839381677090671, 1377.185129373109930, 302.3619043579220147 ) ) ;
#55706=TOROIDAL_SURFACE ( 'NONE', #48582, 8.013264357029999729, 0.5000000000000000000 ) ;
#55716=CARTESIAN_POINT ( 'NONE',  ( -113.3764034147090882, 1389.413060387289988, 303.2221243954415968 ) ) ;
#55718=CARTESIAN_POINT ( 'NONE',  ( -7.767750813309999280, 1384.590689248749868, 218.9085672489989918 ) ) ;
#55721=EDGE_CURVE ( 'NONE', #13675, #49086, #110722, .T. ) ;
#55725=DIRECTION ( 'NONE',  ( 1.836970198721029688E-16, 1.000000000000000000, 0.000000000000000000 ) ) ;
#55738=CARTESIAN_POINT ( 'NONE',  ( -13.07885320302169951, 1380.091007900090062, 209.8378948098500132 ) ) ;
#55744=CARTESIAN_POINT ( 'NONE',  ( -50.85477211639999950, 1380.010081756269983, 242.1550097551590000 ) ) ;
#55753=ORIENTED_EDGE ( 'NONE', *, *, #106886, .T. ) ;
#55755=CYLINDRICAL_SURFACE ( 'NONE', #31497, 0.4999999999999449329 ) ;
#55757=CARTESIAN_POINT ( 'NONE',  ( -1.364749936328269942E-15, 1384.563555726449977, 218.6218459572590120 ) ) ;
#55763=CARTESIAN_POINT ( 'NONE',  ( -59.96754922390000075, 1379.749011644449865, 261.8279529299589967 ) ) ;
#55764=B_SPLINE_CURVE_WITH_KNOTS ( 'NONE', 3,
 ( #36318, #98292, #21566, #95683 ),
 .UNSPECIFIED., .F., .F.,
 ( 4, 4 ),
 ( 55.36930458839999858, 55.41785034089999584 ),
 .UNSPECIFIED. ) ;
#55772=CARTESIAN_POINT ( 'NONE',  ( -89.65022158889999560, 1384.970293222339933, 308.7482827413589348 ) ) ;
#55774=CARTESIAN_POINT ( 'NONE',  ( -28.44980152130050044, 1385.240686751639942, 226.4935510166359904 ) ) ;
#55798=CARTESIAN_POINT ( 'NONE',  ( -105.1057160200000027, 1389.703205635770018, 300.9611973728590328 ) ) ;
#55800=CARTESIAN_POINT ( 'NONE',  ( -106.4020475519999991, 1391.913060387289988, 304.2007934394590620 ) ) ;
#55804=CARTESIAN_POINT ( 'NONE',  ( -104.1991720430000186, 1379.825027202220099, 304.0120836943589779 ) ) ;
#55819=CARTESIAN_POINT ( 'NONE',  ( -109.9987472859999968, 1381.043808635240111, 309.4164141372589825 ) ) ;
#55824=CARTESIAN_POINT ( 'NONE',  ( -109.7178227269999979, 1384.906453685299994, 297.0861895859590049 ) ) ;
#55825=CARTESIAN_POINT ( 'NONE',  ( -8.860592775618536976, 1381.856380555122996, 200.4166704413667333 ) ) ;
#55850=EDGE_CURVE ( 'NONE', #61100, #48273, #68206, .T. ) ;
#55873=CARTESIAN_POINT ( 'NONE',  ( -10.32431769148769973, 1384.511448824909849, 200.0654769700809936 ) ) ;
#55920=CARTESIAN_POINT ( 'NONE',  ( -109.1656546789999993, 1384.956445596120147, 297.1328575266589951 ) ) ;
#55929=CARTESIAN_POINT ( 'NONE',  ( -38.95288734898669958, 1383.829750491509913, 239.9923225223510030 ) ) ;
#55938=CARTESIAN_POINT ( 'NONE',  ( -25.90756897309999829, 1384.546519395709765, 203.4684288897289832 ) ) ;
#55944=CARTESIAN_POINT ( 'NONE',  ( -9.285067551966019295, 1387.122678197030154, 218.0550403871500009 ) ) ;
#55965=CARTESIAN_POINT ( 'NONE',  ( -109.5110906019999959, 1386.650732619270002, 311.1668118922589770 ) ) ;
#55974=CARTESIAN_POINT ( 'NONE',  ( -7.556639502920000417, 1385.398637304449949, 219.0631512379790138 ) ) ;
#55979=EDGE_CURVE ( 'NONE', #103332, #62022, #102317, .T. ) ;
#56000=CARTESIAN_POINT ( 'NONE',  ( -107.2899050854710055, 1379.886892357829993, 309.1794776302379546 ) ) ;
#56020=CARTESIAN_POINT ( 'NONE',  ( -109.0982299788821024, 1382.066543485014108, 297.5654259004551818 ) ) ;
#56024=CARTESIAN_POINT ( 'NONE',  ( -107.2902884299589914, 1391.913060387289988, 307.3027227297359900 ) ) ;
#56031=CARTESIAN_POINT ( 'NONE',  ( -81.22482676457471484, 1384.990768542609885, 304.6421476864239253 ) ) ;
#56032=CARTESIAN_POINT ( 'NONE',  ( -9.721596386979999949, 1387.218309458520253, 200.7551491867290281 ) ) ;
#56074=CARTESIAN_POINT ( 'NONE',  ( -13.64835502960000113, 1380.295393291809887, 210.2814589097189923 ) ) ;
#56075=CARTESIAN_POINT ( 'NONE',  ( -95.83152833198130338, 1384.608534833750127, 310.2052327687620163 ) ) ;
#56076=B_SPLINE_SURFACE_WITH_KNOTS ( 'NONE', 5, 5, ( 
 ( #94781, #18601, #19150, #102064, #25901, #85262 ),
 ( #52253, #1289, #59539, #104292, #60099, #35429 ),
 ( #53357, #26462, #69616, #43292, #94215, #77440 ),
 ( #86379, #44962, #60657, #17490, #79110, #18059 ),
 ( #741, #9665, #86932, #8559, #34872, #2417 ),
 ( #103737, #67954, #42731, #27038, #61226, #76890 ),
 ( #52801, #51688, #27579, #85828, #10223, #44401 ),
 ( #78543, #35992, #16934, #61764, #51136, #96447 ),
 ( #63967, #98082, #29238, #62896, #97545, #46062 ),
 ( #54470, #81275, #107040, #19726, #38725, #80747 ),
 ( #53927, #98631, #37082, #97006, #38182, #105399 ),
 ( #4056, #89685, #72362, #80195, #29779, #79661 ),
 ( #20269, #28692, #88062, #88608, #106494, #47697 ),
 ( #11347, #63427, #21353, #55560, #12967, #47150 ),
 ( #45519, #2965, #28131, #89141, #11890, #71286 ) ),
 .UNSPECIFIED., .F., .F., .F.,
 ( 6, 3, 3, 3, 6 ),
 ( 6, 6 ),
 ( 7.411273261979999916, 10.46453992930000076, 15.62038767109999959, 19.62991602479999997, 26.81730491820000140 ),
 ( 0.000000000000000000, 2.000000000000000000 ),
 .UNSPECIFIED. ) ;
#56077=CARTESIAN_POINT ( 'NONE',  ( -50.37285252689139980, 1385.020400592789883, 225.8367497718959953 ) ) ;
#56086=CARTESIAN_POINT ( 'NONE',  ( -109.8257969779999854, 1384.899434086499923, 311.3808307492589620 ) ) ;
#56106=CARTESIAN_POINT ( 'NONE',  ( -67.33396345445230224, 1379.744479302740046, 278.5401087013319739 ) ) ;
#56117=CARTESIAN_POINT ( 'NONE',  ( -107.1397530847460047, 1378.913060387289988, 307.3765361525499316 ) ) ;
#56133=CARTESIAN_POINT ( 'NONE',  ( -62.99661746870935275, 1379.733886384323114, 268.0375848082739481 ) ) ;
#56137=CARTESIAN_POINT ( 'NONE',  ( -86.19296323747759914, 1384.823008793549889, 289.8026865565949493 ) ) ;
#56167=CARTESIAN_POINT ( 'NONE',  ( -8.847782810029999112, 1384.881200155019997, 199.9249090898990175 ) ) ;
#56178=B_SPLINE_CURVE_WITH_KNOTS ( 'NONE', 3,
 ( #76546, #8779, #92796, #68185, #59767, #100632, #23918, #93888, #23379, #58113, #109607, #50270, #92246 ),
 .UNSPECIFIED., .F., .F.,
 ( 4, 3, 3, 3, 4 ),
 ( 0.9325643982709880264, 0.9611848085218949178, 1.006251133202479942, 1.031824629410019956, 1.051317457883059969 ),
 .UNSPECIFIED. ) ;
#56195=EDGE_CURVE ( 'NONE', #84984, #110163, #87005, .T. ) ;
#56207=CARTESIAN_POINT ( 'NONE',  ( -27.53652019058529987, 1384.837329755710016, 225.6946210897860112 ) ) ;
#56212=CARTESIAN_POINT ( 'NONE',  ( -105.1701305670000011, 1379.114535495230029, 304.0350737403589960 ) ) ;
#56234=CARTESIAN_POINT ( 'NONE',  ( -55.69680533319999682, 1376.605089213109977, 260.2049226822590526 ) ) ;
#56246=CARTESIAN_POINT ( 'NONE',  ( -7.991901621120000243, 1383.415651595959844, 218.6863616538790041 ) ) ;
#56263=CARTESIAN_POINT ( 'NONE',  ( -108.7866006633440179, 1388.050027694506070, 310.6579109707056432 ) ) ;
#56270=CARTESIAN_POINT ( 'NONE',  ( -36.43074434249999172, 1375.172836988449944, 219.9641098163590129 ) ) ;
#56284=CARTESIAN_POINT ( 'NONE',  ( -47.43982414079999899, 1384.124103258099922, 256.2477275100589509 ) ) ;
#56290=CARTESIAN_POINT ( 'NONE',  ( -62.81000518919999109, 1379.749407722699971, 268.0377337381589768 ) ) ;
#56300=CARTESIAN_POINT ( 'NONE',  ( -22.66379694789999988, 1390.973251371299966, 211.6870299638790129 ) ) ;
#56302=CARTESIAN_POINT ( 'NONE',  ( -33.87156971251739890, 1385.214877942069961, 232.6218372687270062 ) ) ;
#56330=CARTESIAN_POINT ( 'NONE',  ( -103.8055019550000111, 1389.814814112089834, 301.7479020532589971 ) ) ;
#56356=CARTESIAN_POINT ( 'NONE',  ( -96.92558477839999398, 1380.099996794379877, 306.8584593190589658 ) ) ;
#56379=ORIENTED_EDGE ( 'NONE', *, *, #87675, .T. ) ;
#56420=CARTESIAN_POINT ( 'NONE',  ( -9.171139168049998958, 1384.273561242960113, 200.0050165398689899 ) ) ;
#56425=CARTESIAN_POINT ( 'NONE',  ( -68.78237022239999021, 1379.747949065490047, 280.2620412852589880 ) ) ;
#56442=CARTESIAN_POINT ( 'NONE',  ( -14.07423802120690759, 1379.606304211416273, 211.7193776285950833 ) ) ;
#56457=CARTESIAN_POINT ( 'NONE',  ( -105.3716458700000089, 1379.306619424940209, 302.1984682570590053 ) ) ;
#56460=B_SPLINE_SURFACE_WITH_KNOTS ( 'NONE', 5, 5, ( 
 ( #6648, #47019, #4988, #109128, #91203, #4459, #74980, #21207, #81144 ),
 ( #13371, #83349, #72766, #30743, #23441, #106893, #32409, #49223, #30181 ),
 ( #21764, #15025, #57635, #22314, #12839, #81682, #82252, #31294, #31847 ),
 ( #66590, #65478, #99587, #64373, #55416, #39703, #89550, #98496, #39132 ),
 ( #14484, #55965, #90088, #47560, #73311, #107447, #82800, #64924, #22870 ),
 ( #13927, #99037, #56517, #90644, #73869, #48114, #107997, #57079, #6094 ),
 ( #48677, #74431, #66033, #108557, #100156, #60382, #75532, #16130, #23977 ),
 ( #9413, #94502, #8842, #7209, #17219, #33484, #50868, #93952, #34609 ),
 ( #58171, #101231, #85546, #67686, #17775, #84997, #100693, #50336, #24531 ),
 ( #77183, #101794, #102356, #76068, #110211, #2563, #93405, #25084, #51977 ),
 ( #36686, #59287, #8292, #15570, #76614, #7749, #43025, #110766, #86119 ),
 ( #34056, #43575, #68248, #41365, #16670, #42455, #51414, #68795, #25639 ),
 ( #59831, #58719, #486, #92854, #92300, #102895, #26194, #84462, #77724 ),
 ( #49772, #83903, #41914, #109667, #32942, #67132, #107192, #106634, #29923 ),
 ( #88199, #80896, #22049, #3665, #54618, #4728, #47843, #30481, #38872 ) ),
 .UNSPECIFIED., .F., .F., .F.,
 ( 6, 3, 3, 3, 6 ),
 ( 6, 3, 6 ),
 ( 7.927024885419999833, 11.42826484960000144, 13.38558606099999970, 18.01519608889999802, 29.56630841140000143 ),
 ( 0.000000000000000000, 1.000000000000000000, 2.000000000000000000 ),
 .UNSPECIFIED. ) ;
#56465=EDGE_CURVE ( 'NONE', #33840, #42195, #103621, .T. ) ;
#56476=CARTESIAN_POINT ( 'NONE',  ( -49.38114550753920184, 1383.812931905830055, 260.0689200899579419 ) ) ;
#56477=CIRCLE ( 'NONE', #106585, 8.013264357029999729 ) ;
#56480=CARTESIAN_POINT ( 'NONE',  ( -9.095279969299012279, 1384.912302393732489, 199.9427318356120793 ) ) ;
#56485=CARTESIAN_POINT ( 'NONE',  ( -15.77939734220000112, 1380.225294738999992, 203.9934837876090228 ) ) ;
#56493=CARTESIAN_POINT ( 'NONE',  ( -10.77049225859999915, 1390.002812723860188, 215.5109487511890052 ) ) ;
#56497=CARTESIAN_POINT ( 'NONE',  ( -105.6627448849999951, 1378.306900235799958, 302.9594593028589884 ) ) ;
#56517=CARTESIAN_POINT ( 'NONE',  ( -109.1219531280000012, 1387.080370060750056, 310.9323500322590235 ) ) ;
#56526=CARTESIAN_POINT ( 'NONE',  ( -8.860009088490000906, 1384.987333740160011, 218.6842292965490060 ) ) ;
#56527=CARTESIAN_POINT ( 'NONE',  ( -14.40559916593009859, 1379.612683021279963, 208.0847104623620112 ) ) ;
#56541=CARTESIAN_POINT ( 'NONE',  ( -108.0096200556839960, 1378.913060387299993, 299.9536600820459853 ) ) ;
#56571=CARTESIAN_POINT ( 'NONE',  ( -109.0845216409653489, 1382.044982048102383, 297.5749921241352922 ) ) ;
#56575=DIRECTION ( 'NONE',  ( -1.000000000000000000, 0.000000000000000000, 0.000000000000000000 ) ) ;
#56582=CARTESIAN_POINT ( 'NONE',  ( -91.62647196664750027, 1384.965762749710166, 309.2156490120800072 ) ) ;
#56583=CARTESIAN_POINT ( 'NONE',  ( -9.503490513250000049, 1386.215136675220037, 200.2136258941289952 ) ) ;
#56596=CARTESIAN_POINT ( 'NONE',  ( -107.6011828208343672, 1389.768012669342397, 298.8907520829743021 ) ) ;
#56614=ADVANCED_FACE ( 'NONE', ( #27276 ), #110811, .T. ) ;
#56622=CARTESIAN_POINT ( 'NONE',  ( -103.9443829322484447, 1380.156439096358099, 306.3198609861664750 ) ) ;
#56628=CARTESIAN_POINT ( 'NONE',  ( -13.53521852579999951, 1379.959041148089909, 211.1154580547890021 ) ) ;
#56630=CARTESIAN_POINT ( 'NONE',  ( -66.14216747191879620, 1385.092570033629954, 257.5864158085420286 ) ) ;
#56642=CARTESIAN_POINT ( 'NONE',  ( -109.3106548430000089, 1384.781303703980029, 311.2625950142589772 ) ) ;
#56656=CARTESIAN_POINT ( 'NONE',  ( -5.187810489148779958, 1375.027207977500211, 203.4482692765930096 ) ) ;
#56662=CARTESIAN_POINT ( 'NONE',  ( -67.99816612459999021, 1379.747625308320039, 279.4122903082590028 ) ) ;
#56665=CARTESIAN_POINT ( 'NONE',  ( -8.813399063861234950, 1381.146817608087304, 217.8464237413924707 ) ) ;
#56690=CARTESIAN_POINT ( 'NONE',  ( -66.04910042496936740, 1379.741981372295641, 274.4777133012353261 ) ) ;
#56694=CARTESIAN_POINT ( 'NONE',  ( -79.38279021894339849, 1384.791171274589942, 282.2745212356039701 ) ) ;
#56730=CARTESIAN_POINT ( 'NONE',  ( -109.6762529225470075, 1383.331248784420040, 311.2558314816980101 ) ) ;
#56734=B_SPLINE_CURVE_WITH_KNOTS ( 'NONE', 3,
 ( #72743, #11191, #63802, #80587, #12264, #97918 ),
 .UNSPECIFIED., .F., .F.,
 ( 4, 2, 4 ),
 ( 0.000000000000000000, 0.5000000000000000000, 1.000000000000000000 ),
 .UNSPECIFIED. ) ;
#56761=CARTESIAN_POINT ( 'NONE',  ( -105.4624709189999834, 1391.255327103129957, 304.2078109453590287 ) ) ;
#56764=CARTESIAN_POINT ( 'NONE',  ( -23.61108870869020393, 1384.850736334059775, 222.7912172758710199 ) ) ;
#56768=CARTESIAN_POINT ( 'NONE',  ( -105.9362968920000014, 1378.913060259759959, 302.4576468725590530 ) ) ;
#56779=CARTESIAN_POINT ( 'NONE',  ( -14.08099615227689938, 1379.586030346570169, 211.7531778911580034 ) ) ;
#56789=CARTESIAN_POINT ( 'NONE',  ( -7.513427089629229449, 1380.366186910970100, 210.0680633349269897 ) ) ;
#56791=CARTESIAN_POINT ( 'NONE',  ( -19.23044006891440105, 1379.597748850580047, 212.7363834275300007 ) ) ;
#56817=CARTESIAN_POINT ( 'NONE',  ( -108.5763715352423162, 1388.342241357154990, 310.4916696162636640 ) ) ;
#56821=CARTESIAN_POINT ( 'NONE',  ( -13.15130281770530019, 1380.001591251920217, 209.0581075734310161 ) ) ;
#56822=ORIENTED_EDGE ( 'NONE', *, *, #46251, .F. ) ;
#56825=CARTESIAN_POINT ( 'NONE',  ( -44.32302097390000029, 1375.083786706710043, 232.1686497034590104 ) ) ;
#56826=EDGE_CURVE ( 'NONE', #26117, #61054, #15232, .T. ) ;
#56841=CARTESIAN_POINT ( 'NONE',  ( -32.10112702670000573, 1384.491500786489951, 229.9526432747589979 ) ) ;
#56855=CARTESIAN_POINT ( 'NONE',  ( -36.25711517340000256, 1386.837822767809939, 235.3814274622590119 ) ) ;
#56857=CARTESIAN_POINT ( 'NONE',  ( -43.39262373593199840, 1385.162178046419967, 248.3670905914219986 ) ) ;
#56866=CARTESIAN_POINT ( 'NONE',  ( -8.861964488639999971, 1384.888492400790028, 218.6850885747989821 ) ) ;
#56883=CARTESIAN_POINT ( 'NONE',  ( -104.1870796810000002, 1390.019597513000008, 303.0474178122589706 ) ) ;
#56886=CARTESIAN_POINT ( 'NONE',  ( -105.5460821599999974, 1391.484866075830041, 304.2071864700590140 ) ) ;
#56889=CARTESIAN_POINT ( 'NONE',  ( -104.4934867380000014, 1379.706082156179946, 304.0189722064590114 ) ) ;
#56904=CARTESIAN_POINT ( 'NONE',  ( -106.4241660069999966, 1383.759861017009825, 311.1380007012590454 ) ) ;
#56907=ORIENTED_EDGE ( 'NONE', *, *, #18438, .T. ) ;
#56942=CARTESIAN_POINT ( 'NONE',  ( -9.093004793099998651, 1384.764870898179879, 199.9460030570490119 ) ) ;
#56949=VERTEX_POINT ( 'NONE', #51672 ) ;
#56962=EDGE_CURVE ( 'NONE', #110163, #91726, #103274, .T. ) ;
#56966=CARTESIAN_POINT ( 'NONE',  ( -21.15898116937230000, 1384.535980822740157, 202.0007022378129875 ) ) ;
#56982=CARTESIAN_POINT ( 'NONE',  ( -68.78439012009999942, 1379.747952156290012, 280.2618955346589473 ) ) ;
#56999=DIRECTION ( 'NONE',  ( 1.000000000000000000, 0.000000000000000000, 0.000000000000000000 ) ) ;
#57006=AXIS2_PLACEMENT_3D ( 'NONE', #35153, #52526, #69896 ) ;
#57022=CARTESIAN_POINT ( 'NONE',  ( -109.1672625384930058, 1385.040948060030132, 297.1348415520359367 ) ) ;
#57040=CARTESIAN_POINT ( 'NONE',  ( -45.63068801059250035, 1383.819138085639906, 252.4128947413499873 ) ) ;
#57049=CARTESIAN_POINT ( 'NONE',  ( -9.645382992169999170, 1380.202965523560124, 203.3638893722689716 ) ) ;
#57054=CARTESIAN_POINT ( 'NONE',  ( -7.720734276493420367, 1386.472163584720192, 218.9022333215830258 ) ) ;
#57058=CARTESIAN_POINT ( 'NONE',  ( -106.7722198320000047, 1381.894365751589930, 298.4459716942589580 ) ) ;
#57079=CARTESIAN_POINT ( 'NONE',  ( -108.3907530290000096, 1386.531684817010046, 310.8877082452589775 ) ) ;
#57109=CARTESIAN_POINT ( 'NONE',  ( -58.30163007960000243, 1385.052442321870103, 240.0694839391589994 ) ) ;
#57136=CARTESIAN_POINT ( 'NONE',  ( -109.4064894422378558, 1382.584668033352500, 297.3600029045636006 ) ) ;
#57148=CARTESIAN_POINT ( 'NONE',  ( -89.61126119283551361, 1384.970433313389776, 308.5825330499230290 ) ) ;
#57151=CARTESIAN_POINT ( 'NONE',  ( -8.978047223340000826, 1387.343619535879952, 200.4278112474989939 ) ) ;
#57166=CARTESIAN_POINT ( 'NONE',  ( -108.3688902241231062, 1388.809589294943862, 298.1335643587438540 ) ) ;
#57190=CARTESIAN_POINT ( 'NONE',  ( -104.5461312646103949, 1380.583296262659132, 307.6660463617352548 ) ) ;
#57197=CARTESIAN_POINT ( 'NONE',  ( -12.32664273690000023, 1378.996295195989887, 209.7960013046609902 ) ) ;
#57199=CARTESIAN_POINT ( 'NONE',  ( -67.03515295860771062, 1385.097188996120167, 259.5578629473649812 ) ) ;
#57207=CARTESIAN_POINT ( 'NONE',  ( -109.6579480409999974, 1384.895131905899916, 311.3230545792589510 ) ) ;
#57227=CARTESIAN_POINT ( 'NONE',  ( -109.1205638390440100, 1384.635319001860125, 311.2541790391259724 ) ) ;
#57229=CARTESIAN_POINT ( 'NONE',  ( -68.43942151631850379, 1379.747151545919905, 280.0290128201230573 ) ) ;
#57242=CARTESIAN_POINT ( 'NONE',  ( -106.1750857939740058, 1378.913060388029862, 305.7883907182979897 ) ) ;
#57262=CARTESIAN_POINT ( 'NONE',  ( -13.84960889600000122, 1379.721631702780087, 208.1907843145939694 ) ) ;
#57269=CARTESIAN_POINT ( 'NONE',  ( -67.24941355666288700, 1384.719574498639986, 260.0378906380789772 ) ) ;
#57323=FACE_OUTER_BOUND ( 'NONE', #62798, .T. ) ;
#57337=CARTESIAN_POINT ( 'NONE',  ( -49.49141214366390074, 1384.742493838780092, 260.6926740138409855 ) ) ;
#57341=CARTESIAN_POINT ( 'NONE',  ( -105.6396896030000079, 1378.913059593480057, 303.5072247312590434 ) ) ;
#57353=CARTESIAN_POINT ( 'NONE',  ( -14.08980430995099908, 1379.613307177060051, 211.6683369410179978 ) ) ;
#57363=CARTESIAN_POINT ( 'NONE',  ( -24.78061434722729928, 1379.805010702669961, 214.9158369873429990 ) ) ;
#57365=CARTESIAN_POINT ( 'NONE',  ( -25.94019285366969996, 1379.613529776539963, 215.4482193062259796 ) ) ;
#57391=CARTESIAN_POINT ( 'NONE',  ( -107.8702472922463045, 1389.245402359266791, 309.8450691920539839 ) ) ;
#57393=CARTESIAN_POINT ( 'NONE',  ( -12.59193496205820040, 1379.616147050329801, 209.6906596629179944 ) ) ;
#57395=DIRECTION ( 'NONE',  ( 0.000000000000000000, -1.000000000000000000, 0.000000000000000000 ) ) ;
#57397=CARTESIAN_POINT ( 'NONE',  ( -35.85007572059999603, 1380.172836988449944, 220.5090016197590046 ) ) ;
#57410=DIRECTION ( 'NONE',  ( 0.000000000000000000, 1.000000000000000000, 0.000000000000000000 ) ) ;
#57412=CARTESIAN_POINT ( 'NONE',  ( -73.55923423229999969, 1384.652831667379814, 298.9494481685590017 ) ) ;
#57423=AXIS2_PLACEMENT_3D ( 'NONE', #1349, #58497, #109995 ) ;
#57425=CARTESIAN_POINT ( 'NONE',  ( -58.25011577389999928, 1386.675189637609947, 240.0949551211589892 ) ) ;
#57427=CARTESIAN_POINT ( 'NONE',  ( -52.23529040485620101, 1385.108628416219972, 266.3036918333839935 ) ) ;
#57437=CARTESIAN_POINT ( 'NONE',  ( -7.544964967010000301, 1384.904326039650186, 219.0876571199189868 ) ) ;
#57453=CARTESIAN_POINT ( 'NONE',  ( -106.6967271639999950, 1389.794052426160079, 299.6927497095589956 ) ) ;
#57468=CARTESIAN_POINT ( 'NONE',  ( -107.0308341067140105, 1383.759393728520081, 311.0596185783539340 ) ) ;
#57476=ORIENTED_EDGE ( 'NONE', *, *, #103236, .F. ) ;
#57503=CARTESIAN_POINT ( 'NONE',  ( -8.602588863709998535, 1384.842044605820092, 199.8691280033089868 ) ) ;
#57591=CARTESIAN_POINT ( 'NONE',  ( -51.92790261707470023, 1383.808767396460098, 265.2969453248350078 ) ) ;
#57605=CARTESIAN_POINT ( 'NONE',  ( -22.76979002380000239, 1383.850662563309925, 221.8906633995589743 ) ) ;
#57617=CARTESIAN_POINT ( 'NONE',  ( -105.3098427040000047, 1380.581413796420065, 300.2387618876589954 ) ) ;
#57622=CARTESIAN_POINT ( 'NONE',  ( -109.1450416020000063, 1385.242479493820156, 297.1468691531589457 ) ) ;
#57635=CARTESIAN_POINT ( 'NONE',  ( -109.7841757200000075, 1385.685848889800127, 311.3436617802590263 ) ) ;
#57646=CARTESIAN_POINT ( 'NONE',  ( -14.46232908324019917, 1379.641877967650089, 208.1640365550420029 ) ) ;
#57666=CARTESIAN_POINT ( 'NONE',  ( -46.07807520840000137, 1384.601971911739838, 219.0368719419589922 ) ) ;
#57697=CARTESIAN_POINT ( 'NONE',  ( -13.25845773799999883, 1379.879620654849987, 213.4412146779690147 ) ) ;
#57704=CARTESIAN_POINT ( 'NONE',  ( -9.369334600000000179, 1386.273946184829811, 200.2255685364590079 ) ) ;
#57737=CARTESIAN_POINT ( 'NONE',  ( -109.1647465200000084, 1384.889898235899864, 297.1327028377589841 ) ) ;
#57741=CARTESIAN_POINT ( 'NONE',  ( -103.8697664565839887, 1380.102834777972475, 306.0827998670219472 ) ) ;
#57747=CARTESIAN_POINT ( 'NONE',  ( -14.11636927220000004, 1379.895574107790026, 211.3023527909790005 ) ) ;
#57749=CARTESIAN_POINT ( 'NONE',  ( -63.27217475398849444, 1385.077751352280075, 251.1831659201390039 ) ) ;
#57762=CARTESIAN_POINT ( 'NONE',  ( -109.3085292789999983, 1384.876463481600013, 311.2645431242589780 ) ) ;
#57778=CARTESIAN_POINT ( 'NONE',  ( -68.45798957863590317, 1379.747194436310110, 280.0509092537030256 ) ) ;
#57780=CARTESIAN_POINT ( 'NONE',  ( -11.14562751756762893, 1378.415159664945577, 214.3954126917513179 ) ) ;
#57788=CARTESIAN_POINT ( 'NONE',  ( -107.9890416813189944, 1378.913060387289988, 308.4545676344260414 ) ) ;
#57808=CARTESIAN_POINT ( 'NONE',  ( -11.19935432940000020, 1391.089542290570080, 214.3845121043189863 ) ) ;
#57809=CARTESIAN_POINT ( 'NONE',  ( -67.03180608143330232, 1384.718158239579907, 259.5610210531770008 ) ) ;
#57833=DIRECTION ( 'NONE',  ( -1.836970198721029688E-16, -1.000000000000000000, 0.000000000000000000 ) ) ;
#57839=CARTESIAN_POINT ( 'NONE',  ( -8.371033105309999556, 1384.892342680180036, 199.7750073836789966 ) ) ;
#57857=CARTESIAN_POINT ( 'NONE',  ( -7.625768530968147552, 1386.113582989909901, 218.9869377475604324 ) ) ;
#57873=CARTESIAN_POINT ( 'NONE',  ( -109.1450416020000063, 1385.242479493820156, 297.1468691531589457 ) ) ;
#57874=CARTESIAN_POINT ( 'NONE',  ( -54.14820250061879392, 1384.720608453650129, 270.1448835903210011 ) ) ;
#57881=DIRECTION ( 'NONE',  ( 1.836970198721029688E-16, 1.000000000000000000, 0.000000000000000000 ) ) ;
#57882=CARTESIAN_POINT ( 'NONE',  ( -8.366802890251092251, 1382.852348275100667, 199.9076995699032011 ) ) ;
#57885=ORIENTED_EDGE ( 'NONE', *, *, #4271, .T. ) ;
#57900=CARTESIAN_POINT ( 'NONE',  ( -34.09660006530000231, 1376.882267573399986, 222.1544401288590223 ) ) ;
#57903=CARTESIAN_POINT ( 'NONE',  ( -40.81304585960000253, 1379.731884794059852, 229.1715070859589787 ) ) ;
#57931=CARTESIAN_POINT ( 'NONE',  ( -108.3146325907701026, 1388.689630667613756, 310.2700825005108527 ) ) ;
#57938=CARTESIAN_POINT ( 'NONE',  ( -11.40322695539999920, 1380.342188321789990, 209.3118815522890088 ) ) ;
#57950=CARTESIAN_POINT ( 'NONE',  ( -86.96730326719999482, 1384.052306858670136, 307.6473153112589785 ) ) ;
#57962=CARTESIAN_POINT ( 'NONE',  ( -70.43097214809999684, 1389.502223237589988, 273.8077508712590316 ) ) ;
#57964=CARTESIAN_POINT ( 'NONE',  ( -38.79897580568190563, 1385.188763823109866, 240.0467092869539840 ) ) ;
#57992=CARTESIAN_POINT ( 'NONE',  ( -105.2029017080000131, 1390.344333028660003, 302.0615195368590093 ) ) ;
#57995=CARTESIAN_POINT ( 'NONE',  ( -107.1612063080000041, 1391.913060387289988, 300.7260049596590079 ) ) ;
#58038=CARTESIAN_POINT ( 'NONE',  ( -110.0631611386010036, 1384.920974733809771, 296.9512360025400426 ) ) ;
#58043=FACE_OUTER_BOUND ( 'NONE', #102638, .T. ) ;
#58069=CARTESIAN_POINT ( 'NONE',  ( -46.70525487443880053, 1384.605919513219760, 220.5286058093979875 ) ) ;
#58113=CARTESIAN_POINT ( 'NONE',  ( -7.545139471115629881, 1384.910385469629773, 219.0876080393670122 ) ) ;
#58117=CARTESIAN_POINT ( 'NONE',  ( -109.1672562883220081, 1384.984605947210184, 297.1332200933230183 ) ) ;
#58122=LINE ( 'NONE', #107952, #99290 ) ;
#58134=CARTESIAN_POINT ( 'NONE',  ( -39.76728728541259983, 1383.828512391789900, 241.3785448166720187 ) ) ;
#58144=CARTESIAN_POINT ( 'NONE',  ( -48.18572634930000476, 1380.371872704240104, 227.8530853065590236 ) ) ;
#58148=CARTESIAN_POINT ( 'NONE',  ( -8.633823299111480054, 1386.054477820370039, 218.5393177817969956 ) ) ;
#58153=CARTESIAN_POINT ( 'NONE',  ( -105.5320588160000028, 1381.208403848540001, 299.1971426474589748 ) ) ;
#58157=CARTESIAN_POINT ( 'NONE',  ( -113.4000000000000057, 1378.913060387289988, 304.2218459572590064 ) ) ;
#58159=CARTESIAN_POINT ( 'NONE',  ( -108.8775172686859918, 1385.241885096709893, 297.1378884389180257 ) ) ;
#58171=CARTESIAN_POINT ( 'NONE',  ( -108.3896730050000059, 1388.605325449289921, 310.3517716152589969 ) ) ;
#58187=DIRECTION ( 'NONE',  ( -1.836970198721029688E-16, -1.000000000000000000, 0.000000000000000000 ) ) ;
#58199=CARTESIAN_POINT ( 'NONE',  ( -50.84956067560000292, 1384.888209502700192, 226.1736401165590280 ) ) ;
#58211=CARTESIAN_POINT ( 'NONE',  ( -10.62594761801030074, 1391.913060387249971, 205.0845642080600157 ) ) ;
#58233=CARTESIAN_POINT ( 'NONE',  ( -12.29033186280000045, 1380.572208205969901, 215.3566307603289829 ) ) ;
#58239=CARTESIAN_POINT ( 'NONE',  ( -12.14635843149999950, 1389.476265811170151, 203.8304572938190233 ) ) ;
#58268=ORIENTED_EDGE ( 'NONE', *, *, #43339, .F. ) ;
#58272=CARTESIAN_POINT ( 'NONE',  ( -110.0633064609999963, 1384.901791039720138, 296.9512369705590231 ) ) ;
#58276=CARTESIAN_POINT ( 'NONE',  ( -104.6561145012381928, 1380.660749972640588, 307.8568443802569732 ) ) ;
#58279=CARTESIAN_POINT ( 'NONE',  ( -109.0737800152069639, 1382.200485035640668, 310.8665753754681305 ) ) ;
#58281=CARTESIAN_POINT ( 'NONE',  ( -12.30978043270000022, 1378.957296234380237, 210.0572917626269884 ) ) ;
#58283=CARTESIAN_POINT ( 'NONE',  ( -53.45114155367870268, 1385.032075449320018, 231.0041225493250181 ) ) ;
#58284=CARTESIAN_POINT ( 'NONE',  ( -10.70151013563189935, 1391.913060387289988, 213.1790326816040135 ) ) ;
#58286=ORIENTED_EDGE ( 'NONE', *, *, #86710, .T. ) ;
#58292=CARTESIAN_POINT ( 'NONE',  ( -109.6575144030000075, 1384.919426084519955, 311.3230337842589961 ) ) ;
#58296=CARTESIAN_POINT ( 'NONE',  ( -109.2942948309999878, 1384.591425206880103, 311.2507045772590004 ) ) ;
#58310=CARTESIAN_POINT ( 'NONE',  ( -109.1645132478509908, 1384.901512804259937, 297.1326343494729940 ) ) ;
#58312=CARTESIAN_POINT ( 'NONE',  ( -68.55621501180290522, 1379.747479911359960, 280.1551959466660264 ) ) ;
#58347=CARTESIAN_POINT ( 'NONE',  ( -85.41229846784960955, 1384.819622699739966, 289.1167610944229978 ) ) ;
#58348=ORIENTED_EDGE ( 'NONE', *, *, #95410, .T. ) ;
#58358=DIRECTION ( 'NONE',  ( 0.9076061524720632212, 0.000000000000000000, -0.4198226673190215696 ) ) ;
#58364=CARTESIAN_POINT ( 'NONE',  ( -54.34609671659999464, 1379.710116771220100, 248.9718466677589959 ) ) ;
#58381=CARTESIAN_POINT ( 'NONE',  ( -7.966233669470000223, 1384.910919823659924, 199.4893341005590059 ) ) ;
#58385=CARTESIAN_POINT ( 'NONE',  ( -109.8241992154370053, 1383.739369478020080, 311.3440882120070228 ) ) ;
#58418=CARTESIAN_POINT ( 'NONE',  ( -52.91565643769759930, 1384.726266332619844, 267.6878703111970026 ) ) ;
#58425=CARTESIAN_POINT ( 'NONE',  ( -10.50535462500723938, 1379.632225880806118, 202.6061242926490422 ) ) ;
#58439=EDGE_CURVE ( 'NONE', #46666, #55409, #94837, .T. ) ;
#58445=CARTESIAN_POINT ( 'NONE',  ( -11.32057025491729974, 1380.342214975079969, 210.2587660409990349 ) ) ;
#58447=AXIS2_PLACEMENT_3D ( 'NONE', #50441, #59949, #75640 ) ;
#58448=CARTESIAN_POINT ( 'NONE',  ( -26.04300106147669780, 1379.718900503969962, 215.2617740064779923 ) ) ;
#58458=CARTESIAN_POINT ( 'NONE',  ( -1.658081806242819971E-15, 1375.886883438980021, 209.1218459572589836 ) ) ;
#58476=CARTESIAN_POINT ( 'NONE',  ( -109.8754351979164738, 1385.888632332895668, 311.3751271473491329 ) ) ;
#58483=CARTESIAN_POINT ( 'NONE',  ( -11.47183536569999873, 1380.342188321910044, 208.5259290606079787 ) ) ;
#58484=ORIENTED_EDGE ( 'NONE', *, *, #52321, .T. ) ;
#58492=EDGE_CURVE ( 'NONE', #60257, #50191, #12515, .T. ) ;
#58497=DIRECTION ( 'NONE',  ( 1.835183309750130004E-16, 1.000000000000000000, 1.599799320660000123E-19 ) ) ;
#58502=ADVANCED_FACE ( 'NONE', ( #60822 ), #68008, .T. ) ;
#58511=CARTESIAN_POINT ( 'NONE',  ( -44.22662318030000250, 1388.378119737989891, 246.9464660031590029 ) ) ;
#58513=CARTESIAN_POINT ( 'NONE',  ( -50.55048253121940149, 1385.118695880380074, 262.8599624479500108 ) ) ;
#58521=CIRCLE ( 'NONE', #10228, 7.999657266239995401 ) ;
#58539=CARTESIAN_POINT ( 'NONE',  ( -105.5774816291841915, 1391.233265412462515, 302.6220820957303772 ) ) ;
#58542=CARTESIAN_POINT ( 'NONE',  ( -109.5642235760000034, 1387.004236421979840, 297.2531471322589596 ) ) ;
#58565=ORIENTED_EDGE ( 'NONE', *, *, #52321, .F. ) ;
#58573=CARTESIAN_POINT ( 'NONE',  ( -12.29271509424149933, 1378.291405090629951, 210.0354033918439995 ) ) ;
#58591=CARTESIAN_POINT ( 'NONE',  ( -7.973835201749999158, 1384.482862421380105, 199.5100561111489981 ) ) ;
#58611=CARTESIAN_POINT ( 'NONE',  ( -109.5441724480000119, 1378.507830972490183, 302.0293835567589440 ) ) ;
#58616=CARTESIAN_POINT ( 'NONE',  ( -36.69594268719530561, 1384.573250885219977, 210.0209466372170084 ) ) ;
#58617=CARTESIAN_POINT ( 'NONE',  ( -14.48969036947769951, 1379.662410256569956, 208.2055791338830204 ) ) ;
#58624=CARTESIAN_POINT ( 'NONE',  ( -9.393822458599998981, 1383.815214525520105, 200.1452963205690025 ) ) ;
#58629=CARTESIAN_POINT ( 'NONE',  ( -68.79001571249999358, 1379.747967232289966, 280.2970183437590208 ) ) ;
#58650=CARTESIAN_POINT ( 'NONE',  ( -8.859802060015358194, 1385.025244372899806, 218.6830422513599785 ) ) ;
#58680=CONICAL_SURFACE ( 'NONE', #108788, 7.999999999999996447, 0.02617993877989872875 ) ;
#58683=CARTESIAN_POINT ( 'NONE',  ( -63.80571065684490151, 1383.791867485110060, 286.7071051378580364 ) ) ;
#58691=CARTESIAN_POINT ( 'NONE',  ( -70.73284055979999607, 1380.574797240599992, 273.6446839984589587 ) ) ;
#58696=CARTESIAN_POINT ( 'NONE',  ( -8.080339290932069929, 1386.284300861730117, 218.6800679842810098 ) ) ;
#58701=CARTESIAN_POINT ( 'NONE',  ( -105.8961900970000016, 1378.203726956179935, 301.8257929996590292 ) ) ;
#58704=AXIS2_PLACEMENT_3D ( 'NONE', #63811, #3362, #21195 ) ;
#58719=CARTESIAN_POINT ( 'NONE',  ( -105.7870492409999912, 1391.295072527720095, 306.5714272217589951 ) ) ;
#58726=CARTESIAN_POINT ( 'NONE',  ( -11.39903424189999903, 1388.037600957480208, 201.7885523045490004 ) ) ;
#58743=ORIENTED_EDGE ( 'NONE', *, *, #89858, .T. ) ;
#58756=CARTESIAN_POINT ( 'NONE',  ( -10.50394959559160135, 1391.913060387279984, 204.8107535540119954 ) ) ;
#58778=DIRECTION ( 'NONE',  ( 1.836970198721029688E-16, 1.000000000000000000, 0.000000000000000000 ) ) ;
#58779=CARTESIAN_POINT ( 'NONE',  ( -11.76384282640000123, 1377.860255930400172, 212.8274665997790009 ) ) ;
#58785=CARTESIAN_POINT ( 'NONE',  ( -12.31074584409999950, 1391.522609710569895, 206.9351367010589797 ) ) ;
#58813=B_SPLINE_CURVE_WITH_KNOTS ( 'NONE', 5,
 ( #27981, #86227, #43686, #62166, #54318, #61071, #1147, #103014, #96857, #96292, #20126, #52646, #17899, #19571, #103580, #26882, #95188, #18447, #86783, #87343, #10072, #44247, #27422, #61605, #19002, #91191, #55406, #81670, #38041, #107987, #4976, #97929, #89538, #4448, #71693, #46464, #88984, #99026, #105812, #3911, #72220, #82240, #106342, #81131, #106881, #12272, #90076, #72752 ),
 .UNSPECIFIED., .F., .F.,
 ( 6, 3, 3, 3, 3, 3, 3, 3, 3, 3, 3, 3, 3, 3, 3, 6 ),
 ( 0.000000000000000000, 0.1188772993508104975, 0.2620754547158732350, 0.4767847777604456994, 0.6196881868957598849, 0.7909627338043010436, 0.8908775806277737797, 0.9289413061621332179, 0.9543180330005532896, 0.9712371219245071741, 0.9825186400522594177, 0.9900448187280238566, 0.9950985928942978065, 0.9968304128275284892, 0.9985622327607588389, 1.000000000000000000 ),
 .UNSPECIFIED. ) ;
#58817=CARTESIAN_POINT ( 'NONE',  ( -109.3494421689999996, 1384.898366538659957, 297.1385770996590168 ) ) ;
#58822=CARTESIAN_POINT ( 'NONE',  ( -105.2354452277541554, 1381.066582002241830, 308.6640088333896870 ) ) ;
#58828=CARTESIAN_POINT ( 'NONE',  ( -14.08142779579999981, 1379.709124900479765, 211.5303545317289888 ) ) ;
#58831=CARTESIAN_POINT ( 'NONE',  ( -79.38120359113469249, 1385.155067698849962, 282.2779454254330176 ) ) ;
#58862=CARTESIAN_POINT ( 'NONE',  ( -68.43062188917149058, 1379.747186918749776, 280.0365307058419830 ) ) ;
#58877=CARTESIAN_POINT ( 'NONE',  ( -109.1655177890000061, 1384.872414444939977, 297.1329087538589420 ) ) ;
#58896=CARTESIAN_POINT ( 'NONE',  ( -93.46913709372920209, 1384.851876627109959, 294.3416048512119687 ) ) ;
#58915=CARTESIAN_POINT ( 'NONE',  ( -56.85802524500000033, 1379.713981567250130, 254.2456484369590157 ) ) ;
#58930=CARTESIAN_POINT ( 'NONE',  ( -9.095184790679999409, 1384.908537446980063, 199.9427583283290062 ) ) ;
#58961=CARTESIAN_POINT ( 'NONE',  ( -12.14288099779810715, 1377.667352148589998, 211.1463812155207052 ) ) ;
#58966=CARTESIAN_POINT ( 'NONE',  ( -53.95864250903900228, 1384.721469025669876, 269.7706786227579983 ) ) ;
#58967=CARTESIAN_POINT ( 'NONE',  ( -106.9811535215749956, 1391.913060387289988, 301.7491911334220163 ) ) ;
#58970=CARTESIAN_POINT ( 'NONE',  ( -108.2039567000000062, 1378.913060387289988, 299.7295690323589952 ) ) ;
#58977=CARTESIAN_POINT ( 'NONE',  ( -10.17189341190630358, 1380.026521348481310, 202.0760537856158976 ) ) ;
#58981=ADVANCED_FACE ( 'NONE', ( #63457 ), #104397, .T. ) ;
#58995=EDGE_CURVE ( 'NONE', #67802, #73303, #74039, .T. ) ;
#59003=CARTESIAN_POINT ( 'NONE',  ( -33.96591335708179571, 1378.821001449670121, 222.2770748186169953 ) ) ;
#59006=CARTESIAN_POINT ( 'NONE',  ( -21.72241338915559794, 1379.603549772170254, 213.5570291714129780 ) ) ;
#59013=FACE_OUTER_BOUND ( 'NONE', #94959, .T. ) ;
#59035=AXIS2_PLACEMENT_3D ( 'NONE', #87187, #45207, #12128 ) ;
#59042=CARTESIAN_POINT ( 'NONE',  ( 5.105014162403789241E-14, 1376.342264060500156, 206.9293834673690071 ) ) ;
#59055=CARTESIAN_POINT ( 'NONE',  ( -102.7434157679999913, 1384.036053956720025, 311.1373841372590050 ) ) ;
#59068=CARTESIAN_POINT ( 'NONE',  ( -52.50755113500000704, 1388.282985474849966, 231.2999456731590158 ) ) ;
#59070=CARTESIAN_POINT ( 'NONE',  ( -53.77332582030280150, 1385.099635535869993, 269.3953241406759957 ) ) ;
#59084=CARTESIAN_POINT ( 'NONE',  ( -108.7920667164509894, 1381.754968429450173, 310.6777004439369989 ) ) ;
#59097=CARTESIAN_POINT ( 'NONE',  ( -108.5296511849999916, 1386.299881632349980, 297.3615022879590128 ) ) ;
#59134=CARTESIAN_POINT ( 'NONE',  ( -12.30596913808479975, 1378.368950717130019, 209.8692018423830064 ) ) ;
#59178=CARTESIAN_POINT ( 'NONE',  ( -46.34909325035440020, 1384.604549084440123, 220.0612681586810311 ) ) ;
#59186=CARTESIAN_POINT ( 'NONE',  ( -53.46082045212465772, 1379.704646932813830, 252.6341302468160848 ) ) ;
#59191=CARTESIAN_POINT ( 'NONE',  ( -68.57934351740000523, 1379.747889361729904, 279.7331283945590030 ) ) ;
#59199=CARTESIAN_POINT ( 'NONE',  ( -5.958828918610000080, 1384.900097640590047, 218.5255276338789940 ) ) ;
#59217=ORIENTED_EDGE ( 'NONE', *, *, #55721, .T. ) ;
#59240=CARTESIAN_POINT ( 'NONE',  ( -12.61172662586290016, 1379.083473090599909, 208.5076072890859962 ) ) ;
#59244=CARTESIAN_POINT ( 'NONE',  ( -60.45726899866969717, 1383.796084930870165, 281.3943264362069954 ) ) ;
#59252=CARTESIAN_POINT ( 'NONE',  ( -68.70547844060000386, 1384.729371863979850, 263.4329467144589785 ) ) ;
#59258=CARTESIAN_POINT ( 'NONE',  ( -8.235011779212388916, 1386.670742518729867, 218.5434337873010122 ) ) ;
#59260=DIRECTION ( 'NONE',  ( -0.1306151939486110136, 0.9872726063158969723, 0.09073297045717730602 ) ) ;
#59263=CARTESIAN_POINT ( 'NONE',  ( -109.2936197549999946, 1383.544291963839896, 297.2875327422589748 ) ) ;
#59287=CARTESIAN_POINT ( 'NONE',  ( -107.0296446230000100, 1389.965289768990033, 308.9939284075589399 ) ) ;
#59296=CARTESIAN_POINT ( 'NONE',  ( -9.094129269030000629, 1384.954944735329946, 199.9429221374590213 ) ) ;
#59334=DIRECTION ( 'NONE',  ( 0.0001373912891020987869, 0.01108474315567990406, -0.9999385529085306201 ) ) ;
#59339=CARTESIAN_POINT ( 'NONE',  ( -3.078458355400000013, 1386.601749568020068, 199.6726121090490267 ) ) ;
#59349=CARTESIAN_POINT ( 'NONE',  ( -11.35047539859999866, 1380.036999151499913, 215.0867406839389844 ) ) ;
#59354=CARTESIAN_POINT ( 'NONE',  ( -108.7828337545389985, 1384.925007157400159, 311.2643083153219550 ) ) ;
#59355=CARTESIAN_POINT ( 'NONE',  ( -13.55796854679999974, 1390.272843676579896, 206.9364406775789860 ) ) ;
#59390=CARTESIAN_POINT ( 'NONE',  ( -5.930127944598649670, 1391.913057044489960, 203.1301316852850221 ) ) ;
#59395=CARTESIAN_POINT ( 'NONE',  ( -108.5877928923653570, 1381.490933517691019, 310.5017133838013592 ) ) ;
#59398=CARTESIAN_POINT ( 'NONE',  ( -11.73107767829999837, 1391.121393030069839, 205.1223722441990276 ) ) ;
#59399=CARTESIAN_POINT ( 'NONE',  ( -79.01945392300798687, 1385.153591211519824, 281.7696847378040275 ) ) ;
#59407=ORIENTED_EDGE ( 'NONE', *, *, #75470, .T. ) ;
#59425=CARTESIAN_POINT ( 'NONE',  ( -68.58629774669110191, 1379.747539349169983, 280.1877734521850130 ) ) ;
#59438=PRESENTATION_STYLE_ASSIGNMENT (( #42069 ) ) ;
#59451=CARTESIAN_POINT ( 'NONE',  ( -14.23346546853939998, 1380.249845882129875, 210.5096821227170096 ) ) ;
#59460=CARTESIAN_POINT ( 'NONE',  ( -97.29693749981930750, 1384.865312593040244, 295.6567534606039658 ) ) ;
#59476=CARTESIAN_POINT ( 'NONE',  ( -57.93277555979999960, 1379.748264674359916, 257.2455319417590545 ) ) ;
#59489=VERTEX_POINT ( 'NONE', #102379 ) ;
#59496=DIRECTION ( 'NONE',  ( -1.836970198721029688E-16, -1.000000000000000000, 0.000000000000000000 ) ) ;
#59507=CARTESIAN_POINT ( 'NONE',  ( -8.363594539798167915, 1387.928394511323859, 218.3056381099177941 ) ) ;
#59524=CARTESIAN_POINT ( 'NONE',  ( -60.96793211269689294, 1384.692043816230125, 282.5782060957649833 ) ) ;
#59525=CARTESIAN_POINT ( 'NONE',  ( -18.51341249058109995, 1384.948111255019967, 201.2951208967390073 ) ) ;
#59527=CARTESIAN_POINT ( 'NONE',  ( -107.1138176589999915, 1379.788324461719867, 299.4659512524589786 ) ) ;
#59539=CARTESIAN_POINT ( 'NONE',  ( -8.435900379319999587, 1384.078873582379856, 199.8582732524889991 ) ) ;
#59552=CARTESIAN_POINT ( 'NONE',  ( -56.94149478592599678, 1379.719693845439906, 259.4788933646619853 ) ) ;
#59559=CARTESIAN_POINT ( 'NONE',  ( -109.1310718750000177, 1384.930040066290076, 311.2646600702590263 ) ) ;
#59585=CARTESIAN_POINT ( 'NONE',  ( -18.96272001720000233, 1375.296266888390164, 209.6316668867899864 ) ) ;
#59612=CARTESIAN_POINT ( 'NONE',  ( -62.13760418270000230, 1386.639474965800218, 284.7250346138590089 ) ) ;
#59614=CARTESIAN_POINT ( 'NONE',  ( -67.42891481536051401, 1385.033601920959882, 291.9986235379319623 ) ) ;
#59627=CARTESIAN_POINT ( 'NONE',  ( -107.6137522180000019, 1380.536624878880275, 309.5969479812590066 ) ) ;
#59676=CARTESIAN_POINT ( 'NONE',  ( -21.44030951619999925, 1380.278426299410057, 211.4934892549489973 ) ) ;
#59702=CARTESIAN_POINT ( 'NONE',  ( -11.97267500829999953, 1391.195698933469885, 205.7774971565190185 ) ) ;
#59714=FACE_OUTER_BOUND ( 'NONE', #22590, .T. ) ;
#59719=CARTESIAN_POINT ( 'NONE',  ( -41.28896974651279805, 1384.586842369110173, 214.1824021301610230 ) ) ;
#59727=CARTESIAN_POINT ( 'NONE',  ( -47.88884525074264076, 1379.684776574018997, 241.7622029387366922 ) ) ;
#59731=CARTESIAN_POINT ( 'NONE',  ( -68.69916525130000196, 1379.747766825639928, 279.9854416248589928 ) ) ;
#59759=FACE_OUTER_BOUND ( 'NONE', #36385, .T. ) ;
#59767=CARTESIAN_POINT ( 'NONE',  ( -7.545141261034559399, 1384.919253706480049, 219.0875759670219907 ) ) ;
#59790=CARTESIAN_POINT ( 'NONE',  ( -53.74473075458050175, 1383.805872317579997, 268.9597808447719558 ) ) ;
#59797=CARTESIAN_POINT ( 'NONE',  ( -40.27282834620000074, 1380.934810191280121, 238.2933727449590151 ) ) ;
#59808=CARTESIAN_POINT ( 'NONE',  ( -108.7999967259999892, 1381.610864533399990, 297.7780583747590413 ) ) ;
#59831=CARTESIAN_POINT ( 'NONE',  ( -105.8118099419999965, 1391.581618872429999, 306.6506172913590262 ) ) ;
#59839=EDGE_CURVE ( 'NONE', #29176, #17951, #4350, .T. ) ;
#59862=CARTESIAN_POINT ( 'NONE',  ( -110.0482597500069915, 1385.373319905469771, 296.9711118272649628 ) ) ;
#59864=CARTESIAN_POINT ( 'NONE',  ( -109.9850845680699933, 1384.907642987549934, 311.4561493310270066 ) ) ;
#59892=CARTESIAN_POINT ( 'NONE',  ( -113.4000000000000057, 1390.939237335599955, 304.2218459572590064 ) ) ;
#59894=CARTESIAN_POINT ( 'NONE',  ( -13.41289550449999979, 1379.525782299150023, 211.7978701437990026 ) ) ;
#59904=CARTESIAN_POINT ( 'NONE',  ( -12.36594955309999833, 1391.700202007920097, 209.7454160267469945 ) ) ;
#59915=B_SPLINE_CURVE_WITH_KNOTS ( 'NONE', 5,
 ( #97546, #20817, #48814, #106495, #38726, #21900, #23016, #107041, #6227, #67268, #32544, #109260 ),
 .UNSPECIFIED., .F., .F.,
 ( 6, 3, 3, 6 ),
 ( 0.000000000000000000, 0.4545476142708403944, 0.7388436783044410872, 1.000000000000000000 ),
 .UNSPECIFIED. ) ;
#59947=CARTESIAN_POINT ( 'NONE',  ( -108.3047457728057452, 1381.116487792409089, 310.2605079287397416 ) ) ;
#59949=DIRECTION ( 'NONE',  ( 0.000000000000000000, -1.000000000000000000, 0.000000000000000000 ) ) ;
#59951=FACE_OUTER_BOUND ( 'NONE', #16969, .T. ) ;
#59952=CARTESIAN_POINT ( 'NONE',  ( -81.15982276781578264, 1385.162085608370035, 284.5929643925970254 ) ) ;
#59953=CARTESIAN_POINT ( 'NONE',  ( -11.03830765538920033, 1391.913060387289988, 212.4289022242699900 ) ) ;
#59989=CARTESIAN_POINT ( 'NONE',  ( -12.57793359742250061, 1378.943374723730130, 208.9206934522059953 ) ) ;
#60009=CARTESIAN_POINT ( 'NONE',  ( -90.07606196291349931, 1384.838993735919985, 292.6108296685719665 ) ) ;
#60028=CARTESIAN_POINT ( 'NONE',  ( -21.14027738949999957, 1379.625625016810091, 209.6601806591559978 ) ) ;
#60078=CARTESIAN_POINT ( 'NONE',  ( -12.16766253904543582, 1377.701433628964878, 210.9975495011200053 ) ) ;
#60083=CARTESIAN_POINT ( 'NONE',  ( -81.23110265244889661, 1384.636034499739935, 304.6366948209559951 ) ) ;
#60099=CARTESIAN_POINT ( 'NONE',  ( -8.920215095379999681, 1384.216085512750169, 199.9962620032089831 ) ) ;
#60112=CARTESIAN_POINT ( 'NONE',  ( -64.37783753600000125, 1379.747207013510206, 273.6112401810589745 ) ) ;
#60118=CARTESIAN_POINT ( 'NONE',  ( -107.1765804579999894, 1378.913059918550061, 307.8836185913590384 ) ) ;
#60120=CARTESIAN_POINT ( 'NONE',  ( -8.606575390850000673, 1385.345214380770130, 218.6410135246489972 ) ) ;
#60142=CARTESIAN_POINT ( 'NONE',  ( -35.68475374490700602, 1379.642202425360210, 218.6381764093407867 ) ) ;
#60143=CARTESIAN_POINT ( 'NONE',  ( -25.65041448810000091, 1380.250345454750004, 213.2122020707489867 ) ) ;
#60171=CARTESIAN_POINT ( 'NONE',  ( -98.86683315710000386, 1385.218296336320009, 296.2584199137589849 ) ) ;
#60173=CARTESIAN_POINT ( 'NONE',  ( -57.94198640639650222, 1385.076618372680059, 277.3417116979370007 ) ) ;
#60184=CARTESIAN_POINT ( 'NONE',  ( -108.7025099737439859, 1381.872732176050022, 310.6179191028680293 ) ) ;
#60210=CARTESIAN_POINT ( 'NONE',  ( -10.00342135130719967, 1384.890128760720017, 218.7594294872120031 ) ) ;
#60217=EDGE_LOOP ( 'NONE', ( #102823, #43582, #15442, #87411 ) ) ;
#60257=VERTEX_POINT ( 'NONE', #70869 ) ;
#60270=CARTESIAN_POINT ( 'NONE',  ( -64.53706522309998661, 1385.084217465399888, 254.0329369609589776 ) ) ;
#60272=CARTESIAN_POINT ( 'NONE',  ( -39.24126402133479985, 1384.580542155480089, 212.2021475517339866 ) ) ;
#60274=CARTESIAN_POINT ( 'NONE',  ( -107.6642996119999935, 1387.006294017490063, 310.6297471052590140 ) ) ;
#60282=CARTESIAN_POINT ( 'NONE',  ( -68.73472092510000664, 1379.747979032470084, 280.1061875640590415 ) ) ;
#60288=DIRECTION ( 'NONE',  ( 0.03204755514876567873, 0.01239821417688169794, 0.9994094448694244015 ) ) ;
#60290=CARTESIAN_POINT ( 'NONE',  ( -59.23371022229999738, 1384.698177673139980, 279.9261678725590059 ) ) ;
#60293=CARTESIAN_POINT ( 'NONE',  ( -13.61444516352630174, 1385.299542045740054, 219.1554977703900136 ) ) ;
#60304=CARTESIAN_POINT ( 'NONE',  ( -8.880888756510550763, 1385.269894070959708, 218.6655104340140099 ) ) ;
#60313=CARTESIAN_POINT ( 'NONE',  ( -105.4624709189999834, 1391.255327103129957, 304.2078109453590287 ) ) ;
#60330=CIRCLE ( 'NONE', #83483, 7.999657266239995401 ) ;
#60339=CARTESIAN_POINT ( 'NONE',  ( -71.42280142184640113, 1383.783904420230101, 296.3576773952639769 ) ) ;
#60346=CARTESIAN_POINT ( 'NONE',  ( -87.00440039350000632, 1383.772198133360007, 307.5612418777589596 ) ) ;
#60348=EDGE_LOOP ( 'NONE', ( #57885, #82090, #33085, #52435 ) ) ;
#60357=CARTESIAN_POINT ( 'NONE',  ( -109.2946818930000035, 1382.595360700089941, 297.4130465109590205 ) ) ;
#60382=CARTESIAN_POINT ( 'NONE',  ( -108.4825948470000014, 1386.816125860719922, 310.7856892562589906 ) ) ;
#60415=ADVANCED_FACE ( 'NONE', ( #101253 ), #6149, .T. ) ;
#60436=CARTESIAN_POINT ( 'NONE',  ( -6.285004828870000004, 1389.626702675270053, 203.0565589641389863 ) ) ;
#60437=CARTESIAN_POINT ( 'NONE',  ( -8.888758267720000106, 1385.314821192629779, 218.6605176881890031 ) ) ;
#60442=CARTESIAN_POINT ( 'NONE',  ( -14.03293030814504050, 1379.586391581537555, 211.8749277816402810 ) ) ;
#60446=CARTESIAN_POINT ( 'NONE',  ( -10.97164840699999999, 1381.332427371100039, 216.7312293341890097 ) ) ;
#60454=CARTESIAN_POINT ( 'NONE',  ( -11.15749597250000136, 1390.963088241619971, 203.6399077860090188 ) ) ;
#60490=CARTESIAN_POINT ( 'NONE',  ( -14.40730585596589997, 1380.239382581250084, 209.2612549436819904 ) ) ;
#60496=CARTESIAN_POINT ( 'NONE',  ( -109.0574111638984505, 1382.174802844307578, 310.8550843848203158 ) ) ;
#60499=CARTESIAN_POINT ( 'NONE',  ( -10.81171441090000052, 1391.913060387289988, 204.7749328824690167 ) ) ;
#60500=CARTESIAN_POINT ( 'NONE',  ( -68.46831016306249751, 1385.104556025459942, 262.6710340492040245 ) ) ;
#60529=CARTESIAN_POINT ( 'NONE',  ( -68.77190087506669158, 1379.747925807530009, 280.3125204381590265 ) ) ;
#60545=CARTESIAN_POINT ( 'NONE',  ( -14.08326878217680012, 1379.708207602939865, 208.2775395970890031 ) ) ;
#60559=CARTESIAN_POINT ( 'NONE',  ( -14.29942586552730077, 1380.320760441320090, 210.0466192271150021 ) ) ;
#60567=CARTESIAN_POINT ( 'NONE',  ( -11.66658881389999891, 1391.913060387289988, 209.7119989811589846 ) ) ;
#60568=CARTESIAN_POINT ( 'NONE',  ( -88.50299786935610769, 1384.832684027770028, 291.5890375481939714 ) ) ;
#60585=CARTESIAN_POINT ( 'NONE',  ( -18.89554632140000479, 1379.602095017590045, 208.7270065393099969 ) ) ;
#60604=CARTESIAN_POINT ( 'NONE',  ( -115.5939564047259296, 1390.913060387289988, 305.4204098037694735 ) ) ;
#60605=CARTESIAN_POINT ( 'NONE',  ( -12.23669307423070052, 1377.661331666050273, 207.7794331870949804 ) ) ;
#60639=CARTESIAN_POINT ( 'NONE',  ( -82.95076918121009157, 1384.632580800539927, 305.6340335797960392 ) ) ;
#60640=CARTESIAN_POINT ( 'NONE',  ( -28.06373293278850056, 1384.965165955840121, 204.5801626712980124 ) ) ;
#60645=CARTESIAN_POINT ( 'NONE',  ( -8.847652261760000414, 1384.947871987750204, 199.9248388310690245 ) ) ;
#60651=EDGE_CURVE ( 'NONE', #59489, #33248, #101672, .T. ) ;
#60657=CARTESIAN_POINT ( 'NONE',  ( -8.627683608919999969, 1383.470579637440096, 200.0452354592789845 ) ) ;
#60671=CARTESIAN_POINT ( 'NONE',  ( -59.57269385937500061, 1379.722641775480042, 264.7994946068799891 ) ) ;
#60707=CARTESIAN_POINT ( 'NONE',  ( -35.65618109042815576, 1379.642124534350387, 218.6101405679489176 ) ) ;
#60714=ORIENTED_EDGE ( 'NONE', *, *, #54852, .F. ) ;
#60715=CARTESIAN_POINT ( 'NONE',  ( -105.5930000624190086, 1378.287466303110023, 305.0491164647540359 ) ) ;
#60738=CARTESIAN_POINT ( 'NONE',  ( -85.13767067070000394, 1388.281031823789817, 290.5355680588589848 ) ) ;
#60749=CARTESIAN_POINT ( 'NONE',  ( -108.0218370616639874, 1383.106230495490308, 310.8121610381319897 ) ) ;
#60750=ORIENTED_EDGE ( 'NONE', *, *, #86442, .F. ) ;
#60763=CARTESIAN_POINT ( 'NONE',  ( -109.7278721679999904, 1385.840206276699973, 297.1154854894589903 ) ) ;
#60767=ORIENTED_EDGE ( 'NONE', *, *, #36509, .F. ) ;
#60778=CARTESIAN_POINT ( 'NONE',  ( -17.51671525713139843, 1384.869800455989889, 220.0655268698560008 ) ) ;
#60822=FACE_OUTER_BOUND ( 'NONE', #72532, .T. ) ;
#60834=CARTESIAN_POINT ( 'NONE',  ( -105.6883447180000104, 1374.461008904089795, 304.2218452742590102 ) ) ;
#60841=CARTESIAN_POINT ( 'NONE',  ( -50.84652256599999731, 1385.021217850319999, 226.1755936018590205 ) ) ;
#60842=CARTESIAN_POINT ( 'NONE',  ( -65.64734824971920091, 1384.709125050150305, 256.5005590946320240 ) ) ;
#60854=CARTESIAN_POINT ( 'NONE',  ( -68.68965169780000224, 1379.747958860950121, 279.9890510275590145 ) ) ;
#60863=CARTESIAN_POINT ( 'NONE',  ( -27.62433227900000077, 1384.972991153419798, 225.6333370715589979 ) ) ;
#60864=ORIENTED_EDGE ( 'NONE', *, *, #58492, .T. ) ;
#60865=CARTESIAN_POINT ( 'NONE',  ( -15.94747805094890225, 1385.291421466249858, 219.6205707809359922 ) ) ;
#60907=CARTESIAN_POINT ( 'NONE',  ( -58.77327825612210432, 1383.798380756109964, 278.4814665550280210 ) ) ;
#60910=DIRECTION ( 'NONE',  ( -0.9702683578407158560, 7.674209871302701496E-33, 0.2420316379589265432 ) ) ;
#60914=CARTESIAN_POINT ( 'NONE',  ( -78.74259975059999306, 1381.827890489759966, 283.5083833816589731 ) ) ;
#60924=CARTESIAN_POINT ( 'NONE',  ( -108.9551702540000093, 1381.838302694970025, 297.6631244000589618 ) ) ;
#60987=CARTESIAN_POINT ( 'NONE',  ( -11.67647783385400118, 1391.913060387289988, 209.3864368603249773 ) ) ;
#60994=VERTEX_POINT ( 'NONE', #27760 ) ;
#61000=CARTESIAN_POINT ( 'NONE',  ( -16.15572484810000020, 1388.284171620699908, 201.6770185590890208 ) ) ;
#61008=DIRECTION ( 'NONE',  ( 1.836970198721029688E-16, 1.000000000000000000, 0.000000000000000000 ) ) ;
#61009=CARTESIAN_POINT ( 'NONE',  ( -9.032305492669999936, 1381.079015021919986, 217.6610502493890067 ) ) ;
#61051=CARTESIAN_POINT ( 'NONE',  ( -6.325225975639999554, 1381.402069227939819, 201.1200243473190028 ) ) ;
#61054=VERTEX_POINT ( 'NONE', #104502 ) ;
#61060=CARTESIAN_POINT ( 'NONE',  ( -13.97255973646679905, 1390.368318560739908, 209.8293641130019864 ) ) ;
#61067=CARTESIAN_POINT ( 'NONE',  ( -12.26982168579999843, 1378.706401005240195, 210.4710064293389848 ) ) ;
#61068=CARTESIAN_POINT ( 'NONE',  ( -12.50888813809999967, 1391.368279522899911, 208.1679514191799854 ) ) ;
#61069=CARTESIAN_POINT ( 'NONE',  ( -71.50884848185910414, 1385.119804080199856, 268.9689710269449847 ) ) ;
#61071=CARTESIAN_POINT ( 'NONE',  ( -30.32475187390000215, 1379.724315040820102, 214.4187306602189835 ) ) ;
#61079=EDGE_LOOP ( 'NONE', ( #70338, #55068, #2831 ) ) ;
#61098=ORIENTED_EDGE ( 'NONE', *, *, #31174, .T. ) ;
#61100=VERTEX_POINT ( 'NONE', #21022 ) ;
#61110=CARTESIAN_POINT ( 'NONE',  ( -12.61627177722139947, 1378.992494172049874, 208.8788604928810173 ) ) ;
#61114=VERTEX_POINT ( 'NONE', #109475 ) ;
#61131=CARTESIAN_POINT ( 'NONE',  ( -11.63792774969999932, 1391.913060387289988, 210.2958033881990048 ) ) ;
#61132=CARTESIAN_POINT ( 'NONE',  ( -102.2551658410750122, 1384.881266493530120, 296.6246253060550089 ) ) ;
#61155=CARTESIAN_POINT ( 'NONE',  ( -68.63354038381854139, 1379.747798109386622, 280.2252688739458790 ) ) ;
#61186=CARTESIAN_POINT ( 'NONE',  ( -12.53282948625640003, 1378.856475634480148, 208.0411585582419889 ) ) ;
#61198=ADVANCED_FACE ( 'NONE', ( #78069 ), #110045, .T. ) ;
#61205=EDGE_CURVE ( 'NONE', #15055, #99409, #47251, .T. ) ;
#61207=CARTESIAN_POINT ( 'NONE',  ( -66.37942218196469923, 1384.673250244690053, 290.6307320938429939 ) ) ;
#61221=CARTESIAN_POINT ( 'NONE',  ( -106.4020496450190052, 1391.913060387289988, 304.2007955189830568 ) ) ;
#61226=CARTESIAN_POINT ( 'NONE',  ( -10.05179545849999911, 1382.519305957850065, 200.9245173917790055 ) ) ;
#61240=CARTESIAN_POINT ( 'NONE',  ( -59.50571812958200013, 1379.724539154309923, 264.8335893427189944 ) ) ;
#61246=CARTESIAN_POINT ( 'NONE',  ( -105.1577856459999936, 1379.115010806019882, 304.6242328078590162 ) ) ;
#61272=CARTESIAN_POINT ( 'NONE',  ( -51.28450536721118880, 1379.693347499785432, 242.1435806264775863 ) ) ;
#61299=CARTESIAN_POINT ( 'NONE',  ( -85.85832257059999506, 1385.179345198489955, 289.6849318678590066 ) ) ;
#61338=CARTESIAN_POINT ( 'NONE',  ( -21.76319146545460015, 1384.856752773889866, 221.7575919100939927 ) ) ;
#61352=DIRECTION ( 'NONE',  ( -1.000000000000000000, 0.000000000000000000, 0.000000000000000000 ) ) ;
#61359=CARTESIAN_POINT ( 'NONE',  ( -109.5441724340000036, 1378.991699893399982, 306.1169303483130193 ) ) ;
#61388=CARTESIAN_POINT ( 'NONE',  ( -64.85694393360000731, 1375.750462046670009, 269.1292758464589951 ) ) ;
#61389=CARTESIAN_POINT ( 'NONE',  ( -106.6345736060380034, 1378.913060387289988, 301.6740162769929725 ) ) ;
#61393=CARTESIAN_POINT ( 'NONE',  ( -94.50884446960000673, 1385.089621650810159, 294.8626808758589846 ) ) ;
#61394=CARTESIAN_POINT ( 'NONE',  ( -58.92658587845429707, 1384.666467992389926, 241.7252083246220025 ) ) ;
#61398=ORIENTED_EDGE ( 'NONE', *, *, #55850, .T. ) ;
#61404=CARTESIAN_POINT ( 'NONE',  ( -67.31912871069998516, 1379.744358027319777, 277.0891020787589696 ) ) ;
#61412=CARTESIAN_POINT ( 'NONE',  ( -43.09011427770000324, 1385.164419251190111, 247.5010251099589880 ) ) ;
#61414=CARTESIAN_POINT ( 'NONE',  ( -105.5185485394360114, 1378.942001926445982, 304.0419961266803170 ) ) ;
#61425=CARTESIAN_POINT ( 'NONE',  ( -5.663447254089540195, 1391.839989632750076, 215.0012937448320258 ) ) ;
#61433=DIRECTION ( 'NONE',  ( 1.402715769532790202E-14, -1.000000000000000000, 4.930380657631320281E-31 ) ) ;
#61457=CARTESIAN_POINT ( 'NONE',  ( -87.69898847370659212, 1383.771786689919963, 307.6789132609320063 ) ) ;
#61458=CARTESIAN_POINT ( 'NONE',  ( -109.7957506965259995, 1384.357922284569895, 311.3498508118249788 ) ) ;
#61464=CARTESIAN_POINT ( 'NONE',  ( -85.83179656309999928, 1383.342000450830028, 289.7170741207590368 ) ) ;
#61474=CARTESIAN_POINT ( 'NONE',  ( -108.5985451479999995, 1381.860774011350031, 297.8915311670589858 ) ) ;
#61545=CARTESIAN_POINT ( 'NONE',  ( -9.321299325100000033, 1391.019964971690115, 208.8523807111220094 ) ) ;
#61554=CARTESIAN_POINT ( 'NONE',  ( -9.448886036450000248, 1383.288095429739997, 218.3547579606889997 ) ) ;
#61557=VERTEX_POINT ( 'NONE', #108604 ) ;
#61580=CARTESIAN_POINT ( 'NONE',  ( -30.85555029051230136, 1383.840996389519887, 228.7204722429899846 ) ) ;
#61588=CARTESIAN_POINT ( 'NONE',  ( -1.112595545632909995E-15, 1378.856372334279968, 208.5307368469939888 ) ) ;
#61595=CARTESIAN_POINT ( 'NONE',  ( -12.29063289509999990, 1392.314904069939985, 209.7401570312620152 ) ) ;
#61602=CARTESIAN_POINT ( 'NONE',  ( -11.97267500829999953, 1391.195698933469885, 205.7774971565190185 ) ) ;
#61603=CARTESIAN_POINT ( 'NONE',  ( -91.57239150403411543, 1385.197581008679890, 293.4610811371219938 ) ) ;
#61605=CARTESIAN_POINT ( 'NONE',  ( -66.34652574609999931, 1379.749084393009980, 275.3210452576589660 ) ) ;
#61630=CARTESIAN_POINT ( 'NONE',  ( -68.77190087506669158, 1379.747925807530009, 280.3125204381590265 ) ) ;
#61643=CARTESIAN_POINT ( 'NONE',  ( -13.24974103930710001, 1379.480115360689979, 208.4658629847600082 ) ) ;
#61662=AXIS2_PLACEMENT_3D ( 'NONE', #88119, #3573, #29292 ) ;
#61686=CARTESIAN_POINT ( 'NONE',  ( -109.8861939232002243, 1383.682673601628721, 297.0706783926800654 ) ) ;
#61689=CARTESIAN_POINT ( 'NONE',  ( -44.12060424749999754, 1379.737242085850085, 229.5711980135589840 ) ) ;
#61693=CARTESIAN_POINT ( 'NONE',  ( -68.70081072619076679, 1379.747840807290004, 280.2881824009641605 ) ) ;
#61725=CARTESIAN_POINT ( 'NONE',  ( -13.78554130023140090, 1379.661829793600191, 208.1182657059560199 ) ) ;
#61732=CARTESIAN_POINT ( 'NONE',  ( -7.594207177912499773, 1384.073165582419961, 219.0227910255269990 ) ) ;
#61745=CARTESIAN_POINT ( 'NONE',  ( -62.29576501915909859, 1384.687103135880079, 284.7157575292210367 ) ) ;
#61746=CARTESIAN_POINT ( 'NONE',  ( -10.29144330875089963, 1384.933285862410003, 200.0364846665950154 ) ) ;
#61750=CARTESIAN_POINT ( 'NONE',  ( -105.7942887633819993, 1378.913060387289988, 304.0474587704230203 ) ) ;
#61752=CARTESIAN_POINT ( 'NONE',  ( -7.965680540240001051, 1384.926148861439970, 199.4891222871690104 ) ) ;
#61764=CARTESIAN_POINT ( 'NONE',  ( -10.63394288230000129, 1381.391042983399984, 201.9860236516190071 ) ) ;
#61778=CARTESIAN_POINT ( 'NONE',  ( -66.39208760710349111, 1379.743175614790061, 277.0517417713629698 ) ) ;
#61793=CARTESIAN_POINT ( 'NONE',  ( -105.8748966381740075, 1378.913060387980067, 304.8767970569450085 ) ) ;
#61810=CARTESIAN_POINT ( 'NONE',  ( -8.297448150139999257, 1384.938007610199747, 218.7034661405789961 ) ) ;
#61813=CARTESIAN_POINT ( 'NONE',  ( -12.63540103640000112, 1379.206155667370012, 208.6368498725950076 ) ) ;
#61814=CARTESIAN_POINT ( 'NONE',  ( -32.26928162443899595, 1379.633198882570241, 215.6001090146092167 ) ) ;
#61825=CARTESIAN_POINT ( 'NONE',  ( -46.82073828382691971, 1379.680985121969115, 239.8219845903596195 ) ) ;
#61846=CARTESIAN_POINT ( 'NONE',  ( -86.93140579660001777, 1384.976593077780080, 307.7302223600589741 ) ) ;
#61857=CARTESIAN_POINT ( 'NONE',  ( -105.1077133852530068, 1379.453477749980038, 305.4638311486609723 ) ) ;
#61885=CARTESIAN_POINT ( 'NONE',  ( -13.66835502576310013, 1384.880622718460017, 219.1890757919979933 ) ) ;
#61891=EDGE_CURVE ( 'NONE', #103208, #62022, #103335, .T. ) ;
#61903=CARTESIAN_POINT ( 'NONE',  ( -109.9718049258029993, 1384.472301579249915, 311.4373116341799914 ) ) ;
#61944=CARTESIAN_POINT ( 'NONE',  ( -85.54616801939999959, 1378.671092583530026, 296.2627734746589567 ) ) ;
#61945=CARTESIAN_POINT ( 'NONE',  ( -105.7942887633819993, 1378.913060387289988, 304.0474587704230203 ) ) ;
#61949=CARTESIAN_POINT ( 'NONE',  ( -103.7379679780000004, 1385.000870667160143, 296.9192581611590072 ) ) ;
#61957=CARTESIAN_POINT ( 'NONE',  ( -13.37005892530000040, 1384.196513454120122, 218.9076047076389955 ) ) ;
#61962=CARTESIAN_POINT ( 'NONE',  ( -67.68830324459999304, 1379.745299480660151, 277.8290332001590173 ) ) ;
#61970=CARTESIAN_POINT ( 'NONE',  ( -36.11306192460000375, 1385.070985855290019, 235.4717389730590185 ) ) ;
#61981=CARTESIAN_POINT ( 'NONE',  ( -5.930127944598639900, 1391.913057044489960, 215.1135602292339968 ) ) ;
#62013=CARTESIAN_POINT ( 'NONE',  ( -92.10450461559780422, 1383.768992061189920, 309.1587668656890173 ) ) ;
#62014=CARTESIAN_POINT ( 'NONE',  ( -109.6411560373970104, 1384.508416019190008, 311.3033268927259769 ) ) ;
#62020=CARTESIAN_POINT ( 'NONE',  ( -90.19765245659999664, 1379.339186696669913, 300.1519328718590032 ) ) ;
#62022=VERTEX_POINT ( 'NONE', #44593 ) ;
#62049=CARTESIAN_POINT ( 'NONE',  ( -110.0629084955440078, 1384.909053975289908, 296.9513011978259556 ) ) ;
#62060=ORIENTED_EDGE ( 'NONE', *, *, #35246, .T. ) ;
#62066=EDGE_CURVE ( 'NONE', #82950, #73589, #41969, .T. ) ;
#62104=CARTESIAN_POINT ( 'NONE',  ( -19.18216750550000071, 1385.279599344249846, 220.5028985859590023 ) ) ;
#62113=CARTESIAN_POINT ( 'NONE',  ( -10.04451165320000072, 1380.536316001939895, 216.6372458847690154 ) ) ;
#62128=CARTESIAN_POINT ( 'NONE',  ( -109.5279943120000041, 1385.221486439480032, 297.1347434786590043 ) ) ;
#62141=CARTESIAN_POINT ( 'NONE',  ( -32.29029968710140253, 1383.839140599110124, 230.3723284232519859 ) ) ;
#62149=CARTESIAN_POINT ( 'NONE',  ( -10.04827894765687724, 1389.656101278125107, 201.8970266557225557 ) ) ;
#62164=CARTESIAN_POINT ( 'NONE',  ( -88.49990301145820126, 1385.187970965449949, 291.5961977735890400 ) ) ;
#62166=CARTESIAN_POINT ( 'NONE',  ( -21.25567046294848694, 1379.716576505264129, 209.8535136764940887 ) ) ;
#62185=CIRCLE ( 'NONE', #90761, 12.34219900309999929 ) ;
#62189=CARTESIAN_POINT ( 'NONE',  ( -68.77190087506669158, 1379.747925807530009, 280.3125204381590265 ) ) ;
#62218=AXIS2_PLACEMENT_3D ( 'NONE', #9151, #43315, #19171 ) ;
#62239=CARTESIAN_POINT ( 'NONE',  ( -109.7763673550909544, 1383.370472583167611, 297.1349124586991479 ) ) ;
#62241=CARTESIAN_POINT ( 'NONE',  ( -26.09133589079999993, 1379.618104246070061, 211.3566207186690065 ) ) ;
#62252=CARTESIAN_POINT ( 'NONE',  ( -66.37566924875659424, 1385.037721167210066, 290.6307433382449972 ) ) ;
#62277=CARTESIAN_POINT ( 'NONE',  ( -12.26530734194249916, 1377.620920188950095, 208.0499041502589819 ) ) ;
#62289=DIRECTION ( 'NONE',  ( -1.000000000000000000, 0.000000000000000000, 0.000000000000000000 ) ) ;
#62301=CARTESIAN_POINT ( 'NONE',  ( -105.2189605138059960, 1384.590928737530021, 311.1873984220050033 ) ) ;
#62302=CARTESIAN_POINT ( 'NONE',  ( -44.08363024569199951, 1385.000492669140158, 217.2190647443480032 ) ) ;
#62311=CARTESIAN_POINT ( 'NONE',  ( -8.604279045229999312, 1384.934799959460179, 199.8686450314289971 ) ) ;
#62318=CARTESIAN_POINT ( 'NONE',  ( -107.2902847454959954, 1391.913060387289988, 307.3027153792770036 ) ) ;
#62334=CARTESIAN_POINT ( 'NONE',  ( -60.26586262799999361, 1379.746226298030024, 265.9249327376589918 ) ) ;
#62346=CARTESIAN_POINT ( 'NONE',  ( -105.8136274632349938, 1378.913060387269979, 304.5029232650449558 ) ) ;
#62348=EDGE_CURVE ( 'NONE', #61054, #26950, #101460, .T. ) ;
#62355=CARTESIAN_POINT ( 'NONE',  ( -5.013264346206871558, 1375.415296214948967, 203.5257471534737874 ) ) ;
#62362=CARTESIAN_POINT ( 'NONE',  ( -8.861951559199999551, 1384.939357637759940, 218.6849988088989960 ) ) ;
#62365=CARTESIAN_POINT ( 'NONE',  ( -49.10452650019272625, 1379.685310564211932, 237.8554457964596338 ) ) ;
#62376=CARTESIAN_POINT ( 'NONE',  ( -46.87897873459490938, 1379.681191137500036, 239.9263311024370751 ) ) ;
#62382=DIRECTION ( 'NONE',  ( -4.481801771516530428E-20, -1.000000000000000000, -2.868959329816139585E-18 ) ) ;
#62397=CARTESIAN_POINT ( 'NONE',  ( -83.92017472829999747, 1389.470547577029947, 291.9741855502589942 ) ) ;
#62408=CARTESIAN_POINT ( 'NONE',  ( -105.9895980336749943, 1381.595986325180093, 309.4771618232359742 ) ) ;
#62438=CARTESIAN_POINT ( 'NONE',  ( -21.26129628348120448, 1384.858351126920070, 221.5120817745969930 ) ) ;
#62466=CARTESIAN_POINT ( 'NONE',  ( -84.31100485922900134, 1379.600296255510102, 298.0934801170350283 ) ) ;
#62478=CARTESIAN_POINT ( 'NONE',  ( -8.205450199690000446, 1383.672729848519793, 218.6026122865090144 ) ) ;
#62502=CARTESIAN_POINT ( 'NONE',  ( -88.45813511300001153, 1378.648767874889927, 298.0129420291590350 ) ) ;
#62504=CARTESIAN_POINT ( 'NONE',  ( -105.8009562800430103, 1378.913060387269979, 303.8747423308259386 ) ) ;
#62507=CARTESIAN_POINT ( 'NONE',  ( -106.7756681350000036, 1384.894991215109940, 297.1173194602590115 ) ) ;
#62514=CARTESIAN_POINT ( 'NONE',  ( -1.252324120818309726E-15, 1383.870885931430166, 218.4497379877689980 ) ) ;
#62520=CARTESIAN_POINT ( 'NONE',  ( -66.64551715449999847, 1379.743402054680018, 275.6922576809590169 ) ) ;
#62529=CARTESIAN_POINT ( 'NONE',  ( -38.50281909529999780, 1385.190821792449924, 239.3058332809590070 ) ) ;
#62531=CARTESIAN_POINT ( 'NONE',  ( -35.04101985798630636, 1385.208921701160079, 234.2276399419079951 ) ) ;
#62554=UNCERTAINTY_MEASURE_WITH_UNIT (LENGTH_MEASURE( 1.000000000000000082E-05 ), #41521, 'distance_accuracy_value', 'NONE');
#62557=FACE_OUTER_BOUND ( 'NONE', #30613, .T. ) ;
#62584=CARTESIAN_POINT ( 'NONE',  ( -85.31977994509040286, 1383.773333636219832, 306.6464895601730518 ) ) ;
#62585=CARTESIAN_POINT ( 'NONE',  ( -109.6626209149679880, 1383.298351538420093, 311.2476010510089850 ) ) ;
#62591=CARTESIAN_POINT ( 'NONE',  ( -94.49938873620000379, 1383.385654720950015, 294.8908487859590082 ) ) ;
#62596=CARTESIAN_POINT ( 'NONE',  ( -109.7177239279999981, 1384.918725008840056, 297.0861730621589913 ) ) ;
#62627=AXIS2_PLACEMENT_3D ( 'NONE', #18766, #362, #34488 ) ;
#62628=EDGE_LOOP ( 'NONE', ( #92608, #4492, #89698, #89401 ) ) ;
#62637=CARTESIAN_POINT ( 'NONE',  ( 10.22326110114815201, 1374.913060387290216, 204.3929701860967896 ) ) ;
#62669=CARTESIAN_POINT ( 'NONE',  ( -24.59348072959999953, 1389.777865159989915, 218.7886947571089991 ) ) ;
#62697=ADVANCED_FACE ( 'NONE', ( #59759 ), #45601, .T. ) ;
#62711=CARTESIAN_POINT ( 'NONE',  ( -18.28047778769730058, 1383.855358566239829, 220.1279645894470036 ) ) ;
#62719=CARTESIAN_POINT ( 'NONE',  ( -3.078458295609999951, 1382.319662484240098, 217.8852017108989969 ) ) ;
#62725=CARTESIAN_POINT ( 'NONE',  ( -11.99567239095710036, 1390.320064639609882, 213.8405493935750030 ) ) ;
#62733=CARTESIAN_POINT ( 'NONE',  ( -7.965935579988510540, 1384.902014119069918, 199.4892638029120064 ) ) ;
#62734=CARTESIAN_POINT ( 'NONE',  ( -89.28323898676370618, 1385.190482965020010, 292.1241280709670036 ) ) ;
#62767=DIRECTION ( 'NONE',  ( -0.02617694830785676288, 0.9996573249755578150, 1.483054601246242193E-17 ) ) ;
#62794=AXIS2_PLACEMENT_3D ( 'NONE', #50643, #84772, #8070 ) ;
#62798=EDGE_LOOP ( 'NONE', ( #55338, #96837 ) ) ;
#62823=CARTESIAN_POINT ( 'NONE',  ( -66.03229317983959845, 1385.039105777579834, 290.1674623452569790 ) ) ;
#62852=CARTESIAN_POINT ( 'NONE',  ( -12.30462497340020001, 1377.683743082049887, 208.6098874196279951 ) ) ;
#62875=CARTESIAN_POINT ( 'NONE',  ( -84.46369479308390282, 1384.629619117830089, 306.4275599946969919 ) ) ;
#62876=CARTESIAN_POINT ( 'NONE',  ( -48.75929104102600320, 1385.014805441129965, 223.3784622248080041 ) ) ;
#62878=CARTESIAN_POINT ( 'NONE',  ( -5.069242052572500157, 1375.174993499499806, 214.7429053951260016 ) ) ;
#62896=CARTESIAN_POINT ( 'NONE',  ( -11.17264282910000084, 1380.903189564030072, 202.7795052211189955 ) ) ;
#62908=CARTESIAN_POINT ( 'NONE',  ( -67.98270077001589584, 1379.746359850080125, 279.4236968873279920 ) ) ;
#62937=VECTOR ( 'NONE', #44347, 1000.000000000000000 ) ;
#62939=CARTESIAN_POINT ( 'NONE',  ( -66.35507711686996402, 1379.742713900610170, 275.1017064096059812 ) ) ;
#62950=CARTESIAN_POINT ( 'NONE',  ( -63.28909092007827297, 1379.735398356163614, 271.9840329659873532 ) ) ;
#62966=CARTESIAN_POINT ( 'NONE',  ( -9.239806556520379743, 1384.978503770619909, 197.9483252412619834 ) ) ;
#62979=CARTESIAN_POINT ( 'NONE',  ( -106.7799791470000059, 1379.928168464490000, 308.6026344867590296 ) ) ;
#63005=CARTESIAN_POINT ( 'NONE',  ( -35.75806911936049914, 1384.805942682020031, 235.2916753997550074 ) ) ;
#63021=CARTESIAN_POINT ( 'NONE',  ( 3.550311703873260096E-15, 1384.899971913130003, 209.1218459572589836 ) ) ;
#63023=ADVANCED_FACE ( 'NONE', ( #36036 ), #24181, .F. ) ;
#63029=CARTESIAN_POINT ( 'NONE',  ( -48.44397510641989868, 1379.564747003970069, 243.3357836602579880 ) ) ;
#63038=CARTESIAN_POINT ( 'NONE',  ( -7.543596773550000023, 1384.566397051120020, 219.0776135590490128 ) ) ;
#63059=CARTESIAN_POINT ( 'NONE',  ( -94.55573068399999670, 1379.531630663989972, 302.1084921616590009 ) ) ;
#63067=CARTESIAN_POINT ( 'NONE',  ( -92.78054746879999470, 1385.201317530089909, 294.1545524748589742 ) ) ;
#63079=CARTESIAN_POINT ( 'NONE',  ( -67.45763281530000199, 1379.744713633030187, 277.3665591780590489 ) ) ;
#63088=CARTESIAN_POINT ( 'NONE',  ( -86.93521348900000589, 1384.624802884190103, 307.7215772890590415 ) ) ;
#63090=CARTESIAN_POINT ( 'NONE',  ( -30.83205449964789935, 1385.229680719480029, 228.9263574028450137 ) ) ;
#63102=ORIENTED_EDGE ( 'NONE', *, *, #8801, .F. ) ;
#63120=CARTESIAN_POINT ( 'NONE',  ( -103.8895706480000030, 1379.883984609199842, 304.0050191322589512 ) ) ;
#63133=CARTESIAN_POINT ( 'NONE',  ( -82.29609599402139963, 1383.775366892559987, 305.0689505943109907 ) ) ;
#63134=CARTESIAN_POINT ( 'NONE',  ( -109.4509034362719859, 1384.431620334350100, 311.2553551991560425 ) ) ;
#63138=CARTESIAN_POINT ( 'NONE',  ( -106.6204612740000073, 1379.399477473190018, 303.3336452769589755 ) ) ;
#63143=CARTESIAN_POINT ( 'NONE',  ( -109.3492103629999974, 1384.912544404370237, 297.1385189228590207 ) ) ;
#63216=CARTESIAN_POINT ( 'NONE',  ( -30.11988021650000036, 1389.744009244819836, 222.9251520012589936 ) ) ;
#63241=CARTESIAN_POINT ( 'NONE',  ( -109.5349736409999934, 1385.152114132390125, 297.1296876067589778 ) ) ;
#63251=CARTESIAN_POINT ( 'NONE',  ( -24.20210390755639907, 1383.848986423020051, 222.9592914590000134 ) ) ;
#63259=CARTESIAN_POINT ( 'NONE',  ( -11.15738487964140013, 1390.939238811560017, 203.8452351040699853 ) ) ;
#63265=CARTESIAN_POINT ( 'NONE',  ( -13.55712941462900112, 1390.145928966170004, 212.6894278554629807 ) ) ;
#63273=CARTESIAN_POINT ( 'NONE',  ( -7.966180769845361276, 1384.913883566769982, 199.4893105002079778 ) ) ;
#63274=CARTESIAN_POINT ( 'NONE',  ( -106.3772841639279960, 1385.236231160509988, 297.0206994190789942 ) ) ;
#63279=ORIENTED_EDGE ( 'NONE', *, *, #56195, .F. ) ;
#63292=CARTESIAN_POINT ( 'NONE',  ( -14.28742066159479940, 1392.367256947369924, 209.8406639845640029 ) ) ;
#63323=EDGE_CURVE ( 'NONE', #52311, #108404, #104184, .T. ) ;
#63350=CARTESIAN_POINT ( 'NONE',  ( -106.1610222967859869, 1391.913060319860051, 304.8404902532309961 ) ) ;
#63351=CARTESIAN_POINT ( 'NONE',  ( -67.37805264042475528, 1379.747543260372140, 278.5100200681151819 ) ) ;
#63359=CARTESIAN_POINT ( 'NONE',  ( -104.5692869006220036, 1384.935441801240131, 311.1781066240710061 ) ) ;
#63361=CARTESIAN_POINT ( 'NONE',  ( -8.888257569051779328, 1385.312153913200063, 218.6608301139260107 ) ) ;
#63365=DIRECTION ( 'NONE',  ( -1.000000000000000000, 0.000000000000000000, 0.000000000000000000 ) ) ;
#63386=CARTESIAN_POINT ( 'NONE',  ( -12.55407686808170098, 1378.884881417289989, 208.1735791207040052 ) ) ;
#63410=CARTESIAN_POINT ( 'NONE',  ( -41.29992742285089946, 1384.993104148180009, 214.1677007736450093 ) ) ;
#63417=CARTESIAN_POINT ( 'NONE',  ( -109.6576113679999906, 1384.901204824579963, 311.3230521602589533 ) ) ;
#63423=CARTESIAN_POINT ( 'NONE',  ( -107.1288397327830069, 1391.913060387289988, 306.9725994467550549 ) ) ;
#63427=CARTESIAN_POINT ( 'NONE',  ( -12.17490798859999934, 1378.378576834209980, 206.9930340770689838 ) ) ;
#63440=CARTESIAN_POINT ( 'NONE',  ( -67.37805264080000711, 1379.747543260419889, 278.5100200678590454 ) ) ;
#63451=CARTESIAN_POINT ( 'NONE',  ( -105.8048160525020052, 1378.913060387249971, 304.4117408737909614 ) ) ;
#63457=FACE_OUTER_BOUND ( 'NONE', #8067, .T. ) ;
#63470=CARTESIAN_POINT ( 'NONE',  ( -14.28029386204369899, 1390.367275669339961, 209.8449220790990069 ) ) ;
#63471=CARTESIAN_POINT ( 'NONE',  ( -67.48208812431644787, 1379.745290141752776, 277.3802860916713371 ) ) ;
#63476=CARTESIAN_POINT ( 'NONE',  ( -49.39991366742589918, 1384.617024020139752, 224.3629336449129994 ) ) ;
#63506=CARTESIAN_POINT ( 'NONE',  ( -113.4000000000000057, 1386.785055403669958, 297.3836343121590176 ) ) ;
#63519=CARTESIAN_POINT ( 'NONE',  ( -104.7786280602689999, 1380.751497738820035, 308.1052390028799550 ) ) ;
#63542=CARTESIAN_POINT ( 'NONE',  ( -41.12117611683139273, 1384.782461838570043, 244.1305867940789938 ) ) ;
#63553=AXIS2_PLACEMENT_3D ( 'NONE', #71717, #10103, #1175 ) ;
#63564=CARTESIAN_POINT ( 'NONE',  ( -42.03938205346800316, 1377.690944531520017, 233.5611963710439909 ) ) ;
#63566=CARTESIAN_POINT ( 'NONE',  ( -16.66186295847979792, 1379.591909316719921, 212.1494488913359930 ) ) ;
#63573=CARTESIAN_POINT ( 'NONE',  ( -7.553780601869999778, 1384.400324961100068, 219.0644599357090101 ) ) ;
#63592=CARTESIAN_POINT ( 'NONE',  ( -14.34382872122290031, 1380.323822069550033, 209.7285467014039853 ) ) ;
#63595=CARTESIAN_POINT ( 'NONE',  ( -70.04184978290001595, 1379.439320607440095, 279.7464857826589650 ) ) ;
#63614=CARTESIAN_POINT ( 'NONE',  ( -68.00907612829999493, 1379.746097695369826, 278.4774409410590010 ) ) ;
#63624=CARTESIAN_POINT ( 'NONE',  ( -86.93140579660001777, 1384.976593077780080, 307.7302223600589741 ) ) ;
#63626=CARTESIAN_POINT ( 'NONE',  ( -30.52320602891570189, 1385.231135277879957, 228.5881811678719941 ) ) ;
#63670=CARTESIAN_POINT ( 'NONE',  ( -109.7600093021320049, 1383.545064258730008, 311.3057984900200381 ) ) ;
#63674=CARTESIAN_POINT ( 'NONE',  ( -113.4000000000000057, 1380.131807193299892, 307.5349059445590001 ) ) ;
#63680=CARTESIAN_POINT ( 'NONE',  ( -109.5347831020000058, 1384.920243598159914, 297.1230830264590281 ) ) ;
#63692=CARTESIAN_POINT ( 'NONE',  ( -113.4000000000000057, 1379.913060387289988, 304.2218459572590064 ) ) ;
#63725=CARTESIAN_POINT ( 'NONE',  ( -26.13451554100480223, 1384.547168729040095, 203.7448848093029881 ) ) ;
#63769=CARTESIAN_POINT ( 'NONE',  ( -12.31060128686659993, 1378.376182493429951, 209.7919535259509871 ) ) ;
#63783=CARTESIAN_POINT ( 'NONE',  ( -30.38379501695840190, 1383.841595863670136, 228.2076059929920007 ) ) ;
#63794=CARTESIAN_POINT ( 'NONE',  ( -9.770253401179999742, 1381.414343185820144, 201.2605876295190228 ) ) ;
#63801=CARTESIAN_POINT ( 'NONE',  ( -10.62909775710000027, 1390.234991692080030, 215.5537828994590086 ) ) ;
#63802=CARTESIAN_POINT ( 'NONE',  ( -10.25401551478790196, 1391.808998814714187, 215.0731684536954731 ) ) ;
#63809=CARTESIAN_POINT ( 'NONE',  ( -7.966081143649218710, 1384.918389534460175, 199.4892681243580057 ) ) ;
#63810=CARTESIAN_POINT ( 'NONE',  ( -94.44233799117999695, 1385.205980051620145, 294.7441417489620221 ) ) ;
#63811=CARTESIAN_POINT ( 'NONE',  ( -113.4000000000000057, 1390.939237335599955, 304.2218459572590064 ) ) ;
#63815=CARTESIAN_POINT ( 'NONE',  ( -120.0391016774570403, 1390.913060387289988, 305.8779575274093077 ) ) ;
#63836=CARTESIAN_POINT ( 'NONE',  ( -7.544890296849999345, 1384.926148866459926, 219.0875903968589853 ) ) ;
#63867=CARTESIAN_POINT ( 'NONE',  ( -113.3174119514818301, 1391.913060387289988, 300.7228204909004603 ) ) ;
#63888=CARTESIAN_POINT ( 'NONE',  ( -106.4421323744290078, 1391.913060418769874, 306.1278572653080232 ) ) ;
#63897=CARTESIAN_POINT ( 'NONE',  ( -89.21014235648939916, 1384.971367781859726, 308.4434907503709837 ) ) ;
#63903=CARTESIAN_POINT ( 'NONE',  ( -7.544898852049939819, 1384.902875181250010, 219.0876726591300212 ) ) ;
#63948=CARTESIAN_POINT ( 'NONE',  ( -94.97055395160710134, 1384.610110349949991, 310.0293933350179714 ) ) ;
#63949=CARTESIAN_POINT ( 'NONE',  ( -31.13530430868299703, 1384.970948276150011, 206.1966052560059950 ) ) ;
#63957=CARTESIAN_POINT ( 'NONE',  ( -109.3075498650000128, 1384.894860980859903, 311.2646804682590300 ) ) ;
#63967=CARTESIAN_POINT ( 'NONE',  ( -10.44371214979999962, 1379.699184266919929, 202.4842574811590055 ) ) ;
#63982=CARTESIAN_POINT ( 'NONE',  ( -68.18659372557320353, 1379.747119388199735, 279.6866116612499695 ) ) ;
#63986=ORIENTED_EDGE ( 'NONE', *, *, #58492, .F. ) ;
#63993=CARTESIAN_POINT ( 'NONE',  ( -105.8258850450579871, 1378.913060387369796, 304.5940478994550062 ) ) ;
#64009=CARTESIAN_POINT ( 'NONE',  ( -8.862296812249999434, 1384.904551176430004, 218.6851794592490137 ) ) ;
#64011=CARTESIAN_POINT ( 'NONE',  ( -65.90777676982870048, 1379.741637275925996, 274.1881090155197285 ) ) ;
#64015=CARTESIAN_POINT ( 'NONE',  ( -51.92850933155389725, 1384.628554692669923, 228.3932471100619921 ) ) ;
#64065=DIRECTION ( 'NONE',  ( -1.000000000000000000, 1.836970198721029688E-16, 0.000000000000000000 ) ) ;
#64079=CARTESIAN_POINT ( 'NONE',  ( -38.22024519373950113, 1384.795465018370123, 239.1128382243029762 ) ) ;
#64082=CARTESIAN_POINT ( 'NONE',  ( -105.2848455000000030, 1379.129118594349848, 302.8293157935589761 ) ) ;
#64102=CARTESIAN_POINT ( 'NONE',  ( -69.50772043394130151, 1378.360807531410046, 286.6555711028250357 ) ) ;
#64105=FACE_OUTER_BOUND ( 'NONE', #47728, .T. ) ;
#64109=CYLINDRICAL_SURFACE ( 'NONE', #99956, 2.500000000000001776 ) ;
#64114=CARTESIAN_POINT ( 'NONE',  ( -8.697719184660000380, 1384.095450953160025, 218.5750472044589969 ) ) ;
#64136=CARTESIAN_POINT ( 'NONE',  ( -14.48029645964409973, 1380.025135367679923, 208.7108227440779729 ) ) ;
#64141=CARTESIAN_POINT ( 'NONE',  ( -44.32302097390000029, 1380.083786706710043, 232.1686497034590104 ) ) ;
#64154=CARTESIAN_POINT ( 'NONE',  ( -25.94071553730000090, 1384.508713631559885, 224.2416845492589914 ) ) ;
#64159=CARTESIAN_POINT ( 'NONE',  ( -62.95758008990000576, 1379.733836041129962, 267.9697104864590074 ) ) ;
#64167=CARTESIAN_POINT ( 'NONE',  ( -76.09690353929998707, 1385.004314140359838, 301.2232021421590389 ) ) ;
#64169=CARTESIAN_POINT ( 'NONE',  ( -21.27099332670459830, 1385.271245282970085, 221.4929286867449889 ) ) ;
#64192=CARTESIAN_POINT ( 'NONE',  ( -105.7922211859999919, 1391.737185282639985, 301.9078056316589596 ) ) ;
#64194=CARTESIAN_POINT ( 'NONE',  ( -107.4307047400000101, 1391.913060387289988, 300.8770155100590387 ) ) ;
#64217=CARTESIAN_POINT ( 'NONE',  ( -96.36158319419999430, 1382.338469500439942, 309.9311367202590191 ) ) ;
#64224=CARTESIAN_POINT ( 'NONE',  ( -9.082617507235918097, 1381.499571894695009, 200.6641547696254975 ) ) ;
#64335=CARTESIAN_POINT ( 'NONE',  ( -37.50821108740120025, 1383.831899505290039, 237.6397739250450059 ) ) ;
#64341=ORIENTED_EDGE ( 'NONE', *, *, #5942, .F. ) ;
#64345=CARTESIAN_POINT ( 'NONE',  ( -23.02925477460000181, 1382.322973038800001, 221.4483044241590335 ) ) ;
#64351=CARTESIAN_POINT ( 'NONE',  ( -11.13127190274779998, 1388.613762639859942, 216.5227499701169620 ) ) ;
#64373=CARTESIAN_POINT ( 'NONE',  ( -109.5779934659999952, 1386.007389322860035, 311.2464976022590122 ) ) ;
#64385=CARTESIAN_POINT ( 'NONE',  ( -8.579591590190000616, 1385.064761779769924, 218.6660937052890006 ) ) ;
#64405=CARTESIAN_POINT ( 'NONE',  ( -6.354406034210000165, 1384.502204350209922, 199.7451528500290010 ) ) ;
#64413=EDGE_CURVE ( 'NONE', #94821, #33676, #50768, .T. ) ;
#64440=CARTESIAN_POINT ( 'NONE',  ( -106.4410097957560026, 1391.810857979010052, 306.8924406162939817 ) ) ;
#64448=CARTESIAN_POINT ( 'NONE',  ( -83.69811532344560590, 1384.984538349280001, 306.0467535211649874 ) ) ;
#64449=CARTESIAN_POINT ( 'NONE',  ( -8.959619814139999860, 1385.213185382589927, 199.9358950396990053 ) ) ;
#64463=CARTESIAN_POINT ( 'NONE',  ( -110.0191722785379653, 1385.664243115142426, 296.9929505227199797 ) ) ;
#64496=CARTESIAN_POINT ( 'NONE',  ( -12.32169722289999925, 1378.992744615490210, 209.8847561567199875 ) ) ;
#64497=CARTESIAN_POINT ( 'NONE',  ( -84.84750775523609434, 1384.628878466070091, 306.6159466445730004 ) ) ;
#64498=CARTESIAN_POINT ( 'NONE',  ( -60.37232013571600220, 1385.063171825080190, 244.7907910518410119 ) ) ;
#64529=CARTESIAN_POINT ( 'NONE',  ( -68.38904811079750345, 1379.747152134330008, 279.9588836171899970 ) ) ;
#64559=CARTESIAN_POINT ( 'NONE',  ( -68.80955101979490962, 1379.748017775673134, 280.2796398541619851 ) ) ;
#64564=CARTESIAN_POINT ( 'NONE',  ( -61.65199887796450895, 1384.683307422990083, 247.6074881643829997 ) ) ;
#64594=CARTESIAN_POINT ( 'NONE',  ( -109.9987473180000137, 1385.244513981200043, 297.1847073398589600 ) ) ;
#64600=CARTESIAN_POINT ( 'NONE',  ( -109.7277482404900013, 1383.460710247889892, 311.2865699025030040 ) ) ;
#64630=CARTESIAN_POINT ( 'NONE',  ( -41.84381950253869320, 1384.779123927429964, 245.4572242766560066 ) ) ;
#64656=CARTESIAN_POINT ( 'NONE',  ( -87.43044411833730578, 1379.577971547200150, 299.9734229985630236 ) ) ;
#64669=FACE_OUTER_BOUND ( 'NONE', #73042, .T. ) ;
#64690=CARTESIAN_POINT ( 'NONE',  ( -12.33449316102499971, 1378.995504077259966, 209.6450772243929919 ) ) ;
#64694=CARTESIAN_POINT ( 'NONE',  ( -59.28197579180000076, 1379.588121118040135, 258.5658342392590043 ) ) ;
#64709=CARTESIAN_POINT ( 'NONE',  ( -43.09053402079999984, 1384.454438790149879, 247.5006848784589977 ) ) ;
#64715=CARTESIAN_POINT ( 'NONE',  ( -50.84608916490000041, 1379.691708908819919, 241.2101448141589799 ) ) ;
#64726=CARTESIAN_POINT ( 'NONE',  ( -24.60516260371240094, 1385.257503092070010, 223.4099358821769954 ) ) ;
#64755=CARTESIAN_POINT ( 'NONE',  ( -106.8894869739999933, 1388.082512067059952, 298.5417979983590158 ) ) ;
#64757=CARTESIAN_POINT ( 'NONE',  ( -107.0467961469999949, 1391.913060387289988, 301.5621515082589781 ) ) ;
#64759=DIRECTION ( 'NONE',  ( -0.002969046283321036261, 0.3161973579630307785, -0.9486887875280103355 ) ) ;
#64761=CARTESIAN_POINT ( 'NONE',  ( -103.8942762430000073, 1379.883600127840054, 303.6250335555589572 ) ) ;
#64763=DIRECTION ( 'NONE',  ( -1.000000000000000000, 0.000000000000000000, 0.000000000000000000 ) ) ;
#64773=CARTESIAN_POINT ( 'NONE',  ( -103.2908355774439997, 1383.761877798790010, 310.9219936770090271 ) ) ;
#64778=CARTESIAN_POINT ( 'NONE',  ( -109.9987473030000018, 1379.411466190030069, 303.3266014941589788 ) ) ;
#64784=CARTESIAN_POINT ( 'NONE',  ( -10.60205606837675951, 1379.520036171940774, 202.7691692326841633 ) ) ;
#64832=CARTESIAN_POINT ( 'NONE',  ( -20.28517678552929837, 1384.534033518609931, 201.7562538433300006 ) ) ;
#64843=CARTESIAN_POINT ( 'NONE',  ( -68.77190080519999071, 1379.747925807450201, 280.3125203366930123 ) ) ;
#64867=ORIENTED_EDGE ( 'NONE', *, *, #8801, .T. ) ;
#64880=CARTESIAN_POINT ( 'NONE',  ( -109.5358681720000078, 1384.943159170210265, 297.1231916241590056 ) ) ;
#64882=ORIENTED_EDGE ( 'NONE', *, *, #56465, .T. ) ;
#64891=CARTESIAN_POINT ( 'NONE',  ( -53.07794406699930079, 1383.806925713539840, 267.6250404484239880 ) ) ;
#64899=CARTESIAN_POINT ( 'NONE',  ( -26.36437929639999922, 1382.323664421269996, 223.7125964019590185 ) ) ;
#64905=CARTESIAN_POINT ( 'NONE',  ( -12.25820234982129975, 1388.996037939079997, 215.8687775299890177 ) ) ;
#64924=CARTESIAN_POINT ( 'NONE',  ( -108.7465780080000002, 1386.162170843670083, 311.0556125892589421 ) ) ;
#64928=CARTESIAN_POINT ( 'NONE',  ( -5.432410439472700858, 1391.426148861440197, 203.3415300314919989 ) ) ;
#64933=CARTESIAN_POINT ( 'NONE',  ( -8.881957496880000136, 1385.278510013270079, 218.6647829999089936 ) ) ;
#64948=CARTESIAN_POINT ( 'NONE',  ( -108.1636966620979905, 1378.913060387289988, 299.7761360902010210 ) ) ;
#64988=CARTESIAN_POINT ( 'NONE',  ( -98.46611804737121076, 1384.949949166809802, 310.6468918634429883 ) ) ;
#64989=CARTESIAN_POINT ( 'NONE',  ( -7.988067379700000359, 1385.733169288700083, 199.5350710154689864 ) ) ;
#65009=CARTESIAN_POINT ( 'NONE',  ( -12.54019733330000008, 1391.397793261360221, 209.7548870936209937 ) ) ;
#65030=CARTESIAN_POINT ( 'NONE',  ( -12.28044260189999903, 1378.789922127170030, 210.3771987704189996 ) ) ;
#65032=CARTESIAN_POINT ( 'NONE',  ( -56.65180216886200526, 1385.045677901099907, 237.0459369986420199 ) ) ;
#65040=CARTESIAN_POINT ( 'NONE',  ( -109.8254909340000012, 1384.904097876479909, 311.3807978792589779 ) ) ;
#65045=CARTESIAN_POINT ( 'NONE',  ( -109.1111606190000032, 1384.583257063580049, 311.2497810012590094 ) ) ;
#65048=EDGE_CURVE ( 'NONE', #51642, #50916, #29213, .T. ) ;
#65066=CARTESIAN_POINT ( 'NONE',  ( -68.45261304049999751, 1379.747725225370004, 280.0177415624590367 ) ) ;
#65069=CARTESIAN_POINT ( 'NONE',  ( -8.325002224603874623, 1381.957443703849094, 218.3429956565692009 ) ) ;
#65079=CARTESIAN_POINT ( 'NONE',  ( -14.37112480107839829, 1379.718463779069907, 208.2713378727540032 ) ) ;
#65098=CARTESIAN_POINT ( 'NONE',  ( -63.87186265362610982, 1379.736347229807961, 269.9239848820633370 ) ) ;
#65103=CARTESIAN_POINT ( 'NONE',  ( -74.21209275916879733, 1384.762929623529999, 274.0793104329180210 ) ) ;
#65170=CARTESIAN_POINT ( 'NONE',  ( -26.41820922019849860, 1384.841236826930071, 224.7638030708410213 ) ) ;
#65178=ADVANCED_FACE ( 'NONE', ( #59951 ), #14314, .T. ) ;
#65198=CARTESIAN_POINT ( 'NONE',  ( -44.32308149723269963, 1380.083786705709826, 232.1686127967639948 ) ) ;
#65228=CARTESIAN_POINT ( 'NONE',  ( -109.9855944279999989, 1384.926148861439970, 311.4562326602589906 ) ) ;
#65231=CARTESIAN_POINT ( 'NONE',  ( -12.31856220172990035, 1378.316865691869907, 209.5864139505719947 ) ) ;
#65234=DIRECTION ( 'NONE',  ( 1.000000000000000000, 0.000000000000000000, 0.000000000000000000 ) ) ;
#65236=CARTESIAN_POINT ( 'NONE',  ( -37.01195473260000313, 1375.480374498559968, 219.4187096247589750 ) ) ;
#65249=CARTESIAN_POINT ( 'NONE',  ( -38.49941284300000177, 1384.470821939250072, 239.3076530171589980 ) ) ;
#65254=CARTESIAN_POINT ( 'NONE',  ( -62.92787051930000075, 1379.731629237049901, 267.9834126184589991 ) ) ;
#65262=CARTESIAN_POINT ( 'NONE',  ( -107.2061239200703824, 1391.913060387192672, 300.7511740610627839 ) ) ;
#65263=EDGE_CURVE ( 'NONE', #33852, #103208, #41313, .T. ) ;
#65266=CARTESIAN_POINT ( 'NONE',  ( -25.90890198950000212, 1386.624726539740095, 203.4658880710290134 ) ) ;
#65268=CARTESIAN_POINT ( 'NONE',  ( -38.23615600544859916, 1385.191880958569982, 239.1136682615309894 ) ) ;
#65293=CARTESIAN_POINT ( 'NONE',  ( -107.2861855960000099, 1387.769792023699893, 298.2427032543589576 ) ) ;
#65310=CARTESIAN_POINT ( 'NONE',  ( -105.2320395018850121, 1383.760598056300068, 311.0135867326180232 ) ) ;
#65317=CARTESIAN_POINT ( 'NONE',  ( -106.7756679679999934, 1383.435927837959980, 297.1269841571589723 ) ) ;
#65343=ORIENTED_EDGE ( 'NONE', *, *, #9225, .F. ) ;
#65352=CARTESIAN_POINT ( 'NONE',  ( -8.372579757359998709, 1384.643036033459794, 199.7849846811289751 ) ) ;
#65353=CARTESIAN_POINT ( 'NONE',  ( -120.2678896395927666, 1378.913060387290216, 304.3291340586740716 ) ) ;
#65375=CARTESIAN_POINT ( 'NONE',  ( -12.36124149779879922, 1384.516177574450012, 200.2720669086149883 ) ) ;
#65395=ORIENTED_EDGE ( 'NONE', *, *, #174, .T. ) ;
#65399=ORIENTED_EDGE ( 'NONE', *, *, #42522, .F. ) ;
#65439=CARTESIAN_POINT ( 'NONE',  ( -42.67632043428780264, 1383.823947953480001, 246.6491155685140200 ) ) ;
#65443=CARTESIAN_POINT ( 'NONE',  ( -9.095061913341748294, 1384.893525202921637, 199.9428029920298968 ) ) ;
#65450=CARTESIAN_POINT ( 'NONE',  ( -27.62980858599999578, 1378.955612583270067, 213.6130983169189790 ) ) ;
#65457=CARTESIAN_POINT ( 'NONE',  ( -8.187507831451240392, 1385.403986602129862, 218.7246662665380086 ) ) ;
#65461=CARTESIAN_POINT ( 'NONE',  ( -105.6574850370000007, 1379.068304266050063, 301.9655839248590041 ) ) ;
#65478=CARTESIAN_POINT ( 'NONE',  ( -109.7495287920000067, 1386.092077302740108, 311.3091851462589830 ) ) ;
#65487=CARTESIAN_POINT ( 'NONE',  ( -14.27693757830880017, 1379.587460516140027, 207.9273167693889945 ) ) ;
#65501=CARTESIAN_POINT ( 'NONE',  ( -107.5342874719949862, 1378.913060387359792, 300.5051711733210595 ) ) ;
#65507=CARTESIAN_POINT ( 'NONE',  ( -25.91358801470000373, 1384.684512614960113, 203.4532549264589818 ) ) ;
#65511=CARTESIAN_POINT ( 'NONE',  ( -105.7049770469999999, 1379.426018556420104, 306.8995712054589831 ) ) ;
#65533=CARTESIAN_POINT ( 'NONE',  ( -108.2677198149262665, 1380.892023996865646, 298.2229625968756750 ) ) ;
#65545=CARTESIAN_POINT ( 'NONE',  ( -84.07870740561909884, 1384.983604346920174, 306.2409631616719707 ) ) ;
#65546=CARTESIAN_POINT ( 'NONE',  ( -8.067891928930000844, 1386.126867263409849, 199.6142371476589972 ) ) ;
#65560=DIRECTION ( 'NONE',  ( 1.000000000000000000, 0.000000000000000000, 0.000000000000000000 ) ) ;
#65581=CARTESIAN_POINT ( 'NONE',  ( -105.2473876565402833, 1381.074936998757721, 308.6785104366205132 ) ) ;
#65589=CARTESIAN_POINT ( 'NONE',  ( -58.02100482020349403, 1385.051923325640018, 239.8170954572080120 ) ) ;
#65598=CARTESIAN_POINT ( 'NONE',  ( -109.4840107539999963, 1384.898108854659995, 311.2841325702589756 ) ) ;
#65601=CARTESIAN_POINT ( 'NONE',  ( -109.6410173800000081, 1384.508238210969921, 311.3032840212590031 ) ) ;
#65615=CARTESIAN_POINT ( 'NONE',  ( -5.513264357029999729, 1374.913060387289988, 203.3066656689789795 ) ) ;
#65622=CARTESIAN_POINT ( 'NONE',  ( -68.54965750324760165, 1379.747397323139921, 280.1613699669709945 ) ) ;
#65625=CARTESIAN_POINT ( 'NONE',  ( -8.121603995746610849, 1382.367886013207908, 218.5361279351766370 ) ) ;
#65648=CARTESIAN_POINT ( 'NONE',  ( -14.51248501049999895, 1379.683207487500113, 208.2417184310789935 ) ) ;
#65653=CARTESIAN_POINT ( 'NONE',  ( -69.05319778136079378, 1384.731230461870155, 263.9282964275780046 ) ) ;
#65689=CARTESIAN_POINT ( 'NONE',  ( -109.9643883132849851, 1384.403371867929991, 311.4317840562709989 ) ) ;
#65720=CARTESIAN_POINT ( 'NONE',  ( -58.60893540860839579, 1384.701328510650001, 278.5430915364260613 ) ) ;
#65749=CARTESIAN_POINT ( 'NONE',  ( -43.31858137841459921, 1379.664109115149813, 233.3688221966910135 ) ) ;
#65777=CARTESIAN_POINT ( 'NONE',  ( -109.1276752832161208, 1387.534014296270470, 310.9046063671660249 ) ) ;
#65779=CARTESIAN_POINT ( 'NONE',  ( -13.83795085007070114, 1380.065366606389944, 208.6746515825599886 ) ) ;
#65783=CARTESIAN_POINT ( 'NONE',  ( -52.12027059030000231, 1375.939285429470146, 241.5351867029590096 ) ) ;
#65796=CARTESIAN_POINT ( 'NONE',  ( -54.29265189920000267, 1383.804803630430115, 270.2912082677589751 ) ) ;
#65813=CARTESIAN_POINT ( 'NONE',  ( -41.51449232029999337, 1389.658647050520131, 237.5849401716589853 ) ) ;
#65815=CARTESIAN_POINT ( 'NONE',  ( -53.14043027547860021, 1385.103307817649920, 268.1312696023829858 ) ) ;
#65825=CARTESIAN_POINT ( 'NONE',  ( -7.545064089280000275, 1384.907233277360092, 219.0876311325589825 ) ) ;
#65842=CARTESIAN_POINT ( 'NONE',  ( -108.6690692859999956, 1387.662519259070223, 297.7628581251590276 ) ) ;
#65870=CARTESIAN_POINT ( 'NONE',  ( -8.862456919400310440, 1384.912279086194303, 218.6852231908899569 ) ) ;
#65924=CARTESIAN_POINT ( 'NONE',  ( -10.93176275610840165, 1384.512863483779938, 200.1239762818750023 ) ) ;
#65948=CARTESIAN_POINT ( 'NONE',  ( -8.743364905860000036, 1385.034306932410118, 218.5834041657990099 ) ) ;
#65953=B_SPLINE_SURFACE_WITH_KNOTS ( 'NONE', 5, 5, ( 
 ( #36361, #1680, #86766, #35821, #61588, #87326, #10622, #95721, #69444 ),
 ( #18986, #96275, #105231, #26863, #19553, #53759, #28519, #62719, #80026 ),
 ( #37471, #96840, #61051, #95173, #18429, #88966, #71674, #29075, #97369 ),
 ( #43669, #52629, #63794, #57049, #31819, #38557, #107970, #23412, #55389 ),
 ( #91175, #81653, #82217, #56485, #72736, #73280, #106861, #47532, #14454 ),
 ( #100128, #12811, #82775, #66007, #90616, #97908, #98466, #31267, #3894 ),
 ( #55938, #90058, #5520, #21179, #4959, #80579, #48648, #30153, #39102 ),
 ( #40221, #29609, #73843, #22843, #65450, #13896, #13340, #64345, #57605 ),
 ( #74402, #38024, #72203, #107417, #30714, #89519, #99559, #64899, #46990 ),
 ( #81114, #4431, #99007, #22283, #21736, #106326, #39676, #48083, #6068 ),
 ( #46447, #108528, #12257, #33452, #109637, #25605, #76032, #102318, #34022 ),
 ( #6619, #26160, #92824, #58144, #8256, #32379, #16098, #51378, #66561 ),
 ( #453, #7177, #76580, #102863, #23947, #49744, #59797, #50303, #50833 ),
 ( #93917, #85512, #110732, #14997, #84431, #100664, #93370, #8808, #68214 ),
 ( #92275, #84964, #67653, #16637, #42422, #7716, #41876, #17184, #40773 ),
 ( #42991, #110180, #68759, #101761, #15544, #77149, #25050, #34574, #91723 ),
 ( #59252, #49196, #41333, #83324, #83872, #74950, #109099, #101205, #75503 ),
 ( #32910, #67103, #24501, #58691, #78797, #45770, #86631, #53621, #1001 ),
 ( #36792, #69869, #70984, #51943, #104544, #9925, #10485, #44096, #95590 ),
 ( #9380, #37346, #60914, #19978, #79906, #27840, #35128, #35679, #45213 ),
 ( #69310, #103985, #27281, #87763, #103417, #53055, #17742, #28390, #78234 ),
 ( #2112, #61464, #19419, #3219, #87193, #86086, #44656, #95042, #18859 ),
 ( #43543, #11044, #79353, #52502, #36238, #26724, #77688, #71544, #18311 ),
 ( #2666, #105100, #96708, #96140, #62020, #105666, #70425, #1547, #60346 ),
 ( #94468, #62591, #54172, #88298, #11592, #73721, #13214, #39546, #82086 ),
 ( #20512, #54721, #74272, #30024, #106197, #56356, #80455, #64217, #99428 ),
 ( #107844, #48514, #55268, #13763, #40090, #72083, #97786, #31133, #98341 ),
 ( #3767, #65317, #22706, #47947, #63138, #21614, #37902, #30590, #56904 ),
 ( #38430, #29479, #22155, #81526, #64778, #98888, #55819, #89938, #5389 ),
 ( #82653, #91037, #47404, #5945, #4828, #63674, #14324, #28949, #97239 ) ),
 .UNSPECIFIED., .F., .F., .F.,
 ( 6, 3, 3, 3, 3, 3, 3, 3, 3, 6 ),
 ( 6, 3, 6 ),
 ( -3.552713678800000397E-15, 15.39383910899999997, 27.58084801740000103, 41.39509552349999666, 65.53909258059999843, 90.91108773649999364, 117.6367619669999982, 132.4493970709999928, 144.8160795070000120, 161.8240513320000105 ),
 ( 2.092690777440000094, 17.86261146360000041, 33.63253214979999939 ),
 .UNSPECIFIED. ) ;
#65980=CARTESIAN_POINT ( 'NONE',  ( -109.1665242455550100, 1385.079937276020019, 297.1361710942769605 ) ) ;
#65999=CARTESIAN_POINT ( 'NONE',  ( -47.66019703560549914, 1383.815780539829802, 256.5296040942980085 ) ) ;
#66007=CARTESIAN_POINT ( 'NONE',  ( -21.97707892889999926, 1380.247610671960047, 205.6383942844589967 ) ) ;
#66011=CARTESIAN_POINT ( 'NONE',  ( -8.348311995175087930, 1386.164425872750144, 218.5824697249680071 ) ) ;
#66015=CARTESIAN_POINT ( 'NONE',  ( -104.9457213230000008, 1380.324877816590060, 300.8469997012589943 ) ) ;
#66033=CARTESIAN_POINT ( 'NONE',  ( -109.0087032940000000, 1387.252923815580061, 310.8549776262589717 ) ) ;
#66065=CARTESIAN_POINT ( 'NONE',  ( -37.21633441560000222, 1384.983113612510124, 210.1703949109789846 ) ) ;
#66069=CIRCLE ( 'NONE', #19513, 2.000012855935070721 ) ;
#66098=CARTESIAN_POINT ( 'NONE',  ( -11.78930676389999910, 1378.156676306969985, 212.7700627114790279 ) ) ;
#66107=CARTESIAN_POINT ( 'NONE',  ( -8.257938479109999008, 1385.286773756459979, 199.7059428756689954 ) ) ;
#66121=CARTESIAN_POINT ( 'NONE',  ( -108.0197652269449407, 1389.258088431015722, 298.4547169909268405 ) ) ;
#66147=CARTESIAN_POINT ( 'NONE',  ( -104.4180155810560535, 1380.492968669763968, 307.4335991971175872 ) ) ;
#66154=CARTESIAN_POINT ( 'NONE',  ( -14.23129321600000097, 1380.257846505089901, 210.5264815996590073 ) ) ;
#66156=CARTESIAN_POINT ( 'NONE',  ( -61.95008448870819961, 1385.071029117499847, 248.2449222687090185 ) ) ;
#66167=CARTESIAN_POINT ( 'NONE',  ( -109.2887680899999907, 1384.559956795920016, 311.2476293452589857 ) ) ;
#66183=CARTESIAN_POINT ( 'NONE',  ( -68.66299202070430852, 1379.747740319620107, 280.2603170350629966 ) ) ;
#66186=CARTESIAN_POINT ( 'NONE',  ( -9.362891644902104460, 1380.380461215845344, 217.2234689991179550 ) ) ;
#66218=CARTESIAN_POINT ( 'NONE',  ( -10.91416569499999945, 1391.310101084879989, 214.8368661670989752 ) ) ;
#66219=CARTESIAN_POINT ( 'NONE',  ( -73.07052337915050089, 1384.756188251220010, 271.9861327822499675 ) ) ;
#66258=CARTESIAN_POINT ( 'NONE',  ( -109.9685895047820026, 1384.440684789770103, 311.4348663963149306 ) ) ;
#66261=DIRECTION ( 'NONE',  ( 1.835183309750130004E-16, 1.000000000000000000, 1.599799320660000123E-19 ) ) ;
#66272=CARTESIAN_POINT ( 'NONE',  ( -8.571699234208210783, 1388.295717325432861, 218.1000065865680710 ) ) ;
#66289=CARTESIAN_POINT ( 'NONE',  ( -50.80134176948489966, 1384.736217744079795, 263.3871381538430114 ) ) ;
#66290=CARTESIAN_POINT ( 'NONE',  ( -106.4627743365379899, 1391.913060387289988, 303.3857292504940233 ) ) ;
#66317=CARTESIAN_POINT ( 'NONE',  ( -56.82419418675780776, 1379.716300530480112, 259.5363713978089777 ) ) ;
#66350=CARTESIAN_POINT ( 'NONE',  ( -57.70298350590000069, 1377.436376805819918, 252.0908766120590201 ) ) ;
#66351=EDGE_LOOP ( 'NONE', ( #28889, #75420, #28222, #42420 ) ) ;
#66359=VERTEX_POINT ( 'NONE', #69431 ) ;
#66362=CARTESIAN_POINT ( 'NONE',  ( -43.23635582379999676, 1383.823167092340100, 247.4293989253590098 ) ) ;
#66376=CARTESIAN_POINT ( 'NONE',  ( -50.36169832019999859, 1389.574744497710071, 254.8962280555589928 ) ) ;
#66378=CARTESIAN_POINT ( 'NONE',  ( -45.19369995658139771, 1385.151324122020014, 251.9073361886829900 ) ) ;
#66381=CIRCLE ( 'NONE', #68141, 8.013264357029999729 ) ;
#66387=FACE_OUTER_BOUND ( 'NONE', #32711, .T. ) ;
#66400=CARTESIAN_POINT ( 'NONE',  ( -105.4624709189999834, 1391.255327103129957, 304.2078109453590287 ) ) ;
#66403=CARTESIAN_POINT ( 'NONE',  ( -105.5788448139999929, 1390.041791431060119, 301.0601375796589991 ) ) ;
#66408=ORIENTED_EDGE ( 'NONE', *, *, #76451, .T. ) ;
#66460=CARTESIAN_POINT ( 'NONE',  ( -8.847783283049999170, 1384.881200138800068, 199.9249094011889838 ) ) ;
#66480=EDGE_CURVE ( 'NONE', #68857, #61100, #52618, .T. ) ;
#66485=CARTESIAN_POINT ( 'NONE',  ( -35.17588676205760123, 1384.569143118210150, 208.8585631465319921 ) ) ;
#66491=VERTEX_POINT ( 'NONE', #39087 ) ;
#66495=CARTESIAN_POINT ( 'NONE',  ( -10.36756237719999874, 1382.682511944280122, 200.8304498154890041 ) ) ;
#66500=CARTESIAN_POINT ( 'NONE',  ( -68.77575455639998836, 1379.747977220560188, 280.2449803406589695 ) ) ;
#66508=CARTESIAN_POINT ( 'NONE',  ( -3.078458293620000230, 1385.190530866809922, 218.5645787212890241 ) ) ;
#66551=CARTESIAN_POINT ( 'NONE',  ( -48.47771611847429796, 1383.814425808469878, 258.2089094142469889 ) ) ;
#66561=CARTESIAN_POINT ( 'NONE',  ( -36.25797752260000095, 1383.833857111379984, 235.3800711337590030 ) ) ;
#66566=CARTESIAN_POINT ( 'NONE',  ( -8.464911085096829879, 1385.365015953710099, 218.6689375795459966 ) ) ;
#66571=CARTESIAN_POINT ( 'NONE',  ( -105.7409752579999918, 1381.140865015730242, 299.3151906013590065 ) ) ;
#66590=CARTESIAN_POINT ( 'NONE',  ( -109.8314448029999966, 1386.134759465500110, 311.3488533982589388 ) ) ;
#66599=CARTESIAN_POINT ( 'NONE',  ( -14.30024709372010072, 1379.589079739520002, 207.9540921923399708 ) ) ;
#66607=CARTESIAN_POINT ( 'NONE',  ( -5.432410439650000811, 1391.426148861440197, 214.9021618825790085 ) ) ;
#66619=CARTESIAN_POINT ( 'NONE',  ( -31.91391880200000131, 1384.560375756019766, 206.3213236589990061 ) ) ;
#66648=CARTESIAN_POINT ( 'NONE',  ( -12.24671249760000080, 1378.552623650770101, 211.6779590913389768 ) ) ;
#66650=ORIENTED_EDGE ( 'NONE', *, *, #73820, .F. ) ;
#66653=CARTESIAN_POINT ( 'NONE',  ( -108.2120120822389850, 1384.926448218169980, 311.2629986585570236 ) ) ;
#66654=CARTESIAN_POINT ( 'NONE',  ( -10.17260142399999978, 1386.954104889990049, 200.6847011332289981 ) ) ;
#66690=CARTESIAN_POINT ( 'NONE',  ( -105.8150085967258605, 1381.470779566475130, 309.3040015815146830 ) ) ;
#66694=CARTESIAN_POINT ( 'NONE',  ( -108.2287821362297251, 1381.019133052909638, 310.1919587077548499 ) ) ;
#66698=CARTESIAN_POINT ( 'NONE',  ( -54.33537259569690292, 1385.035685468000111, 232.6071117302159905 ) ) ;
#66705=CARTESIAN_POINT ( 'NONE',  ( -109.1309838760000019, 1384.924126712679936, 311.2646841762590384 ) ) ;
#66709=CARTESIAN_POINT ( 'NONE',  ( -109.8184593100000086, 1384.563165728690137, 311.3672836522590046 ) ) ;
#66727=CARTESIAN_POINT ( 'NONE',  ( -107.2902847454959954, 1391.913060387289988, 307.3027153792770036 ) ) ;
#66729=CARTESIAN_POINT ( 'NONE',  ( -68.49156254684720579, 1379.747260696060039, 280.0978574668839656 ) ) ;
#66732=CARTESIAN_POINT ( 'NONE',  ( -11.18760872067141321, 1378.375624679992598, 214.3033515264987727 ) ) ;
#66740=CARTESIAN_POINT ( 'NONE',  ( -106.6028128171490010, 1378.913060387289988, 306.5905933178560190 ) ) ;
#66760=CARTESIAN_POINT ( 'NONE',  ( -12.31967538750000202, 1378.053937865659918, 209.2867312853659882 ) ) ;
#66764=ADVANCED_FACE ( 'NONE', ( #22693 ), #81288, .T. ) ;
#66765=CARTESIAN_POINT ( 'NONE',  ( -11.69890093100000072, 1391.698097032839769, 212.7312234011589851 ) ) ;
#66766=CARTESIAN_POINT ( 'NONE',  ( -74.96309076845238906, 1384.767266604889983, 275.4021836984660467 ) ) ;
#66788=EDGE_LOOP ( 'NONE', ( #103246, #96537, #87912, #11630 ) ) ;
#66797=CARTESIAN_POINT ( 'NONE',  ( -8.156761245049999332, 1384.910749514120198, 199.6468897218990151 ) ) ;
#66807=LINE ( 'NONE', #102561, #49652 ) ;
#66831=CARTESIAN_POINT ( 'NONE',  ( -46.05768597449060309, 1384.759096880909965, 253.6622143525649733 ) ) ;
#66832=CARTESIAN_POINT ( 'NONE',  ( -106.4480318723080075, 1391.913060387289988, 303.4929453003720141 ) ) ;
#66838=CARTESIAN_POINT ( 'NONE',  ( -9.270207532385544624, 1381.215922526254872, 200.8810307281849532 ) ) ;
#66852=AXIS2_PLACEMENT_3D ( 'NONE', #21384, #53386, #20847 ) ;
#66859=CARTESIAN_POINT ( 'NONE',  ( -3.771520285720249888, 1380.389610322579983, 209.1217750815700072 ) ) ;
#66862=CARTESIAN_POINT ( 'NONE',  ( -52.20072447709220143, 1379.700295299539903, 250.0227394179869691 ) ) ;
#66869=CARTESIAN_POINT ( 'NONE',  ( -105.2826783650000095, 1379.306804825290101, 305.8448452370589621 ) ) ;
#66889=CARTESIAN_POINT ( 'NONE',  ( -108.0818973204794418, 1388.984710564502166, 310.0551414095012319 ) ) ;
#66896=CARTESIAN_POINT ( 'NONE',  ( -7.567621161430000853, 1375.366160259910203, 208.3364483328870165 ) ) ;
#66909=CARTESIAN_POINT ( 'NONE',  ( -67.18675499840000498, 1383.787653363379832, 292.0788269227589922 ) ) ;
#66921=CARTESIAN_POINT ( 'NONE',  ( -55.46135264680000176, 1389.548669515830170, 241.4579668749589985 ) ) ;
#66923=CARTESIAN_POINT ( 'NONE',  ( -49.22592528755399854, 1385.126725678709818, 260.1312381994819702 ) ) ;
#66949=CARTESIAN_POINT ( 'NONE',  ( -109.9057131499999969, 1385.910548283320168, 297.0533992618589991 ) ) ;
#66979=CARTESIAN_POINT ( 'NONE',  ( -12.30864129963430109, 1378.374850116299967, 209.8264313038230000 ) ) ;
#66986=CARTESIAN_POINT ( 'NONE',  ( -113.3410085367727334, 1390.913060387289988, 301.7225420527170172 ) ) ;
#67027=CARTESIAN_POINT ( 'NONE',  ( -47.05400443392269949, 1384.607290103919922, 220.9981132380000020 ) ) ;
#67039=CARTESIAN_POINT ( 'NONE',  ( -68.78035032010001260, 1379.747955697800080, 280.2621870389589844 ) ) ;
#67090=DIRECTION ( 'NONE',  ( -6.162707975952100561E-15, -1.000000000000000000, -1.094450614310000083E-14 ) ) ;
#67095=CARTESIAN_POINT ( 'NONE',  ( -73.43657703184560148, 1383.782119018540016, 298.3839446379640208 ) ) ;
#67103=CARTESIAN_POINT ( 'NONE',  ( -73.04349225800000056, 1383.258802109350199, 272.3818029833590231 ) ) ;
#67106=ORIENTED_EDGE ( 'NONE', *, *, #94509, .F. ) ;
#67107=CARTESIAN_POINT ( 'NONE',  ( -8.605913743462409116, 1385.346776729300018, 218.6535381029370058 ) ) ;
#67112=CARTESIAN_POINT ( 'NONE',  ( -104.6820493169999935, 1380.404521281969892, 300.7508435114589815 ) ) ;
#67132=CARTESIAN_POINT ( 'NONE',  ( -104.5024257390000031, 1390.098467524800071, 305.3418556385589682 ) ) ;
#67160=CARTESIAN_POINT ( 'NONE',  ( -53.47364387789999540, 1384.899415174140131, 230.7470315883589933 ) ) ;
#67189=CARTESIAN_POINT ( 'NONE',  ( -11.99239960049999887, 1380.797795605900092, 215.7904316102089979 ) ) ;
#67198=CARTESIAN_POINT ( 'NONE',  ( -10.84052017329999806, 1388.346876310129801, 201.9571177318990181 ) ) ;
#67205=EDGE_CURVE ( 'NONE', #81708, #26498, #30163, .T. ) ;
#67222=CARTESIAN_POINT ( 'NONE',  ( -11.20885044277319942, 1383.862009336539813, 218.6925135829310136 ) ) ;
#67235=CARTESIAN_POINT ( 'NONE',  ( -109.1652045310000005, 1384.878244280709850, 297.1328263764589792 ) ) ;
#67240=CARTESIAN_POINT ( 'NONE',  ( -104.0864640810399635, 1380.258016915853659, 306.7182003634226817 ) ) ;
#67248=CARTESIAN_POINT ( 'NONE',  ( -70.69551388654410573, 1385.115795056309935, 267.3360060303040200 ) ) ;
#67262=CARTESIAN_POINT ( 'NONE',  ( -109.1169852539999994, 1384.611753107699997, 311.2523998022589922 ) ) ;
#67268=CARTESIAN_POINT ( 'NONE',  ( -13.73095700724906543, 1379.766849082292993, 213.0184867138244442 ) ) ;
#67277=CARTESIAN_POINT ( 'NONE',  ( -68.46644754685360112, 1379.747474136280061, 280.0435952495369634 ) ) ;
#67281=CARTESIAN_POINT ( 'NONE',  ( -10.29823179855451265, 1379.271150225059955, 215.9527657008635231 ) ) ;
#67300=VERTEX_POINT ( 'NONE', #105936 ) ;
#67303=CARTESIAN_POINT ( 'NONE',  ( -14.28952585159370159, 1380.314717283680011, 210.1167927017139903 ) ) ;
#67310=CARTESIAN_POINT ( 'NONE',  ( -11.83879355810000078, 1391.851285459460087, 211.5674355249090013 ) ) ;
#67311=CARTESIAN_POINT ( 'NONE',  ( -85.93326510183719336, 1384.821889067519805, 289.5792165609069571 ) ) ;
#67329=CARTESIAN_POINT ( 'NONE',  ( -62.16362557989999971, 1379.729112816429961, 266.3118224345589624 ) ) ;
#67345=CARTESIAN_POINT ( 'NONE',  ( -8.156587055619999305, 1384.920249147410232, 199.6468410606589998 ) ) ;
#67363=EDGE_CURVE ( 'NONE', #49086, #90041, #2456, .T. ) ;
#67366=CARTESIAN_POINT ( 'NONE',  ( -9.640608181049721281, 1389.788252704991919, 216.8809208289262358 ) ) ;
#67374=B_SPLINE_CURVE_WITH_KNOTS ( 'NONE', 5,
 ( #3096, #106617, #54601, #96581, #12017, #20945 ),
 .UNSPECIFIED., .F., .F.,
 ( 6, 6 ),
 ( -2.000000000000000000, 0.000000000000000000 ),
 .UNSPECIFIED. ) ;
#67382=CARTESIAN_POINT ( 'NONE',  ( -12.41968314313910682, 1391.384630218451093, 211.0556431160394197 ) ) ;
#67383=ADVANCED_FACE ( 'NONE', ( #21872 ), #89658, .F. ) ;
#67385=CARTESIAN_POINT ( 'NONE',  ( -46.40682475798950435, 1384.757411015490106, 254.3673974098619794 ) ) ;
#67386=CARTESIAN_POINT ( 'NONE',  ( -106.6958069642329860, 1391.913060387289988, 302.4589463478089897 ) ) ;
#67388=CARTESIAN_POINT ( 'NONE',  ( -107.6455384790000096, 1378.913060387289988, 299.9332720164590000 ) ) ;
#67393=CARTESIAN_POINT ( 'NONE',  ( -9.033771706128597145, 1381.576731241501420, 200.6091943981350312 ) ) ;
#67401=CARTESIAN_POINT ( 'NONE',  ( -13.41525439013790155, 1379.584674364849889, 211.7907235378989981 ) ) ;
#67412=CARTESIAN_POINT ( 'NONE',  ( -35.15050912068899436, 1380.172863641740150, 221.1654657214490101 ) ) ;
#67415=CARTESIAN_POINT ( 'NONE',  ( -36.52309517079940093, 1379.688050188520037, 223.7231089615120254 ) ) ;
#67421=CARTESIAN_POINT ( 'NONE',  ( -105.8600500019999942, 1378.913059667080006, 305.6175922275590437 ) ) ;
#67439=ORIENTED_EDGE ( 'NONE', *, *, #94615, .T. ) ;
#67448=CARTESIAN_POINT ( 'NONE',  ( -26.37171023119999802, 1379.942807944750029, 211.7994354412990106 ) ) ;
#67472=CARTESIAN_POINT ( 'NONE',  ( -49.69844455709999664, 1386.731746342069755, 260.8593201508589914 ) ) ;
#67474=CARTESIAN_POINT ( 'NONE',  ( -52.69031413145209797, 1385.105943313089938, 267.2253354263970095 ) ) ;
#67485=CARTESIAN_POINT ( 'NONE',  ( -8.297681820259999341, 1384.894008818040220, 218.7035870978390051 ) ) ;
#67487=CARTESIAN_POINT ( 'NONE',  ( -109.6092339890690113, 1383.179580026969916, 311.2151190870969799 ) ) ;
#67501=CARTESIAN_POINT ( 'NONE',  ( -109.4241442180000092, 1385.278508194390042, 297.1426266650590264 ) ) ;
#67525=CARTESIAN_POINT ( 'NONE',  ( -12.04245058442665695, 1377.963961494413525, 211.7131635820066435 ) ) ;
#67534=CARTESIAN_POINT ( 'NONE',  ( -12.31039754504540085, 1378.376187213689946, 209.7956876274450053 ) ) ;
#67535=CIRCLE ( 'NONE', #74729, 11.34254167809999991 ) ;
#67552=CARTESIAN_POINT ( 'NONE',  ( -7.963748113860001254, 1384.780449526809889, 199.4915856325789889 ) ) ;
#67563=ORIENTED_EDGE ( 'NONE', *, *, #74939, .T. ) ;
#67576=CARTESIAN_POINT ( 'NONE',  ( -45.63678974650149911, 1384.601836401760011, 219.1382722429960097 ) ) ;
#67577=CARTESIAN_POINT ( 'NONE',  ( -14.51138743262410102, 1379.682357218360039, 208.2400043102109919 ) ) ;
#67578=CARTESIAN_POINT ( 'NONE',  ( -108.6463189709999995, 1386.108622646309868, 311.0727272582590217 ) ) ;
#67583=CARTESIAN_POINT ( 'NONE',  ( -55.83192871552868297, 1379.712800777655048, 257.4612982601994986 ) ) ;
#67588=CARTESIAN_POINT ( 'NONE',  ( -68.71298160489999418, 1379.747970726529957, 280.0474361183589735 ) ) ;
#67609=CARTESIAN_POINT ( 'NONE',  ( -8.878224064888490474, 1385.253402910369914, 218.6672395676210101 ) ) ;
#67622=DIRECTION ( 'NONE',  ( 0.000000000000000000, -1.000000000000000000, 0.000000000000000000 ) ) ;
#67628=DIRECTION ( 'NONE',  ( 1.000000000000000000, 0.000000000000000000, 0.000000000000000000 ) ) ;
#67645=CARTESIAN_POINT ( 'NONE',  ( -56.77970903073529740, 1383.801243860249997, 274.8410118865560321 ) ) ;
#67653=CARTESIAN_POINT ( 'NONE',  ( -61.45879576459999782, 1381.674944668329999, 249.7621233603589985 ) ) ;
#67663=CARTESIAN_POINT ( 'NONE',  ( -108.8778232199999962, 1382.941140509790102, 297.5244794079590065 ) ) ;
#67675=B_SPLINE_CURVE_WITH_KNOTS ( 'NONE', 5,
 ( #39391, #30984, #31534, #97648, #73006, #55668 ),
 .UNSPECIFIED., .F., .F.,
 ( 6, 6 ),
 ( 0.000000000000000000, 1.000000000000000000 ),
 .UNSPECIFIED. ) ;
#67686=CARTESIAN_POINT ( 'NONE',  ( -108.0873157920000125, 1388.188583901430093, 310.1965002822589668 ) ) ;
#67722=CARTESIAN_POINT ( 'NONE',  ( -10.68745674553450087, 1391.913060387239966, 205.2244091230350023 ) ) ;
#67742=CARTESIAN_POINT ( 'NONE',  ( -11.23128131019999998, 1378.642388353129945, 214.2935887347389894 ) ) ;
#67748=CARTESIAN_POINT ( 'NONE',  ( -14.02793429120000113, 1390.368118300530114, 208.3706668749019855 ) ) ;
#67753=CARTESIAN_POINT ( 'NONE',  ( -8.860697296614830520, 1384.856270409599801, 218.6846939278150046 ) ) ;
#67758=CARTESIAN_POINT ( 'NONE',  ( -7.769784805680000517, 1383.283764732429972, 218.8591787099389876 ) ) ;
#67767=CARTESIAN_POINT ( 'NONE',  ( -17.22212745223800212, 1383.856419954710191, 219.8022064494420249 ) ) ;
#67780=CARTESIAN_POINT ( 'NONE',  ( -109.8954864790000130, 1384.895399018540047, 297.0284339997589882 ) ) ;
#67793=CARTESIAN_POINT ( 'NONE',  ( -12.23230767969999810, 1391.519584735709941, 206.9802348098490086 ) ) ;
#67794=CARTESIAN_POINT ( 'NONE',  ( -81.94711355757770832, 1385.165090159550118, 285.5376096483210517 ) ) ;
#67795=CARTESIAN_POINT ( 'NONE',  ( -10.38284638997270015, 1391.913060387289988, 213.8006219875449858 ) ) ;
#67802=VERTEX_POINT ( 'NONE', #21067 ) ;
#67822=CARTESIAN_POINT ( 'NONE',  ( -68.61467808968738780, 1379.747555724440190, 280.2219422655999779 ) ) ;
#67837=CARTESIAN_POINT ( 'NONE',  ( -12.47841591940709982, 1378.791065535750022, 209.0505839962389985 ) ) ;
#67850=CARTESIAN_POINT ( 'NONE',  ( -14.31906343784990021, 1380.323795378649947, 209.9058136714729983 ) ) ;
#67860=CARTESIAN_POINT ( 'NONE',  ( -94.44617500847539304, 1384.855411388800121, 294.7348737027389802 ) ) ;
#67873=( BOUNDED_CURVE ( )  B_SPLINE_CURVE ( 3, ( #68182, #103381, #424, #42957 ),
 .UNSPECIFIED., .F., .F. ) 
 B_SPLINE_CURVE_WITH_KNOTS ( ( 4, 4 ),
 ( 1.529854054923474926, 1.666126868289663721 ),
 .UNSPECIFIED. ) 
 CURVE ( )  GEOMETRIC_REPRESENTATION_ITEM ( )  RATIONAL_B_SPLINE_CURVE ( ( 1.000000000000000000, 0.9984530753092233368, 0.9984530753092233368, 1.000000000000000000 ) ) 
 REPRESENTATION_ITEM ( '' )  );
#67880=CARTESIAN_POINT ( 'NONE',  ( -56.77117924490000433, 1379.710828546099947, 254.2839483103589941 ) ) ;
#67896=CARTESIAN_POINT ( 'NONE',  ( -8.371593325730000146, 1384.916486876450108, 199.7749919984989901 ) ) ;
#67907=AXIS2_PLACEMENT_3D ( 'NONE', #44811, #89412, #43144 ) ;
#67935=CARTESIAN_POINT ( 'NONE',  ( -42.89705200377979821, 1384.774197275369943, 247.4398508610279919 ) ) ;
#67936=CARTESIAN_POINT ( 'NONE',  ( -13.67545600135260031, 1384.939478993019975, 200.4147283641960087 ) ) ;
#67941=CARTESIAN_POINT ( 'NONE',  ( 12.26364123839999820, 1375.886883438980021, 209.1218459572589836 ) ) ;
#67954=CARTESIAN_POINT ( 'NONE',  ( -9.226044223009999712, 1381.782332506340026, 200.7881398668789927 ) ) ;
#67969=CARTESIAN_POINT ( 'NONE',  ( -31.47360974209560069, 1379.679433932790062, 219.1936121500959871 ) ) ;
#67975=CARTESIAN_POINT ( 'NONE',  ( -106.7853852970000048, 1379.183277988550117, 308.1922113726590169 ) ) ;
#67980=DIRECTION ( 'NONE',  ( -1.000000000000000000, 0.000000000000000000, 0.000000000000000000 ) ) ;
#67991=ORIENTED_EDGE ( 'NONE', *, *, #81643, .F. ) ;
#68003=CARTESIAN_POINT ( 'NONE',  ( 7.203018087042108522E-14, 1375.720597897399784, 207.5503168488490076 ) ) ;
#68008=CONICAL_SURFACE ( 'NONE', #17910, 8.000000000000003553, 0.02617993877989872875 ) ;
#68029=CARTESIAN_POINT ( 'NONE',  ( -75.49308973149999247, 1385.139059930169878, 276.6890413075590232 ) ) ;
#68031=CARTESIAN_POINT ( 'NONE',  ( -65.68353430217270272, 1385.040512093280086, 289.6969188980430090 ) ) ;
#68042=CARTESIAN_POINT ( 'NONE',  ( -107.6966557359999968, 1380.358943897680092, 309.6768259782589894 ) ) ;
#68047=CARTESIAN_POINT ( 'NONE',  ( 8.013264357029996177, 1374.913060387290216, 209.1218459572589836 ) ) ;
#68056=CARTESIAN_POINT ( 'NONE',  ( -109.3769603020000005, 1386.852787485200224, 297.3396656358589780 ) ) ;
#68092=CARTESIAN_POINT ( 'NONE',  ( -12.31029123717709872, 1378.376174907870109, 209.7976204910740137 ) ) ;
#68108=AXIS2_PLACEMENT_3D ( 'NONE', #2704, #78272, #18899 ) ;
#68139=CARTESIAN_POINT ( 'NONE',  ( -39.93074616002299848, 1384.582610175510126, 212.8423831063259968 ) ) ;
#68141=AXIS2_PLACEMENT_3D ( 'NONE', #13754, #54711, #79341 ) ;
#68147=CARTESIAN_POINT ( 'NONE',  ( -47.49308081550576333, 1379.683368846476242, 241.0371517381914543 ) ) ;
#68153=CARTESIAN_POINT ( 'NONE',  ( -68.64714017240000032, 1379.747635037359942, 279.8389543138589488 ) ) ;
#68161=CARTESIAN_POINT ( 'NONE',  ( -5.959427381639999410, 1385.323914143830052, 218.4985401614089824 ) ) ;
#68163=DIRECTION ( 'NONE',  ( -1.836970198721029688E-16, -1.000000000000000000, 0.000000000000000000 ) ) ;
#68182=CARTESIAN_POINT ( 'NONE',  ( -109.1321487942470014, 1384.869787291219836, 311.2644937792119322 ) ) ;
#68185=CARTESIAN_POINT ( 'NONE',  ( -7.545069326662110498, 1384.921616245829910, 219.0875787902100171 ) ) ;
#68197=ORIENTED_EDGE ( 'NONE', *, *, #24762, .T. ) ;
#68206=LINE ( 'NONE', #41865, #25420 ) ;
#68208=CARTESIAN_POINT ( 'NONE',  ( -58.43686276432150351, 1383.798853279400191, 277.8809885620339628 ) ) ;
#68210=FACE_OUTER_BOUND ( 'NONE', #75392, .T. ) ;
#68214=CARTESIAN_POINT ( 'NONE',  ( -43.23635582379999676, 1383.823167092340100, 247.4293989253590098 ) ) ;
#68216=ORIENTED_EDGE ( 'NONE', *, *, #82837, .F. ) ;
#68224=CARTESIAN_POINT ( 'NONE',  ( -109.0547027409999998, 1384.148091023459756, 297.1846209902590203 ) ) ;
#68248=CARTESIAN_POINT ( 'NONE',  ( -106.1218566759999931, 1390.573852006310062, 307.5911815855589566 ) ) ;
#68257=CARTESIAN_POINT ( 'NONE',  ( -10.17260142399999978, 1386.954104889990049, 200.6847011332289981 ) ) ;
#68298=CARTESIAN_POINT ( 'NONE',  ( -17.91820893009999693, 1388.567218049629901, 218.5290927580890070 ) ) ;
#68306=CARTESIAN_POINT ( 'NONE',  ( -12.87022724600000068, 1379.571428314189916, 212.7941117598390122 ) ) ;
#68312=CARTESIAN_POINT ( 'NONE',  ( -11.34705161930000017, 1388.497955604420213, 202.3274404867889871 ) ) ;
#68348=CARTESIAN_POINT ( 'NONE',  ( -12.10381429186880098, 1391.176685838770027, 212.4734229069189837 ) ) ;
#68355=CARTESIAN_POINT ( 'NONE',  ( -12.28448051250000006, 1391.742831658529894, 209.7423389907770002 ) ) ;
#68356=CARTESIAN_POINT ( 'NONE',  ( -82.21241141603550773, 1385.166088929280022, 285.8448996073630042 ) ) ;
#68394=CARTESIAN_POINT ( 'NONE',  ( -13.12590621660049983, 1379.413787799840065, 208.5216990791799958 ) ) ;
#68416=CARTESIAN_POINT ( 'NONE',  ( -11.04795325579999954, 1391.825117937869891, 213.7027257443090207 ) ) ;
#68417=CARTESIAN_POINT ( 'NONE',  ( -88.24446303712089446, 1384.831625806059947, 291.4064741984150260 ) ) ;
#68433=CARTESIAN_POINT ( 'NONE',  ( -14.13710051290000003, 1379.612303426159997, 208.0723505047189974 ) ) ;
#68484=CARTESIAN_POINT ( 'NONE',  ( -63.63973605229279684, 1384.682326359059971, 286.7712759306380121 ) ) ;
#68499=EDGE_CURVE ( 'NONE', #8871, #26117, #87506, .T. ) ;
#68502=CARTESIAN_POINT ( 'NONE',  ( -12.91320920036129927, 1379.508606576809825, 211.2369201494429944 ) ) ;
#68515=CARTESIAN_POINT ( 'NONE',  ( -60.23506803088569939, 1379.735844319070111, 265.9408027383549893 ) ) ;
#68531=SURFACE_SIDE_STYLE ('',( #51722 ) ) ;
#68547=CARTESIAN_POINT ( 'NONE',  ( -34.38452233966944505, 1379.638702217783703, 217.4075408561711527 ) ) ;
#68548=CARTESIAN_POINT ( 'NONE',  ( -19.47048158160000142, 1377.796266888499986, 207.6494986257190192 ) ) ;
#68556=B_SPLINE_CURVE_WITH_KNOTS ( 'NONE', 3,
 ( #29805, #70210, #104315, #46088, #63451, #62346, #63993, #98104, #27608, #61793, #95915, #53381, #10817, #44987, #79135, #2443, #104868, #96471, #19750, #57242, #14090, #30350, #49372, #23038, #82423, #40955, #5719, #47172, #66740, #74579, #100843, #39863, #75134, #91371, #99748, #48279, #74027, #108160, #56117, #40402, #81300, #73481, #23600, #100314, #30899, #90251, #21922, #14651, #38749, #48838, #57788, #108715 ),
 .UNSPECIFIED., .F., .F.,
 ( 4, 3, 3, 3, 3, 3, 3, 3, 3, 3, 3, 3, 3, 3, 3, 3, 3, 4 ),
 ( -12.17647483446349987, -11.45127338244570048, -10.72607193042779983, -9.975235041999999552, -9.382994760010351598, -8.586766221277258637, -7.762798876129999748, -7.064923798146399925, -6.276317141653310117, -5.531936552890000414, -4.937941270824259377, -4.105330589925559437, -3.273015945220000944, -3.105111820674819612, -2.294061070765691213, -1.507377760193390870, -0.7388578846428242031, -2.629008122312370688E-13 ),
 .UNSPECIFIED. ) ;
#68573=CARTESIAN_POINT ( 'NONE',  ( -53.42810237920000560, 1386.663619491189820, 230.7733755451590127 ) ) ;
#68575=CARTESIAN_POINT ( 'NONE',  ( -74.53493904026449002, 1385.009369445449920, 299.6431026865259923 ) ) ;
#68584=CARTESIAN_POINT ( 'NONE',  ( -108.7614019690100093, 1383.708971085589837, 311.0587876456319805 ) ) ;
#68654=CARTESIAN_POINT ( 'NONE',  ( -8.868478827680000620, 1384.515996041270000, 199.9512279144889817 ) ) ;
#68662=VERTEX_POINT ( 'NONE', #109257 ) ;
#68665=B_SPLINE_CURVE_WITH_KNOTS ( 'NONE', 3,
 ( #588, #92403, #93506, #51527, #77831, #9512, #92963, #43680, #77290, #33595, #66694, #59947, #24091, #103007, #110321, #50982, #59395, #94616, #1140, #101899, #34715, #26304, #60496, #42571, #58279, #25745, #68906, #43132 ),
 .UNSPECIFIED., .F., .F.,
 ( 4, 2, 1, 2, 2, 2, 1, 1, 2, 2, 2, 1, 1, 1, 2, 2, 4 ),
 ( 0.000000000000000000, 0.1249999999999616696, 0.1874999999999424904, 0.2187499999998885059, 0.2499999999998345213, 0.3749999999995644595, 0.4374999999994318434, 0.4687499999993567923, 0.4843749999993692823, 0.4999999999993818278, 0.6249999999998263611, 0.6875000000000558442, 0.7187500000001132427, 0.7343750000001351141, 0.7421875000000797140, 0.7500000000000243139, 1.000000000000000000 ),
 .UNSPECIFIED. ) ;
#68679=CARTESIAN_POINT ( 'NONE',  ( -34.04223167274130191, 1384.566179893659864, 208.0543316770909996 ) ) ;
#68681=CARTESIAN_POINT ( 'NONE',  ( -103.9064370230000094, 1389.684541055990167, 306.7300248541590122 ) ) ;
#68691=CARTESIAN_POINT ( 'NONE',  ( -68.69754074780000508, 1379.747811941090276, 279.9522140925590179 ) ) ;
#68700=CARTESIAN_POINT ( 'NONE',  ( -25.93597669760000102, 1384.979378440369828, 224.2477222537590364 ) ) ;
#68703=CARTESIAN_POINT ( 'NONE',  ( -10.67935949065659962, 1385.309203628900150, 218.7885473373299874 ) ) ;
#68752=CARTESIAN_POINT ( 'NONE',  ( -57.10737429603420168, 1383.800764999470175, 275.4500855170770137 ) ) ;
#68759=CARTESIAN_POINT ( 'NONE',  ( -63.55875838910000653, 1381.694990308149954, 254.4830528533589700 ) ) ;
#68772=CARTESIAN_POINT ( 'NONE',  ( -108.2161777049999927, 1381.376084645610035, 298.2029669646590264 ) ) ;
#68795=CARTESIAN_POINT ( 'NONE',  ( -104.7362624609999955, 1389.320518635239978, 307.7539050006589605 ) ) ;
#68803=CARTESIAN_POINT ( 'NONE',  ( -14.14948096550000045, 1390.186770710789915, 206.8378643784789972 ) ) ;
#68827=CARTESIAN_POINT ( 'NONE',  ( -109.9849338725829995, 1384.911448804600013, 311.4561116875739799 ) ) ;
#68843=CARTESIAN_POINT ( 'NONE',  ( -5.991971352970000275, 1388.626171318960132, 216.9651239126190205 ) ) ;
#68844=CARTESIAN_POINT ( 'NONE',  ( -9.071295794445763505, 1385.910742335272971, 218.5589077471069857 ) ) ;
#68857=VERTEX_POINT ( 'NONE', #53786 ) ;
#68862=CARTESIAN_POINT ( 'NONE',  ( -10.22261203090000059, 1388.971412213310032, 201.9214163269789992 ) ) ;
#68868=CARTESIAN_POINT ( 'NONE',  ( -9.005778233164750901, 1384.117648528409973, 218.5947890724640104 ) ) ;
#68898=CARTESIAN_POINT ( 'NONE',  ( -109.5349683309999875, 1384.900884850210105, 297.1231244331590347 ) ) ;
#68902=CARTESIAN_POINT ( 'NONE',  ( -12.18719547259109959, 1391.620637730509998, 211.5989438970109973 ) ) ;
#68906=CARTESIAN_POINT ( 'NONE',  ( -109.4677423672981575, 1382.863364883987970, 311.1289870959311656 ) ) ;
#68909=CARTESIAN_POINT ( 'NONE',  ( -12.45388125799999912, 1391.576963816120042, 208.7046256454329978 ) ) ;
#68910=CARTESIAN_POINT ( 'NONE',  ( -83.03005440452790253, 1385.169125049510058, 286.7572543505270346 ) ) ;
#68970=CARTESIAN_POINT ( 'NONE',  ( -11.55222382600000053, 1391.913060387289988, 210.8753015047989834 ) ) ;
#68971=CARTESIAN_POINT ( 'NONE',  ( -87.47508722668870007, 1384.828440509849770, 290.8377656053449982 ) ) ;
#68989=CARTESIAN_POINT ( 'NONE',  ( -44.33415861099999944, 1379.660740675520174, 229.4371355697589649 ) ) ;
#68996=ORIENTED_EDGE ( 'NONE', *, *, #58439, .F. ) ;
#69042=CARTESIAN_POINT ( 'NONE',  ( -82.20641648805589341, 1384.634060515750207, 305.2179643079160201 ) ) ;
#69043=CARTESIAN_POINT ( 'NONE',  ( -11.60963209123129936, 1384.935719060559904, 200.1630794765560211 ) ) ;
#69060=CARTESIAN_POINT ( 'NONE',  ( -14.08836401118779946, 1379.655773939669871, 211.5932977078229840 ) ) ;
#69073=CARTESIAN_POINT ( 'NONE',  ( -65.37646396962441031, 1379.739460607499950, 275.4797537947760020 ) ) ;
#69104=CARTESIAN_POINT ( 'NONE',  ( -60.03054239385676993, 1379.724805969880208, 261.4558930067639722 ) ) ;
#69120=CARTESIAN_POINT ( 'NONE',  ( -111.2060435952740676, 1379.913060387289988, 303.0232821107484824 ) ) ;
#69125=CIRCLE ( 'NONE', #11877, 2.000079904907770434 ) ;
#69130=CARTESIAN_POINT ( 'NONE',  ( -102.9162786870000019, 1389.260382295949967, 308.6471719622589944 ) ) ;
#69141=CARTESIAN_POINT ( 'NONE',  ( -107.2549441997609989, 1382.093684753940124, 310.1063884366330399 ) ) ;
#69168=CARTESIAN_POINT ( 'NONE',  ( -14.27824533756169956, 1384.878970200230015, 219.2940513638699827 ) ) ;
#69202=CARTESIAN_POINT ( 'NONE',  ( -9.116411868360000170, 1384.545094513749746, 199.9660485183590026 ) ) ;
#69231=CARTESIAN_POINT ( 'NONE',  ( -79.49322724790000905, 1384.792572819600082, 282.9493281527590511 ) ) ;
#69233=CARTESIAN_POINT ( 'NONE',  ( -58.69053996021689557, 1384.665059837310082, 241.2311621880149914 ) ) ;
#69244=CARTESIAN_POINT ( 'NONE',  ( -68.36039621120001186, 1379.746991223579926, 279.2258544646589939 ) ) ;
#69253=CARTESIAN_POINT ( 'NONE',  ( -32.10879564089999860, 1385.224147136040074, 229.9470470709589733 ) ) ;
#69255=CARTESIAN_POINT ( 'NONE',  ( -105.1514435807109180, 1379.134842035547763, 304.0347158685106024 ) ) ;
#69259=ADVANCED_FACE ( 'NONE', ( #79383 ), #64109, .F. ) ;
#69302=CARTESIAN_POINT ( 'NONE',  ( -55.50846133737319832, 1383.803145790959888, 272.4221409317659663 ) ) ;
#69310=CARTESIAN_POINT ( 'NONE',  ( -84.13119167140000343, 1384.814165098149942, 288.0554183306589948 ) ) ;
#69321=CARTESIAN_POINT ( 'NONE',  ( -107.8318265130000100, 1381.795387502540052, 298.2715083548590087 ) ) ;
#69398=CARTESIAN_POINT ( 'NONE',  ( -13.98236733160000078, 1389.833769007690080, 215.1277130629090095 ) ) ;
#69406=DIRECTION ( 'NONE',  ( -1.000000000000000000, 0.000000000000000000, 0.000000000000000000 ) ) ;
#69431=CARTESIAN_POINT ( 'NONE',  ( -109.1320112420000044, 1384.953741877089897, 311.2644403302589353 ) ) ;
#69436=CARTESIAN_POINT ( 'NONE',  ( -13.49764385317659965, 1383.859966380460037, 218.9859143532220003 ) ) ;
#69444=CARTESIAN_POINT ( 'NONE',  ( -3.148024555753120272E-16, 1383.870885931430166, 218.4497379877689980 ) ) ;
#69449=VERTEX_POINT ( 'NONE', #104802 ) ;
#69450=CARTESIAN_POINT ( 'NONE',  ( -5.789140635075550101, 1391.897372272190069, 203.1891863557009970 ) ) ;
#69451=CARTESIAN_POINT ( 'NONE',  ( -14.47059702760379984, 1380.054458738409949, 208.7831629986500275 ) ) ;
#69460=CARTESIAN_POINT ( 'NONE',  ( -10.81222349729999976, 1391.793768475530214, 204.0084625770589923 ) ) ;
#69461=CARTESIAN_POINT ( 'NONE',  ( -86.45172696223220044, 1385.181189174330257, 290.0270867646340207 ) ) ;
#69487=CARTESIAN_POINT ( 'NONE',  ( -68.75534438227138878, 1379.747886361640212, 280.3294090916749610 ) ) ;
#69517=AXIS2_PLACEMENT_3D ( 'NONE', #88207, #13116, #81423 ) ;
#69520=ADVANCED_FACE ( 'NONE', ( #96964 ), #42795, .T. ) ;
#69524=CARTESIAN_POINT ( 'NONE',  ( -11.97707799540000018, 1391.854779651599983, 210.9632173721890069 ) ) ;
#69525=CARTESIAN_POINT ( 'NONE',  ( -95.05970678514869121, 1384.857596447410060, 294.9623361036900064 ) ) ;
#69598=CARTESIAN_POINT ( 'NONE',  ( -73.71138866091139619, 1384.652804003510028, 298.8779072345359964 ) ) ;
#69599=CARTESIAN_POINT ( 'NONE',  ( -22.04486723005910065, 1384.954349268969963, 202.2380667361449866 ) ) ;
#69606=CARTESIAN_POINT ( 'NONE',  ( -8.156530043329999202, 1384.922241695169760, 199.6468276065789667 ) ) ;
#69616=CARTESIAN_POINT ( 'NONE',  ( -8.515407867320000435, 1383.766919741620086, 199.9370010572289971 ) ) ;
#69630=CARTESIAN_POINT ( 'NONE',  ( -65.86034991249999848, 1379.747388898590089, 276.1189993382589591 ) ) ;
#69638=CARTESIAN_POINT ( 'NONE',  ( -7.769002550049999734, 1384.928845206309916, 218.9178303808890007 ) ) ;
#69654=CARTESIAN_POINT ( 'NONE',  ( -5.013380061527799469, 1375.424024322329842, 203.5256954671220058 ) ) ;
#69664=CARTESIAN_POINT ( 'NONE',  ( -35.67105607187449579, 1379.642165080909763, 218.6247323468043646 ) ) ;
#69672=CARTESIAN_POINT ( 'NONE',  ( -103.9221348808119956, 1379.919223396519783, 305.0512315340399709 ) ) ;
#69682=CARTESIAN_POINT ( 'NONE',  ( -106.4218829409999927, 1384.032086002479900, 311.2287423822589858 ) ) ;
#69696=CARTESIAN_POINT ( 'NONE',  ( -90.54195131439999500, 1389.308449918279848, 306.1970171789590154 ) ) ;
#69707=CARTESIAN_POINT ( 'NONE',  ( -108.0462788022180121, 1381.309336268219795, 310.1032626428960270 ) ) ;
#69762=ORIENTED_EDGE ( 'NONE', *, *, #19247, .T. ) ;
#69787=CARTESIAN_POINT ( 'NONE',  ( -62.88186284109999491, 1379.821258372850025, 270.0876510056589836 ) ) ;
#69795=CARTESIAN_POINT ( 'NONE',  ( -64.59470153520619817, 1384.702257275750071, 254.1534755538610284 ) ) ;
#69807=CARTESIAN_POINT ( 'NONE',  ( -68.69258099389999472, 1379.747741134600119, 279.9541405716590248 ) ) ;
#69816=CARTESIAN_POINT ( 'NONE',  ( -36.12389091449999512, 1385.203813137380166, 235.4649545851590062 ) ) ;
#69818=CARTESIAN_POINT ( 'NONE',  ( -13.54997464361210113, 1385.299760518590119, 219.1450828324119868 ) ) ;
#69859=CARTESIAN_POINT ( 'NONE',  ( -99.18220428064979899, 1383.764529278820191, 310.5488099629289991 ) ) ;
#69869=CARTESIAN_POINT ( 'NONE',  ( -75.43085291519999203, 1383.276795896440035, 276.7272104215589934 ) ) ;
#69880=CARTESIAN_POINT ( 'NONE',  ( -107.5397600339999968, 1382.037659314800067, 298.2264582646590725 ) ) ;
#69891=ORIENTED_EDGE ( 'NONE', *, *, #54816, .T. ) ;
#69896=DIRECTION ( 'NONE',  ( -0.9702683578407158560, 7.674209871302701496E-33, 0.2420316379589265432 ) ) ;
#69943=CARTESIAN_POINT ( 'NONE',  ( -11.39275159694039985, 1391.913060387289988, 207.2216192889670197 ) ) ;
#69946=ORIENTED_EDGE ( 'NONE', *, *, #97295, .F. ) ;
#69954=CARTESIAN_POINT ( 'NONE',  ( -8.976689669389999793, 1389.857300751820048, 214.6605541070490233 ) ) ;
#69964=CARTESIAN_POINT ( 'NONE',  ( -9.153278953699999221, 1381.244387431579980, 217.5834349994690058 ) ) ;
#69994=CARTESIAN_POINT ( 'NONE',  ( -25.46281358831500086, 1383.847540614680156, 223.8241380845890092 ) ) ;
#70004=CARTESIAN_POINT ( 'NONE',  ( -9.920431381559678741, 1389.497472067758736, 201.7143931154362235 ) ) ;
#70011=CARTESIAN_POINT ( 'NONE',  ( -14.38501648843540082, 1380.276608459779936, 209.4261068465210087 ) ) ;
#70019=CARTESIAN_POINT ( 'NONE',  ( -12.25663671779999930, 1391.732016969049937, 208.2029345092809933 ) ) ;
#70020=CARTESIAN_POINT ( 'NONE',  ( -87.98538269667260181, 1385.186294664909838, 291.2263267895870058 ) ) ;
#70101=CARTESIAN_POINT ( 'NONE',  ( -25.94889933050000153, 1379.671554933049947, 211.6347087375590093 ) ) ;
#70121=CARTESIAN_POINT ( 'NONE',  ( -7.544964944700390141, 1384.904325550069871, 219.0876571251629912 ) ) ;
#70155=EDGE_CURVE ( 'NONE', #35724, #66359, #74007, .T. ) ;
#70162=CARTESIAN_POINT ( 'NONE',  ( -75.37878430945180241, 1384.648787239799958, 300.3730460693899431 ) ) ;
#70163=CARTESIAN_POINT ( 'NONE',  ( -23.31512350511849974, 1384.956600135750023, 202.6507508542970015 ) ) ;
#70169=CARTESIAN_POINT ( 'NONE',  ( -5.432410439650000811, 1391.426148861440197, 214.9021618825790085 ) ) ;
#70175=CARTESIAN_POINT ( 'NONE',  ( -106.4081690619180023, 1391.913060387289988, 304.4390516697600333 ) ) ;
#70182=CARTESIAN_POINT ( 'NONE',  ( -12.28864222183389998, 1378.254430273839944, 210.0761076775810068 ) ) ;
#70197=CARTESIAN_POINT ( 'NONE',  ( -60.20344105345110108, 1379.728587437710075, 265.9570968973860090 ) ) ;
#70203=CARTESIAN_POINT ( 'NONE',  ( -105.2302759960000031, 1379.130298687069853, 305.2168657121590059 ) ) ;
#70204=CARTESIAN_POINT ( 'NONE',  ( -109.4839102970000084, 1384.920889589209992, 311.2841191852589873 ) ) ;
#70207=EDGE_CURVE ( 'NONE', #108404, #83875, #68665, .T. ) ;
#70210=CARTESIAN_POINT ( 'NONE',  ( -105.7924919010939959, 1378.913060387289988, 304.1383837694310159 ) ) ;
#70226=CARTESIAN_POINT ( 'NONE',  ( -8.580820927359999573, 1384.944142096140013, 218.6694753803189997 ) ) ;
#70229=CARTESIAN_POINT ( 'NONE',  ( -53.08802174891025061, 1379.700056302278199, 245.9205172436845146 ) ) ;
#70240=CARTESIAN_POINT ( 'NONE',  ( -43.49718241125740548, 1379.669396352335298, 234.1649366570986217 ) ) ;
#70255=CARTESIAN_POINT ( 'NONE',  ( -85.09270623130001354, 1390.599118280639914, 298.7241002662590290 ) ) ;
#70267=CARTESIAN_POINT ( 'NONE',  ( -106.8792834639999967, 1379.710674565020099, 308.6693595243589812 ) ) ;
#70294=CARTESIAN_POINT ( 'NONE',  ( -20.70560609375029770, 1384.860107662629844, 221.2521089292840202 ) ) ;
#70338=ORIENTED_EDGE ( 'NONE', *, *, #25998, .T. ) ;
#70346=CARTESIAN_POINT ( 'NONE',  ( -71.62432531729999141, 1374.712643070490230, 285.2199721836589674 ) ) ;
#70352=CARTESIAN_POINT ( 'NONE',  ( -50.99365685415219929, 1384.624155639869969, 226.8516233277449885 ) ) ;
#70359=CARTESIAN_POINT ( 'NONE',  ( -1.385482440409720093E-15, 1384.214058746219962, 218.5641289260389897 ) ) ;
#70363=CARTESIAN_POINT ( 'NONE',  ( -65.30777065759998834, 1379.749275567730137, 273.2377066393590326 ) ) ;
#70372=CARTESIAN_POINT ( 'NONE',  ( -47.37385164190000353, 1385.009681923870176, 256.2782761542590038 ) ) ;
#70374=CARTESIAN_POINT ( 'NONE',  ( -14.54965318006719954, 1385.296335759480144, 219.3214808617400138 ) ) ;
#70384=CARTESIAN_POINT ( 'NONE',  ( -5.607667144112699731, 1391.799625134960024, 214.9775039132319705 ) ) ;
#70416=CARTESIAN_POINT ( 'NONE',  ( -83.41305439239448560, 1383.774604776039951, 305.6893928593270289 ) ) ;
#70419=CARTESIAN_POINT ( 'NONE',  ( -109.7131932503749994, 1383.420641160820196, 311.2779527788660516 ) ) ;
#70425=CARTESIAN_POINT ( 'NONE',  ( -87.68417812469999717, 1381.021699689639945, 305.9844954027590234 ) ) ;
#70428=ORIENTED_EDGE ( 'NONE', *, *, #42847, .T. ) ;
#70488=B_SPLINE_CURVE_WITH_KNOTS ( 'NONE', 3,
 ( #6243, #75669, #31998, #76209, #74570, #65625, #109813, #83490, #48272, #14642, #92994, #65069, #74017, #24124, #91363, #84596, #100306, #5710, #56665, #49361, #49914, #108706, #48828, #15175, #66186, #82951, #40393, #33092, #24663, #14082, #67281, #23591, #110354, #7887, #99185, #99738, #57780, #66732, #23030, #22464, #6785 ),
 .UNSPECIFIED., .F., .F.,
 ( 4, 2, 2, 1, 1, 2, 2, 2, 1, 1, 1, 2, 2, 2, 1, 1, 2, 2, 2, 2, 2, 2, 2, 4 ),
 ( 0.000000000000000000, 0.06250000000013367085, 0.09375000000022679081, 0.1093750000002732536, 0.1171875000002964018, 0.1210937500003325812, 0.1250000000003687606, 0.1875000000003629319, 0.2187500000003601286, 0.2343750000003837208, 0.2421875000003934908, 0.2460937500003762823, 0.2500000000003590461, 0.3125000000004938272, 0.3437500000005588308, 0.3593750000005890288, 0.3671875000005865308, 0.3750000000005840328, 0.5000000000004931611, 0.6250000000004023448, 0.6875000000003569367, 0.7187500000003310685, 0.7500000000003052003, 1.000000000000000000 ),
 .UNSPECIFIED. ) ;
#70510=CARTESIAN_POINT ( 'NONE',  ( -36.52015904620000697, 1388.283625214549829, 211.0401408952490101 ) ) ;
#70511=FACE_OUTER_BOUND ( 'NONE', #27742, .T. ) ;
#70518=CARTESIAN_POINT ( 'NONE',  ( -8.836665542129999551, 1381.997304831789961, 217.9968222378790017 ) ) ;
#70544=CARTESIAN_POINT ( 'NONE',  ( -29.50517310080210365, 1383.842696339350141, 227.2997455133179869 ) ) ;
#70552=CARTESIAN_POINT ( 'NONE',  ( -8.601711843582590333, 1387.512598758959939, 200.1433781083956660 ) ) ;
#70560=CARTESIAN_POINT ( 'NONE',  ( -13.49218435975080155, 1390.354837178909975, 211.7086340214200106 ) ) ;
#70567=CARTESIAN_POINT ( 'NONE',  ( -96.20702463676329330, 1385.210891181070110, 295.3517524571470290 ) ) ;
#70591=CARTESIAN_POINT ( 'NONE',  ( 3.550311703873260096E-15, 1384.899971913130003, 209.1218459572589836 ) ) ;
#70594=CARTESIAN_POINT ( 'NONE',  ( -103.5801209296959939, 1379.883073482990085, 303.9981235976169955 ) ) ;
#70647=CARTESIAN_POINT ( 'NONE',  ( -110.0494255671617054, 1384.394578747806008, 296.9720231736403662 ) ) ;
#70649=CARTESIAN_POINT ( 'NONE',  ( -30.44593040359999847, 1379.623838566320273, 214.2479615521790208 ) ) ;
#70654=CARTESIAN_POINT ( 'NONE',  ( -21.80201530938867549, 1379.715454459142848, 213.3549729146243976 ) ) ;
#70661=CARTESIAN_POINT ( 'NONE',  ( -56.62033099439780415, 1385.083666504650182, 274.9067868046199692 ) ) ;
#70692=CARTESIAN_POINT ( 'NONE',  ( -9.269106418329268848, 1384.253990364469928, 197.9928380864789972 ) ) ;
#70710=CARTESIAN_POINT ( 'NONE',  ( -78.31511690615438681, 1384.642162581499861, 302.6921158508910139 ) ) ;
#70711=CARTESIAN_POINT ( 'NONE',  ( -45.64952612643359231, 1385.004992914349941, 219.1277060083630204 ) ) ;
#70718=CARTESIAN_POINT ( 'NONE',  ( -8.371048524560000814, 1384.932744135109942, 199.7749417901490006 ) ) ;
#70743=CARTESIAN_POINT ( 'NONE',  ( -67.12659018946959577, 1379.744665315070051, 278.1807872282039966 ) ) ;
#70749=CARTESIAN_POINT ( 'NONE',  ( -105.2954588910000098, 1379.016081903610029, 304.6073168026589997 ) ) ;
#70754=B_SPLINE_CURVE_WITH_KNOTS ( 'NONE', 5,
 ( #4869, #39012, #73190, #59702, #100576, #93814, #84868, #110092, #84334 ),
 .UNSPECIFIED., .F., .F.,
 ( 6, 3, 6 ),
 ( 0.000000000000000000, 0.5677246447800281537, 1.000000000000000000 ),
 .UNSPECIFIED. ) ;
#70768=VERTEX_POINT ( 'NONE', #50846 ) ;
#70774=CARTESIAN_POINT ( 'NONE',  ( -8.023236032950000762, 1384.902848640620050, 218.7875340078090005 ) ) ;
#70777=CARTESIAN_POINT ( 'NONE',  ( -59.10983982511428536, 1379.721706864959515, 259.3694688010850200 ) ) ;
#70789=CARTESIAN_POINT ( 'NONE',  ( -57.28523240820543805, 1379.717557217216381, 260.4048635326923886 ) ) ;
#70810=CARTESIAN_POINT ( 'NONE',  ( -102.7371261779999969, 1386.485993092710032, 311.2182069122590065 ) ) ;
#70822=CARTESIAN_POINT ( 'NONE',  ( -105.6030581432469972, 1377.982187984739994, 305.0819089094490550 ) ) ;
#70828=AXIS2_PLACEMENT_3D ( 'NONE', #52908, #10327, #44500 ) ;
#70849=CARTESIAN_POINT ( 'NONE',  ( -12.73211671072519913, 1384.883120266560127, 219.0473556928539836 ) ) ;
#70869=CARTESIAN_POINT ( 'NONE',  ( 7.513264357029996177, 1375.413060387289988, 209.1218459572589836 ) ) ;
#70870=CARTESIAN_POINT ( 'NONE',  ( -55.15136628130240837, 1379.936376804820156, 253.2598006625759695 ) ) ;
#70880=CARTESIAN_POINT ( 'NONE',  ( -7.587808279129999889, 1384.071260043419898, 219.0277729778390210 ) ) ;
#70901=CARTESIAN_POINT ( 'NONE',  ( -85.54616801760001010, 1375.529499929939902, 296.2627734727589655 ) ) ;
#70903=CARTESIAN_POINT ( 'NONE',  ( -105.8501189142269965, 1378.913060387460064, 303.4887780044520014 ) ) ;
#70907=CARTESIAN_POINT ( 'NONE',  ( -94.50912602849999189, 1384.855827234549906, 294.8620370673590401 ) ) ;
#70915=B_SPLINE_CURVE_WITH_KNOTS ( 'NONE', 5,
 ( #83747, #16511, #100543, #50701, #92693, #25474, #32786, #67525, #15422 ),
 .UNSPECIFIED., .F., .F.,
 ( 6, 3, 6 ),
 ( 0.000000000000000000, 0.4999976322456015643, 1.000000000000000000 ),
 .UNSPECIFIED. ) ;
#70922=CARTESIAN_POINT ( 'NONE',  ( -65.88578210080000019, 1379.740759783769818, 274.2509442001589832 ) ) ;
#70931=CARTESIAN_POINT ( 'NONE',  ( -27.63867464639999838, 1385.244481134689977, 225.6178332698589770 ) ) ;
#70933=CARTESIAN_POINT ( 'NONE',  ( -31.27769646076779964, 1385.227575565290181, 229.4193426744380133 ) ) ;
#70946=EDGE_CURVE ( 'NONE', #42195, #98535, #89934, .T. ) ;
#70977=CARTESIAN_POINT ( 'NONE',  ( -80.19811966763030853, 1383.776841508610005, 303.7771253361019603 ) ) ;
#70978=CARTESIAN_POINT ( 'NONE',  ( -109.0351493388839828, 1384.329153919109785, 311.2187254259250153 ) ) ;
#70984=CARTESIAN_POINT ( 'NONE',  ( -74.66787686629999143, 1381.796287462720102, 277.1868353108590100 ) ) ;
#70989=CARTESIAN_POINT ( 'NONE',  ( -110.0629862560000021, 1384.919307705380106, 296.9512714754590093 ) ) ;
#71062=CARTESIAN_POINT ( 'NONE',  ( -39.76804797110000322, 1384.988983489909742, 212.4493689816489734 ) ) ;
#71063=CARTESIAN_POINT ( 'NONE',  ( -12.56539978307642791, 1389.228131685772041, 215.4313030480873294 ) ) ;
#71070=CARTESIAN_POINT ( 'NONE',  ( -9.599331020219999289, 1381.710107449539919, 217.4672660472789687 ) ) ;
#71099=CARTESIAN_POINT ( 'NONE',  ( -24.69891064529219804, 1383.848419887520095, 223.2892647768329653 ) ) ;
#71107=CARTESIAN_POINT ( 'NONE',  ( -9.240102488050887075, 1388.574724895332793, 200.8464198674274996 ) ) ;
#71113=CARTESIAN_POINT ( 'NONE',  ( -9.428062662729999488, 1388.903456711819899, 217.2485254379789978 ) ) ;
#71119=CARTESIAN_POINT ( 'NONE',  ( -12.29983469507761917, 1377.704127499016067, 208.5802176589124031 ) ) ;
#71123=CARTESIAN_POINT ( 'NONE',  ( -105.1325957748820059, 1385.233345991170154, 296.9340941069459632 ) ) ;
#71146=CARTESIAN_POINT ( 'NONE',  ( -109.1848878950000028, 1384.511724394249995, 297.1380044401590226 ) ) ;
#71158=VERTEX_POINT ( 'NONE', #28129 ) ;
#71208=CARTESIAN_POINT ( 'NONE',  ( -66.72509573152139239, 1385.036337219960160, 291.0918609499310037 ) ) ;
#71243=CARTESIAN_POINT ( 'NONE',  ( -7.765511611824870819, 1383.298095908590085, 218.8630668455809882 ) ) ;
#71262=CARTESIAN_POINT ( 'NONE',  ( -44.00405079680249543, 1385.000270709609822, 217.1257494786190136 ) ) ;
#71263=CARTESIAN_POINT ( 'NONE',  ( -5.013279353751990186, 1375.408587603007163, 214.7179514574215204 ) ) ;
#71269=CARTESIAN_POINT ( 'NONE',  ( -8.604402833090000868, 1384.931574737560140, 199.8686422932590006 ) ) ;
#71276=CIRCLE ( 'NONE', #3320, 12.49965726619999984 ) ;
#71281=CARTESIAN_POINT ( 'NONE',  ( -106.4226887258490137, 1391.913060387289988, 304.6216818903239414 ) ) ;
#71286=CARTESIAN_POINT ( 'NONE',  ( -14.17772863140000084, 1379.591530680210099, 207.8208987399890191 ) ) ;
#71297=CARTESIAN_POINT ( 'NONE',  ( -68.28298542711279140, 1379.746875315909847, 279.8596883230670187 ) ) ;
#71303=CARTESIAN_POINT ( 'NONE',  ( -109.1314240389999952, 1384.941892907230113, 311.2645748072590095 ) ) ;
#71323=EDGE_LOOP ( 'NONE', ( #23860, #82822, #654, #99500 ) ) ;
#71330=CARTESIAN_POINT ( 'NONE',  ( -13.88298926620000096, 1379.761820614679891, 208.2296881040550147 ) ) ;
#71348=FACE_OUTER_BOUND ( 'NONE', #94844, .T. ) ;
#71364=CARTESIAN_POINT ( 'NONE',  ( -94.46405900630000474, 1386.760127987169881, 294.9897091881589972 ) ) ;
#71376=CARTESIAN_POINT ( 'NONE',  ( -106.4468452320000011, 1379.239802504850104, 307.9198481384590309 ) ) ;
#71377=CIRCLE ( 'NONE', #85605, 7.513435694540000043 ) ;
#71401=CARTESIAN_POINT ( 'NONE',  ( -35.39279618899279711, 1384.807458296239929, 234.7559858425150026 ) ) ;
#71428=CARTESIAN_POINT ( 'NONE',  ( -71.62438411370330016, 1379.712643069029809, 285.2199323073880350 ) ) ;
#71440=CARTESIAN_POINT ( 'NONE',  ( -9.129808330190000376, 1383.863787716949901, 218.5279287960690056 ) ) ;
#71444=CARTESIAN_POINT ( 'NONE',  ( -110.0634901748029932, 1384.899971912700039, 296.9512050915229793 ) ) ;
#71464=CARTESIAN_POINT ( 'NONE',  ( -87.79856897099999458, 1374.577971548089863, 299.2711673883590038 ) ) ;
#71479=CARTESIAN_POINT ( 'NONE',  ( -67.99787016330000711, 1379.746136258720071, 278.4829519276589735 ) ) ;
#71487=CARTESIAN_POINT ( 'NONE',  ( -96.24131551039999977, 1384.723465092230072, 310.5839496812590141 ) ) ;
#71489=CARTESIAN_POINT ( 'NONE',  ( -32.15151909282970877, 1385.223364821960104, 230.4497740801809869 ) ) ;
#71502=CARTESIAN_POINT ( 'NONE',  ( -5.433843300390170050, 1391.480867605439926, 214.9027815983120036 ) ) ;
#71538=CARTESIAN_POINT ( 'NONE',  ( -79.35849551933969792, 1383.777447801099925, 303.2169598375339774 ) ) ;
#71539=CARTESIAN_POINT ( 'NONE',  ( -109.6045263617230034, 1384.282720651610134, 311.2785409792999758 ) ) ;
#71544=CARTESIAN_POINT ( 'NONE',  ( -81.53378978499999619, 1382.336709067400079, 304.3954627607590169 ) ) ;
#71626=CARTESIAN_POINT ( 'NONE',  ( -50.84652256599999731, 1385.021217850319999, 226.1755936018590205 ) ) ;
#71627=B_SPLINE_CURVE_WITH_KNOTS ( 'NONE', 3,
 ( #33044, #32512, #20107, #1129, #20640, #11185, #77820, #2249, #10055, #45346, #79485, #36913, #104671, #70552, #27405, #2792, #11718, #44229, #27965, #105794, #71107, #54300, #53183, #88428, #35259, #87893, #70004, #62149, #104118, #78941, #45889, #103561, #54842, #78373, #3347, #63259 ),
 .UNSPECIFIED., .F., .F.,
 ( 4, 2, 2, 1, 1, 1, 2, 2, 2, 2, 1, 1, 1, 2, 2, 2, 2, 1, 1, 2, 2, 4 ),
 ( 0.000000000000000000, 0.1250000000019153013, 0.1875000000029100888, 0.2187500000034410808, 0.2343750000037066461, 0.2421875000038058723, 0.2460937500038569148, 0.2500000000039079295, 0.3750000000046815885, 0.4375000000050380811, 0.4687500000052188254, 0.4843750000053117510, 0.4921875000053556604, 0.4960937500053528848, 0.5000000000053500537, 0.6250000000040984993, 0.6875000000034486858, 0.7187500000031239455, 0.7343750000029616309, 0.7421875000028802516, 0.7500000000027988722, 1.000000000000000000 ),
 .UNSPECIFIED. ) ;
#71632=CARTESIAN_POINT ( 'NONE',  ( -14.08302796437247828, 1379.638023313924123, 211.6372550111867383 ) ) ;
#71665=CARTESIAN_POINT ( 'NONE',  ( -21.05048463384780177, 1383.852467042130229, 221.2200317013300150 ) ) ;
#71674=CARTESIAN_POINT ( 'NONE',  ( -6.004020725660000224, 1380.880730018859822, 216.3710173946490158 ) ) ;
#71681=CARTESIAN_POINT ( 'NONE',  ( -8.680524314125149132, 1387.563194770179962, 218.1353776963400151 ) ) ;
#71691=CARTESIAN_POINT ( 'NONE',  ( -92.68011806984669931, 1385.200888536659932, 294.0055341178320418 ) ) ;
#71693=CARTESIAN_POINT ( 'NONE',  ( -68.43569653030000666, 1379.748342192099926, 279.4446506693590209 ) ) ;
#71700=CIRCLE ( 'NONE', #26893, 7.932410439649999923 ) ;
#71715=CARTESIAN_POINT ( 'NONE',  ( -107.7596963679999931, 1382.859817520469733, 297.6961126062590210 ) ) ;
#71717=CARTESIAN_POINT ( 'NONE',  ( -113.4000000000000057, 1384.913060387289988, 304.2218459572590064 ) ) ;
#71725=CARTESIAN_POINT ( 'NONE',  ( -109.9855944279999989, 1384.926148861439970, 311.4562326602589906 ) ) ;
#71748=ORIENTED_EDGE ( 'NONE', *, *, #96917, .T. ) ;
#71772=CARTESIAN_POINT ( 'NONE',  ( -76.63588753610599724, 1385.003182676139886, 301.4206644342669961 ) ) ;
#71789=FACE_OUTER_BOUND ( 'NONE', #18030, .T. ) ;
#71806=CARTESIAN_POINT ( 'NONE',  ( -7.641220756667040703, 1383.796531935709936, 218.9774033050359776 ) ) ;
#71821=CARTESIAN_POINT ( 'NONE',  ( -39.94094280074159542, 1384.989748394649951, 212.8264697954110147 ) ) ;
#71830=CARTESIAN_POINT ( 'NONE',  ( -109.4849134029999931, 1384.882923838719989, 311.2840634072589978 ) ) ;
#71831=B_SPLINE_CURVE_WITH_KNOTS ( 'NONE', 3,
 ( #65228, #74183, #98805, #81994, #22066, #82572, #5301, #58476, #49531, #92064, #4744, #22614, #73069, #99339, #30498, #31598, #100998, #6410, #74730, #108864, #108314, #38888, #14241, #39459, #65777, #41108, #91517, #107210, #6951, #73632, #90392, #56263, #83656, #56817, #48430, #5864, #23743, #40005, #57931, #99894, #66889, #92604, #75285, #23192, #57391, #109431, #24294, #14797, #48983, #32157, #15877, #50080 ),
 .UNSPECIFIED., .F., .F.,
 ( 4, 2, 2, 1, 1, 2, 2, 2, 2, 1, 1, 2, 2, 2, 1, 1, 1, 2, 2, 2, 1, 1, 2, 2, 2, 1, 2, 2, 2, 2, 4 ),
 ( 0.000000000000000000, 0.06249999999934317818, 0.09374999999905359038, 0.1093749999989083177, 0.1171874999988343352, 0.1210937499987959215, 0.1249999999987574939, 0.1874999999981092347, 0.2187499999977872700, 0.2343749999976272314, 0.2421874999975472120, 0.2460937499974766018, 0.2499999999974060194, 0.3124999999966770470, 0.3437499999963145592, 0.3593749999961312058, 0.3671874999960428876, 0.3710937499960308972, 0.3749999999960189623, 0.4374999999965382136, 0.4687499999967978392, 0.4843749999968984254, 0.4921874999969200748, 0.4999999999969416686, 0.5624999999973839815, 0.5937499999976038056, 0.6093749999977137177, 0.6249999999978236298, 0.6874999999981920018, 0.7499999999985602628, 1.000000000000000000 ),
 .UNSPECIFIED. ) ;
#71838=CARTESIAN_POINT ( 'NONE',  ( -106.4502107925090115, 1391.913060387289988, 304.8668619185630178 ) ) ;
#71855=CARTESIAN_POINT ( 'NONE',  ( -68.33529581026429867, 1379.747047273969883, 279.8915150897229864 ) ) ;
#71886=CARTESIAN_POINT ( 'NONE',  ( -12.62971280459999868, 1379.172876932190093, 208.6065707151580000 ) ) ;
#71887=CARTESIAN_POINT ( 'NONE',  ( -63.86443237624047953, 1379.736326793258058, 269.9080968292980742 ) ) ;
#71916=CARTESIAN_POINT ( 'NONE',  ( -113.4000000000000057, 1389.425727822280123, 300.1302024219590407 ) ) ;
#71930=CARTESIAN_POINT ( 'NONE',  ( -106.1419745320000061, 1379.261221625959934, 307.4042368804589955 ) ) ;
#71931=ORIENTED_EDGE ( 'NONE', *, *, #65263, .F. ) ;
#71951=CARTESIAN_POINT ( 'NONE',  ( -40.62633303070520441, 1384.784726197159898, 243.2388129929060199 ) ) ;
#71968=CARTESIAN_POINT ( 'NONE',  ( -109.9864287870510111, 1384.705349330230092, 311.4509910198939906 ) ) ;
#71973=CARTESIAN_POINT ( 'NONE',  ( -66.39852830834199438, 1377.354015942380101, 281.9312505627179917 ) ) ;
#71975=CARTESIAN_POINT ( 'NONE',  ( -14.03937168550959846, 1379.585977840610212, 211.7499898191520344 ) ) ;
#71982=CARTESIAN_POINT ( 'NONE',  ( -7.946775756959999271, 1383.555175293329967, 218.7288224669989916 ) ) ;
#71995=ORIENTED_EDGE ( 'NONE', *, *, #34372, .T. ) ;
#72004=CARTESIAN_POINT ( 'NONE',  ( -68.69226509189999774, 1379.746858117560123, 280.5557816734590233 ) ) ;
#72009=CARTESIAN_POINT ( 'NONE',  ( -113.4000000000000057, 1384.913060387289988, 297.2218459572590064 ) ) ;
#72015=CARTESIAN_POINT ( 'NONE',  ( -22.68421185029999876, 1384.517311655589992, 222.0365106238589874 ) ) ;
#72021=CARTESIAN_POINT ( 'NONE',  ( -67.97548607400000265, 1379.747377450629983, 278.4939589122589609 ) ) ;
#72031=CARTESIAN_POINT ( 'NONE',  ( -102.7367842069999995, 1384.710423195750082, 311.2303077692589568 ) ) ;
#72034=CARTESIAN_POINT ( 'NONE',  ( -22.02211068124400128, 1385.268219036880055, 221.8684547256000030 ) ) ;
#72065=CARTESIAN_POINT ( 'NONE',  ( -103.6168536339999946, 1379.900079317219934, 303.2097866628589600 ) ) ;
#72078=CARTESIAN_POINT ( 'NONE',  ( -81.02254885351089797, 1383.776253998839820, 304.3069785600009709 ) ) ;
#72079=CARTESIAN_POINT ( 'NONE',  ( -109.2306744385840034, 1383.829459731100087, 311.1332719636980073 ) ) ;
#72083=CARTESIAN_POINT ( 'NONE',  ( -102.9989294650000033, 1380.111416001630232, 307.4955441714590165 ) ) ;
#72103=EDGE_CURVE ( 'NONE', #59489, #67300, #85888, .T. ) ;
#72122=ORIENTED_EDGE ( 'NONE', *, *, #1915, .F. ) ;
#72162=CARTESIAN_POINT ( 'NONE',  ( -9.104488409295518281, 1384.623999641839873, 199.9569213373260084 ) ) ;
#72166=CARTESIAN_POINT ( 'NONE',  ( -14.08142637225379978, 1379.709117121690042, 211.5303641152310092 ) ) ;
#72185=CARTESIAN_POINT ( 'NONE',  ( -109.1643725169999897, 1385.128571951890081, 297.1381730982590170 ) ) ;
#72188=EDGE_CURVE ( 'NONE', #33248, #78937, #4388, .T. ) ;
#72196=CARTESIAN_POINT ( 'NONE',  ( -26.26504494448730043, 1383.846605286560134, 224.4265172497430001 ) ) ;
#72203=CARTESIAN_POINT ( 'NONE',  ( -36.40844407859999876, 1381.507950937409987, 211.1775457167789796 ) ) ;
#72209=CARTESIAN_POINT ( 'NONE',  ( -9.849592119879998720, 1390.061260120649877, 216.6447051224889719 ) ) ;
#72218=CARTESIAN_POINT ( 'NONE',  ( -97.56006093131890111, 1385.214537156219876, 295.7380020258559625 ) ) ;
#72220=CARTESIAN_POINT ( 'NONE',  ( -68.70865610920000677, 1379.748126065489942, 280.0489821606589658 ) ) ;
#72237=CARTESIAN_POINT ( 'NONE',  ( -8.305981014989999522, 1385.249635131719970, 218.6869742267090260 ) ) ;
#72241=ORIENTED_EDGE ( 'NONE', *, *, #15349, .F. ) ;
#72287=CARTESIAN_POINT ( 'NONE',  ( -105.9720658651419996, 1391.644115899230201, 306.2957621946390532 ) ) ;
#72288=CARTESIAN_POINT ( 'NONE',  ( -60.26586262694746665, 1379.746226297675776, 265.9249327382016190 ) ) ;
#72295=CARTESIAN_POINT ( 'NONE',  ( -78.30924043174148608, 1384.998499083409797, 302.6966419283749588 ) ) ;
#72344=CARTESIAN_POINT ( 'NONE',  ( -90.41991271562498866, 1384.618437443740049, 308.8387648450170104 ) ) ;
#72345=CARTESIAN_POINT ( 'NONE',  ( -46.00916994163010543, 1385.006067563419947, 219.5881877202340036 ) ) ;
#72362=CARTESIAN_POINT ( 'NONE',  ( -12.04010205419999835, 1379.345554316609878, 205.4175452398490052 ) ) ;
#72375=CARTESIAN_POINT ( 'NONE',  ( -68.07056945215670396, 1379.746976000390077, 279.5289119377829934 ) ) ;
#72382=CARTESIAN_POINT ( 'NONE',  ( -109.8255548870000098, 1384.923179268330159, 311.3807808352589745 ) ) ;
#72395=CARTESIAN_POINT ( 'NONE',  ( -11.15738487964140013, 1390.939238811560017, 203.8452351040699853 ) ) ;
#72402=CARTESIAN_POINT ( 'NONE',  ( -8.298029079490001791, 1384.907497196539907, 218.7036230386890168 ) ) ;
#72404=CARTESIAN_POINT ( 'NONE',  ( -68.56305339912407248, 1379.747553719651478, 279.6255597516078524 ) ) ;
#72409=CARTESIAN_POINT ( 'NONE',  ( -58.01177053069230283, 1384.661045340669943, 239.8217497119959773 ) ) ;
#72439=CARTESIAN_POINT ( 'NONE',  ( -8.604462330509999646, 1384.894731729009891, 199.8686916664790090 ) ) ;
#72454=CIRCLE ( 'NONE', #86732, 2.000015581134258369 ) ;
#72460=PLANE ( 'NONE',  #84192 ) ;
#72472=CARTESIAN_POINT ( 'NONE',  ( -30.22200536124639925, 1384.827631819069893, 228.2875610643100117 ) ) ;
#72473=CARTESIAN_POINT ( 'NONE',  ( -105.7666966480000070, 1378.955190987910100, 302.3809606587589656 ) ) ;
#72494=CARTESIAN_POINT ( 'NONE',  ( -94.35249819378030622, 1379.531630662760108, 302.8770685251070631 ) ) ;
#72505=CARTESIAN_POINT ( 'NONE',  ( -8.445660594239999597, 1383.900183497409898, 218.5659211283389993 ) ) ;
#72524=CARTESIAN_POINT ( 'NONE',  ( -12.31497494632570167, 1378.366662294749858, 209.7019801924109856 ) ) ;
#72528=CARTESIAN_POINT ( 'NONE',  ( -29.63091391959999754, 1375.535769174380221, 213.7170380704389743 ) ) ;
#72532=EDGE_LOOP ( 'NONE', ( #67991, #68197, #67563, #31821, #37393 ) ) ;
#72545=CARTESIAN_POINT ( 'NONE',  ( -68.16069380650000653, 1379.746470013149974, 278.7868268744589955 ) ) ;
#72554=CARTESIAN_POINT ( 'NONE',  ( -113.4000000000000057, 1384.913060387289988, 311.2218459572590064 ) ) ;
#72556=CARTESIAN_POINT ( 'NONE',  ( -29.95569946650590154, 1385.233789043189745, 227.9819273993630020 ) ) ;
#72583=CARTESIAN_POINT ( 'NONE',  ( -104.4930758389999994, 1390.118383696849833, 304.1821339162590334 ) ) ;
#72611=CARTESIAN_POINT ( 'NONE',  ( -109.5347599920000050, 1384.912562451920166, 297.1230869496590117 ) ) ;
#72612=CARTESIAN_POINT ( 'NONE',  ( -8.431440857724776805, 1382.698224402347705, 199.9722048618648955 ) ) ;
#72640=B_SPLINE_CURVE_WITH_KNOTS ( 'NONE', 3,
 ( #83945, #33521, #25123, #100729, #58756, #24014, #58211, #67722, #49815, #7245, #92337, #15609, #41406, #101830, #93438, #24565, #32980, #75573, #101269, #16168, #84497, #11126, #104057, #69943, #86157, #78308, #43062, #96218, #19495, #26800, #25677, #36858, #17816, #53697, #77222, #2737, #102394, #8881, #78883, #45285, #44733, #60987, #87265, #44170, #95113, #36302 ),
 .UNSPECIFIED., .F., .F.,
 ( 4, 3, 3, 3, 3, 3, 3, 3, 3, 3, 3, 3, 3, 3, 3, 4 ),
 ( 0.000000000000000000, 0.8425732785457979990, 1.714272507910759913, 2.605598717659390218, 3.529198674031960081, 3.734573540650000023, 4.706518334241139634, 5.735038120595219446, 6.516940428549999886, 7.557162126475709840, 8.512610629112849381, 9.373333392597750446, 9.468059131749999580, 10.28051844247830005, 11.05372975085490062, 11.47905148820000143 ),
 .UNSPECIFIED. ) ;
#72657=ORIENTED_EDGE ( 'NONE', *, *, #49792, .F. ) ;
#72663=CARTESIAN_POINT ( 'NONE',  ( -16.77637052012299890, 1384.526196172110076, 200.9536932091479855 ) ) ;
#72669=ORIENTED_EDGE ( 'NONE', *, *, #6343, .T. ) ;
#72713=CARTESIAN_POINT ( 'NONE',  ( -105.1761031979999927, 1379.258906148879987, 302.7941945437589766 ) ) ;
#72721=EDGE_CURVE ( 'NONE', #66491, #82014, #81686, .T. ) ;
#72727=CARTESIAN_POINT ( 'NONE',  ( -42.48766164769039477, 1383.824249582309903, 246.2945377681980119 ) ) ;
#72736=CARTESIAN_POINT ( 'NONE',  ( -14.94466045259999909, 1378.908932901829985, 209.1574112226180091 ) ) ;
#72742=CARTESIAN_POINT ( 'NONE',  ( -10.18804078449999828, 1389.424862935219835, 216.4200518291889921 ) ) ;
#72743=CARTESIAN_POINT ( 'NONE',  ( -9.809994025999090539, 1391.913060387289988, 214.8154631801960193 ) ) ;
#72752=CARTESIAN_POINT ( 'NONE',  ( -68.77278092737650184, 1379.747928288920093, 280.3133413970129482 ) ) ;
#72766=CARTESIAN_POINT ( 'NONE',  ( -109.8365661610000075, 1385.307778176620104, 311.3803512332590344 ) ) ;
#72777=CARTESIAN_POINT ( 'NONE',  ( -7.780674843099999904, 1385.361898457490042, 218.8940646902889853 ) ) ;
#72799=CARTESIAN_POINT ( 'NONE',  ( -3.078458355069999985, 1384.494027187519805, 199.6978503428690033 ) ) ;
#72830=CARTESIAN_POINT ( 'NONE',  ( -40.81304585798746842, 1379.731884792838628, 229.1715070870794762 ) ) ;
#72837=CARTESIAN_POINT ( 'NONE',  ( -90.81899498049169495, 1384.967630141919926, 308.9748035079580291 ) ) ;
#72838=CARTESIAN_POINT ( 'NONE',  ( -8.480130668890000223, 1385.259995920419897, 199.8152338849189675 ) ) ;
#72877=CARTESIAN_POINT ( 'NONE',  ( -5.000000000000000000, 1374.913060387289988, 209.1218459572589836 ) ) ;
#72880=CARTESIAN_POINT ( 'NONE',  ( -12.29056600139999844, 1378.273160383739878, 210.0576833531530099 ) ) ;
#72881=CARTESIAN_POINT ( 'NONE',  ( -92.43963088858200194, 1384.614736519750068, 309.4282936136820013 ) ) ;
#72882=CARTESIAN_POINT ( 'NONE',  ( -37.45666113624130134, 1384.983989573890085, 210.6155393482590057 ) ) ;
#72914=CARTESIAN_POINT ( 'NONE',  ( -67.59948389071639951, 1379.746398059029843, 278.8592533132159588 ) ) ;
#72934=ORIENTED_EDGE ( 'NONE', *, *, #34393, .F. ) ;
#72942=CARTESIAN_POINT ( 'NONE',  ( -12.31949146110000015, 1378.253793539069875, 209.5105131724709793 ) ) ;
#72943=CARTESIAN_POINT ( 'NONE',  ( -68.76678092981147472, 1379.747948897872448, 280.1164399018334166 ) ) ;
#72949=CARTESIAN_POINT ( 'NONE',  ( -52.54124001031040336, 1384.631524148350081, 229.4357186639910253 ) ) ;
#72950=EDGE_LOOP ( 'NONE', ( #63986, #101764, #13765, #22200 ) ) ;
#72957=CARTESIAN_POINT ( 'NONE',  ( -111.2060435952740676, 1379.013060387289897, 303.0232821107484824 ) ) ;
#72977=CARTESIAN_POINT ( 'NONE',  ( -106.5907474589999993, 1390.522254817180055, 304.4566592667590044 ) ) ;
#73006=CARTESIAN_POINT ( 'NONE',  ( -105.5460821599999974, 1391.484866075830041, 304.2071864700581614 ) ) ;
#73015=CARTESIAN_POINT ( 'NONE',  ( -37.93199094438229935, 1384.796719469609798, 238.6434350429059918 ) ) ;
#73039=CARTESIAN_POINT ( 'NONE',  ( -57.85321423391380335, 1379.895658627149942, 259.2190435032479741 ) ) ;
#73041=CARTESIAN_POINT ( 'NONE',  ( -14.01382144633140037, 1379.590371145329982, 211.9185990975750258 ) ) ;
#73042=EDGE_LOOP ( 'NONE', ( #23188, #84834, #25109, #11538 ) ) ;
#73051=CARTESIAN_POINT ( 'NONE',  ( -7.724153670609999800, 1383.436097328069991, 218.9006927288590134 ) ) ;
#73069=CARTESIAN_POINT ( 'NONE',  ( -109.7582210444096802, 1386.278646697699969, 311.3050739296813845 ) ) ;
#73072=CARTESIAN_POINT ( 'NONE',  ( -14.43834517638610038, 1380.180499307529999, 209.0320278544499786 ) ) ;
#73073=AXIS2_PLACEMENT_3D ( 'NONE', #63815, #99028, #108549 ) ;
#73077=CARTESIAN_POINT ( 'NONE',  ( -52.12027059500000092, 1379.080878082759909, 241.5351867017590166 ) ) ;
#73089=CARTESIAN_POINT ( 'NONE',  ( -81.22608496769998965, 1384.058471608169839, 304.8846490667589819 ) ) ;
#73094=CARTESIAN_POINT ( 'NONE',  ( -60.11231289889999374, 1379.722095685149952, 261.7638568618589829 ) ) ;
#73104=CARTESIAN_POINT ( 'NONE',  ( -28.14421679356709660, 1385.242063718970030, 226.2112307642150029 ) ) ;
#73128=CARTESIAN_POINT ( 'NONE',  ( -103.5631853459999974, 1389.967198823729859, 302.9633942972590148 ) ) ;
#73130=CARTESIAN_POINT ( 'NONE',  ( -106.4806709740000059, 1391.913060444069970, 302.1193611446589671 ) ) ;
#73134=FACE_OUTER_BOUND ( 'NONE', #98363, .T. ) ;
#73138=DIRECTION ( 'NONE',  ( 6.360620485575798415E-17, 1.000000000000000000, -8.754643039332639448E-17 ) ) ;
#73144=AXIS2_PLACEMENT_3D ( 'NONE', #27782, #68163, #33968 ) ;
#73157=CARTESIAN_POINT ( 'NONE',  ( -109.1646038599999997, 1384.934474657399960, 297.1326231125589743 ) ) ;
#73158=CARTESIAN_POINT ( 'NONE',  ( -11.66675062582269895, 1378.331411511049055, 205.1377757328165785 ) ) ;
#73190=CARTESIAN_POINT ( 'NONE',  ( -11.73107767829999837, 1391.121393030069839, 205.1223722441990276 ) ) ;
#73200=B_SPLINE_SURFACE_WITH_KNOTS ( 'NONE', 5, 5, ( 
 ( #12108, #19953, #46301, #97765, #21037, #72583, #21593, #22131, #38948 ),
 ( #90462, #22684, #4803, #13188, #49591, #89914, #56883, #82632, #73128 ),
 ( #64192, #74791, #13739, #98314, #57992, #92126, #49044, #39524, #56330 ),
 ( #15402, #47923, #30565, #40620, #66403, #55798, #108934, #6470, #47376 ),
 ( #32222, #14303, #23801, #57453, #40070, #82059, #107270, #91014, #91580 ),
 ( #30001, #106711, #48493, #81501, #5924, #74249, #64755, #100522, #98866 ),
 ( #5364, #83723, #73699, #107825, #31113, #14853, #65293, #99406, #108380 ),
 ( #31662, #83180, #7018, #65842, #41175, #99961, #23254, #101058, #299 ),
 ( #58542, #84810, #68056, #50146, #24356, #101605, #7568, #15945, #59097 ),
 ( #84273, #92668, #18163, #41723, #25448, #51227, #75883, #33865, #32766 ),
 ( #93221, #66949, #26567, #60763, #17593, #8109, #24890, #110031, #94886 ),
 ( #9235, #34971, #33306, #77542, #85932, #67501, #42276, #846, #93752 ) ),
 .UNSPECIFIED., .F., .F., .F.,
 ( 6, 3, 3, 6 ),
 ( 6, 3, 6 ),
 ( 29.56117038800000074, 40.55923757500000448, 46.18177991610000532, 51.15186658319999680 ),
 ( 0.000000000000000000, 1.000000000000000000, 2.000000000000000000 ),
 .UNSPECIFIED. ) ;
#73206=CARTESIAN_POINT ( 'NONE',  ( -18.50881575315199967, 1384.530072707220143, 201.3187559258710166 ) ) ;
#73231=B_SPLINE_CURVE_WITH_KNOTS ( 'NONE', 5,
 ( #38265, #39376, #108227, #55653, #20903, #13045 ),
 .UNSPECIFIED., .F., .F.,
 ( 6, 6 ),
 ( -1.999999915403020134, 0.000000000000000000 ),
 .UNSPECIFIED. ) ;
#73238=CARTESIAN_POINT ( 'NONE',  ( -14.06292235172921679, 1379.592324727026835, 211.7786485450617135 ) ) ;
#73254=ADVANCED_FACE ( 'NONE', ( #100063 ), #86619, .F. ) ;
#73269=CARTESIAN_POINT ( 'NONE',  ( -52.39341264816799537, 1383.808018661449978, 266.2425820643259726 ) ) ;
#73280=CARTESIAN_POINT ( 'NONE',  ( -14.07327828060000030, 1379.838870826219818, 214.5512279352489884 ) ) ;
#73286=PRODUCT_DEFINITION_SHAPE ( 'NONE', 'NONE',  #41841 ) ;
#73288=CARTESIAN_POINT ( 'NONE',  ( -11.63740560221349973, 1390.801072237219842, 213.8478914447200054 ) ) ;
#73303=VERTEX_POINT ( 'NONE', #55480 ) ;
#73311=CARTESIAN_POINT ( 'NONE',  ( -109.1427469879999990, 1386.396569596549853, 311.0572058512590274 ) ) ;
#73320=CARTESIAN_POINT ( 'NONE',  ( -8.579394357329999110, 1384.984320043210118, 218.6689291461190123 ) ) ;
#73342=CARTESIAN_POINT ( 'NONE',  ( -23.00221949109999997, 1384.956020836430071, 202.3857052141389943 ) ) ;
#73350=DIRECTION ( 'NONE',  ( 1.000000000000000000, 0.000000000000000000, 0.000000000000000000 ) ) ;
#73375=CARTESIAN_POINT ( 'NONE',  ( -106.0930553259309903, 1391.335640847810055, 307.0497040399930029 ) ) ;
#73384=CARTESIAN_POINT ( 'NONE',  ( -81.83538110834038548, 1384.989206256060015, 305.0088236927869616 ) ) ;
#73386=CARTESIAN_POINT ( 'NONE',  ( -10.77443953700000101, 1387.520226337789836, 201.1700256806890081 ) ) ;
#73427=CARTESIAN_POINT ( 'NONE',  ( -104.5246723904855770, 1380.568180134393060, 307.6284135004361247 ) ) ;
#73435=CARTESIAN_POINT ( 'NONE',  ( -86.83071232126310690, 1384.625104402849956, 307.5136755095109606 ) ) ;
#73436=CARTESIAN_POINT ( 'NONE',  ( -60.12142991202459541, 1385.061945964109782, 244.2500411141640200 ) ) ;
#73449=CARTESIAN_POINT ( 'NONE',  ( -109.8265548189999947, 1384.687384907379965, 311.3749632952589650 ) ) ;
#73469=CARTESIAN_POINT ( 'NONE',  ( -67.66759637757709811, 1379.745741269309974, 278.9788985089999755 ) ) ;
#73481=CARTESIAN_POINT ( 'NONE',  ( -107.3025753749169979, 1378.913060387289988, 307.5931263302900334 ) ) ;
#73501=CARTESIAN_POINT ( 'NONE',  ( -13.15516956290000117, 1379.513185268939878, 208.2695793243090066 ) ) ;
#73506=CARTESIAN_POINT ( 'NONE',  ( -68.27866047183589160, 1384.726245259990037, 262.2716603733960028 ) ) ;
#73538=CARTESIAN_POINT ( 'NONE',  ( -8.604696469749999466, 1384.902331291159953, 199.8686668561790043 ) ) ;
#73579=CARTESIAN_POINT ( 'NONE',  ( -30.81915246055419999, 1384.825406036370168, 228.9375977134340019 ) ) ;
#73589=VERTEX_POINT ( 'NONE', #71444 ) ;
#73603=CARTESIAN_POINT ( 'NONE',  ( -18.52790950258529890, 1380.296293541789964, 211.3290533409030161 ) ) ;
#73632=CARTESIAN_POINT ( 'NONE',  ( -108.9682439114556729, 1387.781254760463980, 310.7917411045218046 ) ) ;
#73634=CARTESIAN_POINT ( 'NONE',  ( -14.51820269904870031, 1379.827956527899914, 208.4132882441429899 ) ) ;
#73639=CARTESIAN_POINT ( 'NONE',  ( -57.14396137519999286, 1379.007173132990147, 252.3469708262589961 ) ) ;
#73651=CARTESIAN_POINT ( 'NONE',  ( -47.53302541269999892, 1383.816002435690052, 256.2046081452590442 ) ) ;
#73657=CARTESIAN_POINT ( 'NONE',  ( -47.71314244639999913, 1379.676121073949844, 235.3060314611589945 ) ) ;
#73666=B_SPLINE_CURVE_WITH_KNOTS ( 'NONE', 3,
 ( #21081, #37920, #30607, #39562, #54189, #80471 ),
 .UNSPECIFIED., .F., .F.,
 ( 4, 2, 4 ),
 ( 0.000000000000000000, 0.5000000000000000000, 1.000000000000000000 ),
 .UNSPECIFIED. ) ;
#73667=CARTESIAN_POINT ( 'NONE',  ( -22.78935994269999910, 1386.920570514349947, 221.8588691826589923 ) ) ;
#73669=CARTESIAN_POINT ( 'NONE',  ( -42.71391872090229924, 1385.166217023060199, 247.0682200317750130 ) ) ;
#73699=CARTESIAN_POINT ( 'NONE',  ( -108.1293204100000054, 1388.564942467859964, 298.2680007914589737 ) ) ;
#73701=FACE_OUTER_BOUND ( 'NONE', #891, .T. ) ;
#73704=CARTESIAN_POINT ( 'NONE',  ( -104.2332084890000061, 1379.842145981129988, 303.2776814956590101 ) ) ;
#73715=CARTESIAN_POINT ( 'NONE',  ( -108.6616353267809956, 1383.758284946439971, 311.0749865448200353 ) ) ;
#73721=CARTESIAN_POINT ( 'NONE',  ( -90.90849950880000563, 1380.088580609059818, 305.1544273986589815 ) ) ;
#73751=CARTESIAN_POINT ( 'NONE',  ( -8.846465147500001791, 1384.759259630609904, 199.9281972367089963 ) ) ;
#73766=AXIS2_PLACEMENT_3D ( 'NONE', #84920, #102279, #41287 ) ;
#73772=CARTESIAN_POINT ( 'NONE',  ( -14.32917876877730023, 1384.520675589830034, 200.5334063978870063 ) ) ;
#73781=CARTESIAN_POINT ( 'NONE',  ( -13.53579909870000009, 1380.123783341879971, 205.1599962651189912 ) ) ;
#73785=CARTESIAN_POINT ( 'NONE',  ( -68.78265774330000681, 1379.747948328889834, 280.2440287133589436 ) ) ;
#73819=CARTESIAN_POINT ( 'NONE',  ( -109.1507334230530120, 1385.214303402609858, 297.1444598211750190 ) ) ;
#73820=EDGE_CURVE ( 'NONE', #59489, #82014, #58813, .T. ) ;
#73835=CARTESIAN_POINT ( 'NONE',  ( -41.78068117807720228, 1383.825374438059953, 244.9784035970620266 ) ) ;
#73843=CARTESIAN_POINT ( 'NONE',  ( -31.25669922000000156, 1381.487600021890103, 207.4386042761090039 ) ) ;
#73849=CARTESIAN_POINT ( 'NONE',  ( -7.798852395605240240, 1385.469439152710038, 218.8921415146500067 ) ) ;
#73853=CARTESIAN_POINT ( 'NONE',  ( -105.1998544249999981, 1380.198630363649954, 300.9198567136589872 ) ) ;
#73869=CARTESIAN_POINT ( 'NONE',  ( -108.8231103770000061, 1386.831205869259975, 310.8600928752589425 ) ) ;
#73895=CARTESIAN_POINT ( 'NONE',  ( -107.7635570413719961, 1378.913060387369796, 300.2373514716429668 ) ) ;
#73901=CARTESIAN_POINT ( 'NONE',  ( -6.354804813069999447, 1384.643210436399841, 199.7268052247689809 ) ) ;
#73924=CARTESIAN_POINT ( 'NONE',  ( -109.0753561177834285, 1382.030600553431668, 297.5814012535014967 ) ) ;
#73928=CARTESIAN_POINT ( 'NONE',  ( -106.4049054108890004, 1391.248032509690120, 307.7491839806990015 ) ) ;
#73935=CARTESIAN_POINT ( 'NONE',  ( -94.05214484065579938, 1384.960168895200013, 309.8416638810129484 ) ) ;
#73936=CARTESIAN_POINT ( 'NONE',  ( -9.216856378879999312, 1385.697103985929971, 200.0334226857090130 ) ) ;
#73949=CARTESIAN_POINT ( 'NONE',  ( -107.0452211441419621, 1390.407136375272330, 299.6009371605423439 ) ) ;
#73974=CARTESIAN_POINT ( 'NONE',  ( -108.4397519767807552, 1383.495406804093136, 310.9866756129748069 ) ) ;
#73981=CARTESIAN_POINT ( 'NONE',  ( -13.67445017210000024, 1380.322169305999978, 210.0770191355990164 ) ) ;
#73983=CARTESIAN_POINT ( 'NONE',  ( -51.00415357460500587, 1385.022678461219812, 226.8415894493760163 ) ) ;
#73995=CARTESIAN_POINT ( 'NONE',  ( -109.6606343030000090, 1384.812795754960007, 311.3218902852589736 ) ) ;
#73996=DIRECTION ( 'NONE',  ( 1.439455173507210273E-14, 1.000000000000000000, 2.465190328815660140E-31 ) ) ;
#74007=B_SPLINE_CURVE_WITH_KNOTS ( 'NONE', 3,
 ( #108109, #108669, #39818, #40908 ),
 .UNSPECIFIED., .F., .F.,
 ( 4, 4 ),
 ( 29.60747119820000250, 29.67279265790000053 ),
 .UNSPECIFIED. ) ;
#74009=CARTESIAN_POINT ( 'NONE',  ( -5.023678250220539709, 1375.295974637168456, 203.5210896577872859 ) ) ;
#74014=CARTESIAN_POINT ( 'NONE',  ( -68.54059710952350315, 1379.747571644130176, 280.1307283583089998 ) ) ;
#74017=CARTESIAN_POINT ( 'NONE',  ( -8.417565570956876186, 1381.789049435770949, 218.2528661022787162 ) ) ;
#74027=CARTESIAN_POINT ( 'NONE',  ( -107.1098322795840119, 1378.913060387289988, 307.3359821571719976 ) ) ;
#74039=CIRCLE ( 'NONE', #107978, 7.999657266239995401 ) ;
#74046=CARTESIAN_POINT ( 'NONE',  ( -14.49997346389999997, 1379.670736723790014, 208.2214565508510020 ) ) ;
#74052=CARTESIAN_POINT ( 'NONE',  ( -67.67528647966889821, 1384.722340586130031, 260.9666397543829817 ) ) ;
#74064=EDGE_CURVE ( 'NONE', #61100, #53370, #42990, .T. ) ;
#74091=CARTESIAN_POINT ( 'NONE',  ( -66.58099742339999239, 1379.774555183159919, 276.6312621969589713 ) ) ;
#74122=DIRECTION ( 'NONE',  ( 0.01258894674767200433, 0.9999149092275962936, 0.003419462553138305841 ) ) ;
#74124=CARTESIAN_POINT ( 'NONE',  ( -53.35900147057170528, 1384.724215327180218, 268.5776327521460303 ) ) ;
#74125=CARTESIAN_POINT ( 'NONE',  ( -106.7981877087919997, 1391.913060387289988, 302.1811662082889711 ) ) ;
#74136=EDGE_LOOP ( 'NONE', ( #37139, #14961, #85029, #91177, #58286, #22787 ) ) ;
#74153=CARTESIAN_POINT ( 'NONE',  ( -28.76043848733170094, 1380.228231663270208, 215.0391681145920018 ) ) ;
#74183=CARTESIAN_POINT ( 'NONE',  ( -109.9907908981719231, 1385.097515532879925, 311.4537231510988136 ) ) ;
#74185=CARTESIAN_POINT ( 'NONE',  ( -13.76314899857599983, 1380.295045644700167, 209.3459254739570099 ) ) ;
#74186=ADVANCED_FACE ( 'NONE', ( #103297 ), #25775, .F. ) ;
#74192=CARTESIAN_POINT ( 'NONE',  ( -29.63091391959999754, 1379.920694154159946, 213.7170380699990062 ) ) ;
#74205=CARTESIAN_POINT ( 'NONE',  ( -32.09555170170000338, 1384.821019989420165, 229.9571600258589967 ) ) ;
#74212=AXIS2_PLACEMENT_3D ( 'NONE', #72877, #39817, #13482 ) ;
#74222=CARTESIAN_POINT ( 'NONE',  ( -39.64020011839999569, 1388.419118112470187, 238.6562341694589975 ) ) ;
#74224=CARTESIAN_POINT ( 'NONE',  ( -53.58581700929299529, 1385.100721272199962, 269.0214992842330162 ) ) ;
#74249=CARTESIAN_POINT ( 'NONE',  ( -107.0577634130000035, 1388.202339906730003, 298.5958247604589815 ) ) ;
#74251=CARTESIAN_POINT ( 'NONE',  ( -105.4593524120000012, 1391.263056100180165, 303.4133042968589962 ) ) ;
#74256=CARTESIAN_POINT ( 'NONE',  ( 1.756561144747210293E-16, 1391.913060387289988, 209.1218459572589836 ) ) ;
#74272=CARTESIAN_POINT ( 'NONE',  ( -98.72417372059999252, 1381.942632977169751, 297.0446025502590146 ) ) ;
#74299=CARTESIAN_POINT ( 'NONE',  ( -5.013264356158945390, 1375.417427871223254, 214.7179447576116900 ) ) ;
#74340=EDGE_CURVE ( 'NONE', #99409, #15055, #94862, .T. ) ;
#74342=CARTESIAN_POINT ( 'NONE',  ( -68.78852321903210054, 1379.747967857259937, 280.2968415580110673 ) ) ;
#74381=CARTESIAN_POINT ( 'NONE',  ( -109.1689158750000104, 1385.013785682389880, 297.1335957845589633 ) ) ;
#74393=CARTESIAN_POINT ( 'NONE',  ( -49.07962222725669932, 1383.813429589529960, 259.4477374396440155 ) ) ;
#74400=VERTEX_POINT ( 'NONE', #64928 ) ;
#74402=CARTESIAN_POINT ( 'NONE',  ( -37.20406409030000106, 1384.574232116320218, 210.1855829817990013 ) ) ;
#74413=CARTESIAN_POINT ( 'NONE',  ( -105.5912118399999997, 1378.611694080989992, 302.9832659653590099 ) ) ;
#74431=CARTESIAN_POINT ( 'NONE',  ( -109.1023536789999895, 1387.345544197499976, 310.8967553272590294 ) ) ;
#74456=CARTESIAN_POINT ( 'NONE',  ( -107.2926799547009864, 1378.913060387329779, 300.7951754864200211 ) ) ;
#74457=DIRECTION ( 'NONE',  ( -3.247745162871014848E-19, -1.000000000000000000, -7.717164782866489769E-18 ) ) ;
#74462=CARTESIAN_POINT ( 'NONE',  ( -39.76527504970000138, 1384.717239764220039, 212.4523225820389882 ) ) ;
#74493=CARTESIAN_POINT ( 'NONE',  ( -12.55357009390000123, 1380.105834429130255, 214.3611497310990046 ) ) ;
#74498=CARTESIAN_POINT ( 'NONE',  ( -102.5889311002350155, 1384.940216307899846, 311.0676245730850269 ) ) ;
#74499=CARTESIAN_POINT ( 'NONE',  ( -8.753431510080000422, 1385.526834493349952, 199.9255429183990032 ) ) ;
#74534=CARTESIAN_POINT ( 'NONE',  ( -104.0123117872064142, 1380.205049092886156, 306.5154211266013817 ) ) ;
#74539=CARTESIAN_POINT ( 'NONE',  ( -12.30840189449999933, 1378.376159634960231, 209.8321859945540098 ) ) ;
#74541=CARTESIAN_POINT ( 'NONE',  ( -65.89688115222600118, 1385.091299999440025, 257.0426204345699830 ) ) ;
#74552=CARTESIAN_POINT ( 'NONE',  ( -109.4716062389999962, 1384.569436532440022, 311.2688442282590131 ) ) ;
#74567=CARTESIAN_POINT ( 'NONE',  ( -68.58923311738080031, 1379.747637154969880, 280.1848937903309888 ) ) ;
#74570=CARTESIAN_POINT ( 'NONE',  ( -8.055471353928528089, 1382.512276592904755, 218.5978840298738817 ) ) ;
#74579=CARTESIAN_POINT ( 'NONE',  ( -106.6474845526250022, 1378.913060387289988, 306.6623049594010126 ) ) ;
#74590=ORIENTED_EDGE ( 'NONE', *, *, #27539, .F. ) ;
#74597=AXIS2_PLACEMENT_3D ( 'NONE', #16105, #59260, #7723 ) ;
#74598=CARTESIAN_POINT ( 'NONE',  ( -13.16532433220000087, 1379.531301371890095, 208.2880016088489867 ) ) ;
#74603=CARTESIAN_POINT ( 'NONE',  ( -73.83428086117611144, 1384.760717133270191, 273.3968393063270241 ) ) ;
#74604=ORIENTED_EDGE ( 'NONE', *, *, #103310, .F. ) ;
#74646=TOROIDAL_SURFACE ( 'NONE', #1266, 8.013264357029999729, 0.5000000000000000000 ) ;
#74656=CARTESIAN_POINT ( 'NONE',  ( -9.012915958852776299, 1388.961832031413678, 217.6296823903735174 ) ) ;
#74658=EDGE_CURVE ( 'NONE', #101907, #40922, #77043, .T. ) ;
#74675=CARTESIAN_POINT ( 'NONE',  ( -55.66145447376079858, 1384.713837345919956, 273.0923277504820135 ) ) ;
#74676=CARTESIAN_POINT ( 'NONE',  ( -107.1942030874700009, 1391.913060387289988, 301.3138641182989659 ) ) ;
#74679=CARTESIAN_POINT ( 'NONE',  ( -106.8337455069999891, 1378.992203654629748, 300.5412270638589689 ) ) ;
#74692=CARTESIAN_POINT ( 'NONE',  ( -14.05435969296220122, 1379.579181450040096, 211.8388747788069963 ) ) ;
#74702=CARTESIAN_POINT ( 'NONE',  ( -3.771520282370200317, 1380.389636976869951, 210.0680625258100065 ) ) ;
#74704=CARTESIAN_POINT ( 'NONE',  ( -54.22704658621609752, 1379.707482379519888, 254.1827617957189602 ) ) ;
#74729=AXIS2_PLACEMENT_3D ( 'NONE', #74256, #110586, #33872 ) ;
#74730=CARTESIAN_POINT ( 'NONE',  ( -109.4932991490571084, 1386.884154433499134, 311.1438796777470088 ) ) ;
#74732=CARTESIAN_POINT ( 'NONE',  ( -12.34520063366950104, 1378.885613852760116, 209.2790730372699954 ) ) ;
#74735=CARTESIAN_POINT ( 'NONE',  ( -37.47102956639999860, 1379.243633315240004, 218.9879198348490092 ) ) ;
#74747=CARTESIAN_POINT ( 'NONE',  ( -27.66920512940000165, 1384.171455447559993, 225.5844863493589969 ) ) ;
#74750=EDGE_CURVE ( 'NONE', #6492, #55409, #70754, .T. ) ;
#74762=CARTESIAN_POINT ( 'NONE',  ( -61.90500753679999946, 1389.465434365910141, 278.4656905976589769 ) ) ;
#74764=CARTESIAN_POINT ( 'NONE',  ( -46.41362929351480204, 1385.143899196999882, 254.3628368276549736 ) ) ;
#74773=CARTESIAN_POINT ( 'NONE',  ( -8.022894047070002088, 1384.893632254190152, 218.7875299896990100 ) ) ;
#74791=CARTESIAN_POINT ( 'NONE',  ( -105.7729677439999989, 1391.435361027740100, 301.9753519533589952 ) ) ;
#74842=CARTESIAN_POINT ( 'NONE',  ( -110.0634396883849888, 1384.924418016600157, 296.9511783967739689 ) ) ;
#74847=CARTESIAN_POINT ( 'NONE',  ( -8.602127442139998692, 1384.796933599069916, 199.8703343037190052 ) ) ;
#74848=CARTESIAN_POINT ( 'NONE',  ( -113.4589914632272354, 1379.913060387289988, 306.7211498618012229 ) ) ;
#74869=CARTESIAN_POINT ( 'NONE',  ( -40.61359552661080130, 1384.584710295609966, 213.5025725185709859 ) ) ;
#74884=CARTESIAN_POINT ( 'NONE',  ( -68.78640996459999712, 1379.747964976010053, 280.2617497814590024 ) ) ;
#74890=CARTESIAN_POINT ( 'NONE',  ( -7.965999071544743515, 1384.920974961468573, 199.4892359573080682 ) ) ;
#74892=CARTESIAN_POINT ( 'NONE',  ( -13.36052273939999857, 1384.881792980340151, 218.9673617354289945 ) ) ;
#74910=ORIENTED_EDGE ( 'NONE', *, *, #88529, .T. ) ;
#74939=EDGE_CURVE ( 'NONE', #7907, #83109, #48287, .T. ) ;
#74942=CARTESIAN_POINT ( 'NONE',  ( -36.89664068000400476, 1383.832789048189852, 236.6899286370959885 ) ) ;
#74948=ORIENTED_EDGE ( 'NONE', *, *, #102175, .F. ) ;
#74950=CARTESIAN_POINT ( 'NONE',  ( -57.78400604769999660, 1379.993142806879860, 268.6303832713589372 ) ) ;
#74954=CARTESIAN_POINT ( 'NONE',  ( -7.832093571712239743, 1386.408921254229881, 218.8164462652940188 ) ) ;
#74960=CARTESIAN_POINT ( 'NONE',  ( -106.4588356590000018, 1379.450307938419883, 300.3490905575590091 ) ) ;
#74980=CARTESIAN_POINT ( 'NONE',  ( -109.3083912430000026, 1384.947610311819972, 311.2693625272590339 ) ) ;
#75008=CARTESIAN_POINT ( 'NONE',  ( -85.85832257059999506, 1385.179345198489955, 289.6849318678590066 ) ) ;
#75011=CIRCLE ( 'NONE', #59035, 12.34219900309999929 ) ;
#75039=CARTESIAN_POINT ( 'NONE',  ( -10.86174217150000132, 1379.353463880399886, 215.1474020563989882 ) ) ;
#75046=CARTESIAN_POINT ( 'NONE',  ( -9.189822540219999780, 1387.666581765899991, 200.6527716693889829 ) ) ;
#75053=CARTESIAN_POINT ( 'NONE',  ( -9.107652377995819393, 1383.903739771440087, 218.5399116860239985 ) ) ;
#75057=B_SPLINE_SURFACE_WITH_KNOTS ( 'NONE', 5, 5, ( 
 ( #107579, #108121, #13495, #71830, #107029, #31415 ),
 ( #12416, #56086, #57207, #46600, #89671, #30865 ),
 ( #4579, #65040, #63417, #65598, #63957, #99710 ),
 ( #14054, #80735, #105949, #4044, #99157, #98071 ),
 ( #98621, #22436, #21341, #81264, #21884, #38714 ),
 ( #90212, #48243, #58292, #48, #15151, #66705 ) ),
 .UNSPECIFIED., .F., .F., .F.,
 ( 6, 6 ),
 ( 6, 6 ),
 ( 0.9035843706480000126, 1.040557828610000124 ),
 ( 0.000000000000000000, 2.000000000000000000 ),
 .UNSPECIFIED. ) ;
#75060=CARTESIAN_POINT ( 'NONE',  ( -108.4006655237829619, 1388.767505148533473, 298.1061185306318180 ) ) ;
#75085=CARTESIAN_POINT ( 'NONE',  ( -106.3938867745919765, 1381.879201070689533, 309.8074937847794104 ) ) ;
#75091=CARTESIAN_POINT ( 'NONE',  ( -12.31045119110000030, 1378.376187955050000, 209.7947064970570068 ) ) ;
#75093=CARTESIAN_POINT ( 'NONE',  ( -52.85310310605240147, 1385.029698763549959, 229.9496117000900028 ) ) ;
#75106=CARTESIAN_POINT ( 'NONE',  ( -109.1338056169999930, 1384.841083573769993, 311.2641749022590147 ) ) ;
#75122=CARTESIAN_POINT ( 'NONE',  ( -68.63354038389999801, 1379.747798109390033, 280.2252688738590223 ) ) ;
#75134=CARTESIAN_POINT ( 'NONE',  ( -106.8251098314479890, 1378.913060387289988, 306.9346524642279519 ) ) ;
#75156=CARTESIAN_POINT ( 'NONE',  ( -11.92422106699999951, 1391.277242477369782, 212.8274739234090021 ) ) ;
#75157=CARTESIAN_POINT ( 'NONE',  ( -84.36447712522229381, 1384.814979508860006, 288.1273280664730123 ) ) ;
#75181=CARTESIAN_POINT ( 'NONE',  ( -113.4000000000000057, 1391.913060387289988, 304.2218459572590064 ) ) ;
#75188=CARTESIAN_POINT ( 'NONE',  ( -8.848479971949998912, 1384.899922694570023, 199.9247835823190087 ) ) ;
#75203=DIRECTION ( 'NONE',  ( 0.000000000000000000, 0.000000000000000000, -1.000000000000000000 ) ) ;
#75207=CARTESIAN_POINT ( 'NONE',  ( -12.26364123840000175, 1375.886883438980021, 209.1218459572589836 ) ) ;
#75225=CARTESIAN_POINT ( 'NONE',  ( -43.38367995432890467, 1384.771901656779846, 248.3716437928619882 ) ) ;
#75229=CARTESIAN_POINT ( 'NONE',  ( -107.7365696490000033, 1379.032352522900055, 299.3254846616590044 ) ) ;
#75234=CARTESIAN_POINT ( 'NONE',  ( -10.42233989824366702, 1379.729316471301445, 202.4697405137477801 ) ) ;
#75244=CARTESIAN_POINT ( 'NONE',  ( -13.47873387835659997, 1379.610484773819962, 211.5873092184639859 ) ) ;
#75255=CARTESIAN_POINT ( 'NONE',  ( -24.56185491079999750, 1376.959776039820099, 215.3443103757190329 ) ) ;
#75257=CARTESIAN_POINT ( 'NONE',  ( -29.83023120264250139, 1379.643204280620012, 217.9872659232200078 ) ) ;
#75263=ORIENTED_EDGE ( 'NONE', *, *, #51030, .T. ) ;
#75270=AXIS2_PLACEMENT_3D ( 'NONE', #79061, #104791, #2366 ) ;
#75285=CARTESIAN_POINT ( 'NONE',  ( -107.9413468032178116, 1389.158540163861062, 309.9172676812428904 ) ) ;
#75291=CARTESIAN_POINT ( 'NONE',  ( -7.592224575760000427, 1375.673697770030230, 207.5503173039290061 ) ) ;
#75306=CARTESIAN_POINT ( 'NONE',  ( -76.11462884880000956, 1384.355091197029878, 301.2025005888589817 ) ) ;
#75320=CARTESIAN_POINT ( 'NONE',  ( -54.13887208369999371, 1385.096747890979941, 270.3642349231589606 ) ) ;
#75322=CARTESIAN_POINT ( 'NONE',  ( -48.32414939222230288, 1385.132224470989740, 258.2732643174430223 ) ) ;
#75330=CIRCLE ( 'NONE', #102148, 7.999657266239995401 ) ;
#75333=CARTESIAN_POINT ( 'NONE',  ( -113.4000000000000057, 1384.899971913130003, 304.2218459572590064 ) ) ;
#75369=ORIENTED_EDGE ( 'NONE', *, *, #50873, .F. ) ;
#75381=CARTESIAN_POINT ( 'NONE',  ( -50.14839348009999753, 1380.010081756269983, 242.5009839091590038 ) ) ;
#75392=EDGE_LOOP ( 'NONE', ( #44616, #41220, #32461, #55267, #10646 ) ) ;
#75420=ORIENTED_EDGE ( 'NONE', *, *, #101505, .T. ) ;
#75421=CARTESIAN_POINT ( 'NONE',  ( -101.9210842609999901, 1379.177752269670009, 302.4435101425590346 ) ) ;
#75428=CARTESIAN_POINT ( 'NONE',  ( -47.39586428316670208, 1384.608660850170054, 221.4693795585880025 ) ) ;
#75440=CONICAL_SURFACE ( 'NONE', #21753, 12.50000000000000000, 0.02617993877989872875 ) ;
#75441=CARTESIAN_POINT ( 'NONE',  ( -68.74147317429999759, 1379.748081684489989, 280.1371050876589948 ) ) ;
#75470=EDGE_CURVE ( 'NONE', #7502, #41641, #15939, .T. ) ;
#75485=EDGE_LOOP ( 'NONE', ( #65395, #58348, #58268, #18768 ) ) ;
#75495=CARTESIAN_POINT ( 'NONE',  ( -69.24343105989969160, 1383.785972937140059, 293.9299002094780349 ) ) ;
#75503=CARTESIAN_POINT ( 'NONE',  ( -54.29265189920000267, 1383.804803630430115, 270.2912082677589751 ) ) ;
#75507=CARTESIAN_POINT ( 'NONE',  ( -8.888812255142289231, 1385.314781883149863, 218.6605257023059892 ) ) ;
#75512=CARTESIAN_POINT ( 'NONE',  ( -106.6838299039999924, 1381.594688875880138, 298.7333698723590487 ) ) ;
#75527=CARTESIAN_POINT ( 'NONE',  ( -8.861903497826141063, 1384.885539543426603, 218.6850719556965998 ) ) ;
#75532=CARTESIAN_POINT ( 'NONE',  ( -108.3701702990000086, 1386.736519522250092, 310.7981234312589436 ) ) ;
#75561=CARTESIAN_POINT ( 'NONE',  ( -53.45887188369999876, 1384.635297440300064, 230.7554238970589893 ) ) ;
#75573=CARTESIAN_POINT ( 'NONE',  ( -11.12430337309289818, 1391.913060387059886, 206.3375259381840294 ) ) ;
#75595=CARTESIAN_POINT ( 'NONE',  ( -10.42949413029999839, 1379.124834216069985, 215.7630140696190040 ) ) ;
#75602=CARTESIAN_POINT ( 'NONE',  ( -14.28029416299999887, 1390.367276380369958, 209.8449221693030040 ) ) ;
#75607=CARTESIAN_POINT ( 'NONE',  ( -8.981694392507570512, 1384.175213772349935, 218.6078250012760122 ) ) ;
#75632=CARTESIAN_POINT ( 'NONE',  ( -109.7183341539999901, 1384.893508909079856, 297.0862237871589855 ) ) ;
#75636=CARTESIAN_POINT ( 'NONE',  ( -103.6849498593194454, 1379.968036174091139, 305.2864844434715224 ) ) ;
#75640=DIRECTION ( 'NONE',  ( 0.000000000000000000, 0.000000000000000000, -1.000000000000000000 ) ) ;
#75641=CARTESIAN_POINT ( 'NONE',  ( -14.09844076420000114, 1379.806461617270088, 211.4199521846090022 ) ) ;
#75643=CARTESIAN_POINT ( 'NONE',  ( -59.16917651648999055, 1385.057337441720165, 242.2145958383559901 ) ) ;
#75644=CARTESIAN_POINT ( 'NONE',  ( -11.31284123697730060, 1391.913060387289988, 211.6673135973910291 ) ) ;
#75653=CARTESIAN_POINT ( 'NONE',  ( -109.1319690089999881, 1384.726207818360081, 311.2603020862590029 ) ) ;
#75667=CARTESIAN_POINT ( 'NONE',  ( -68.62877234682019889, 1379.747624006590058, 280.2303598637119535 ) ) ;
#75669=CARTESIAN_POINT ( 'NONE',  ( -7.827642019093867809, 1383.090619493809072, 218.8065417710187432 ) ) ;
#75700=CARTESIAN_POINT ( 'NONE',  ( -71.50733119889839884, 1384.746684647190023, 268.9689952328979530 ) ) ;
#75717=CARTESIAN_POINT ( 'NONE',  ( -60.07536325030000057, 1379.722864260740153, 261.7802271240589675 ) ) ;
#75733=CARTESIAN_POINT ( 'NONE',  ( -7.966197656679999461, 1384.914723845990011, 199.4893138218189961 ) ) ;
#75750=CARTESIAN_POINT ( 'NONE',  ( -10.06053593028460647, 1390.279853981375481, 216.3031875838134681 ) ) ;
#75766=CARTESIAN_POINT ( 'NONE',  ( -48.61829462142750202, 1384.746706768770082, 258.8939480861469633 ) ) ;
#75767=CARTESIAN_POINT ( 'NONE',  ( -106.5910199462759920, 1391.913060387289988, 302.7980903714330339 ) ) ;
#75769=CARTESIAN_POINT ( 'NONE',  ( -106.4840262270000011, 1379.607751643809934, 300.2526974370589983 ) ) ;
#75773=CARTESIAN_POINT ( 'NONE',  ( -12.10295352893632703, 1377.835289027229692, 206.7956396381484012 ) ) ;
#75793=CARTESIAN_POINT ( 'NONE',  ( -39.44686632430000373, 1376.826872897580188, 228.9534929901590203 ) ) ;
#75796=CARTESIAN_POINT ( 'NONE',  ( -43.20831771794370013, 1379.668237090550065, 233.4372218537739911 ) ) ;
#75802=CARTESIAN_POINT ( 'NONE',  ( -105.7049770469999999, 1379.426018556420104, 306.8995712054589831 ) ) ;
#75803=DIRECTION ( 'NONE',  ( -3.237679667471999896E-17, -1.000000000000000000, -6.999474336859099157E-17 ) ) ;
#75831=CARTESIAN_POINT ( 'NONE',  ( -28.76039927569999932, 1375.228231664269970, 215.0392276715589901 ) ) ;
#75836=CARTESIAN_POINT ( 'NONE',  ( -105.3710641919550000, 1378.843319234500086, 304.5215261602800183 ) ) ;
#75845=CARTESIAN_POINT ( 'NONE',  ( -109.9987472809999929, 1384.304072719160104, 311.2333125242590199 ) ) ;
#75855=CARTESIAN_POINT ( 'NONE',  ( -60.19932042489999446, 1388.230348997210058, 279.3978214739589703 ) ) ;
#75857=CARTESIAN_POINT ( 'NONE',  ( -51.53876818608200239, 1385.112767378740045, 264.8854167730279414 ) ) ;
#75866=CARTESIAN_POINT ( 'NONE',  ( -8.580993339069999948, 1384.885542790459795, 218.6696210660190047 ) ) ;
#75868=CARTESIAN_POINT ( 'NONE',  ( -106.6282499509799919, 1381.613467129139963, 309.5665933865749935 ) ) ;
#75869=ORIENTED_EDGE ( 'NONE', *, *, #74939, .F. ) ;
#75872=AXIS2_PLACEMENT_3D ( 'NONE', #5505, #67090, #6055 ) ;
#75883=CARTESIAN_POINT ( 'NONE',  ( -109.0477392060000028, 1386.067204197109959, 297.2757566815589598 ) ) ;
#75912=CARTESIAN_POINT ( 'NONE',  ( -12.30069474339200042, 1378.346207744910089, 209.9425806866760240 ) ) ;
#75926=CARTESIAN_POINT ( 'NONE',  ( -110.0628941928870006, 1384.909579410989863, 296.9513031325649877 ) ) ;
#75929=CARTESIAN_POINT ( 'NONE',  ( -7.964281638630000160, 1384.840201205250196, 199.4899964382389896 ) ) ;
#75936=ORIENTED_EDGE ( 'NONE', *, *, #11837, .F. ) ;
#75944=AXIS2_PLACEMENT_3D ( 'NONE', #62966, #45591, #89217 ) ;
#75947=AXIS2_PLACEMENT_3D ( 'NONE', #38960, #73138, #107280 ) ;
#75956=CARTESIAN_POINT ( 'NONE',  ( -44.14995057972470249, 1384.596438297579880, 217.3237505064830088 ) ) ;
#75963=CARTESIAN_POINT ( 'NONE',  ( -16.16124070225407294, 1379.595261704359018, 212.2433978542155444 ) ) ;
#75968=CARTESIAN_POINT ( 'NONE',  ( -68.31895350100000996, 1379.747064260159959, 279.0929441650590093 ) ) ;
#75976=CARTESIAN_POINT ( 'NONE',  ( -1.381610875089999979E-15, 1384.913060387289988, 218.6218459572590120 ) ) ;
#76000=CARTESIAN_POINT ( 'NONE',  ( -4.145978979534980458E-15, 1375.413060387289988, 209.1218459572589836 ) ) ;
#76020=CARTESIAN_POINT ( 'NONE',  ( -71.04079330152269733, 1383.784253855209954, 295.9543559495810428 ) ) ;
#76027=ADVANCED_FACE ( 'NONE', ( #40374 ), #23153, .F. ) ;
#76032=CARTESIAN_POINT ( 'NONE',  ( -33.74298654390000252, 1380.921279986640229, 228.6690588220590143 ) ) ;
#76045=CARTESIAN_POINT ( 'NONE',  ( -104.2862556689999991, 1379.876065007149919, 302.9147207968590578 ) ) ;
#76068=CARTESIAN_POINT ( 'NONE',  ( -107.7932546339999931, 1388.509443340949929, 309.9252778232590231 ) ) ;
#76078=CARTESIAN_POINT ( 'NONE',  ( -14.33548952289999967, 1390.363893295419984, 208.3507362592630159 ) ) ;
#76090=CARTESIAN_POINT ( 'NONE',  ( -12.61160394886860026, 1379.083170910369972, 208.5076010362149930 ) ) ;
#76101=CARTESIAN_POINT ( 'NONE',  ( -109.9849286017959997, 1384.913355884089924, 311.4561078401599730 ) ) ;
#76118=CARTESIAN_POINT ( 'NONE',  ( -3.078458326440000281, 1391.041439170870035, 208.7217714433539868 ) ) ;
#76126=CARTESIAN_POINT ( 'NONE',  ( -13.14956782490000009, 1379.692368811980032, 212.8542620991189835 ) ) ;
#76133=CARTESIAN_POINT ( 'NONE',  ( -13.37265018080000090, 1390.548598904210166, 209.7987839237050309 ) ) ;
#76151=CARTESIAN_POINT ( 'NONE',  ( -15.41379235132240133, 1383.858177494749953, 219.3473563989259958 ) ) ;
#76165=CARTESIAN_POINT ( 'NONE',  ( -110.0629075430000086, 1384.909055395449968, 296.9513015316589986 ) ) ;
#76167=CARTESIAN_POINT ( 'NONE',  ( -5.607667144112319590, 1391.799625134960024, 203.2661880012859967 ) ) ;
#76176=CARTESIAN_POINT ( 'NONE',  ( -11.03495751070000175, 1391.553749705140035, 203.9031261639289880 ) ) ;
#76177=CARTESIAN_POINT ( 'NONE',  ( -84.62390092619399695, 1385.174868275669951, 288.3880241305470236 ) ) ;
#76178=CARTESIAN_POINT ( 'NONE',  ( -10.51241594247230005, 1391.913060387289988, 213.5546871049940023 ) ) ;
#76182=EDGE_CURVE ( 'NONE', #51642, #27006, #9822, .T. ) ;
#76192=CARTESIAN_POINT ( 'NONE',  ( -14.08142637225379978, 1379.709117121690042, 211.5303641152310092 ) ) ;
#76206=CARTESIAN_POINT ( 'NONE',  ( -68.70087839430000543, 1379.747840857399979, 280.2882393206589882 ) ) ;
#76209=CARTESIAN_POINT ( 'NONE',  ( -8.013767138614300123, 1382.608589018177554, 218.6364342332414026 ) ) ;
#76220=( NAMED_UNIT ( * ) PLANE_ANGLE_UNIT ( ) SI_UNIT ( $, .RADIAN. ) );
#76221=CARTESIAN_POINT ( 'NONE',  ( -13.38006552295539997, 1379.538105693709895, 208.4172449948689803 ) ) ;
#76233=CARTESIAN_POINT ( 'NONE',  ( -14.15085831685690110, 1380.030482968580145, 211.0724251982179851 ) ) ;
#76239=CARTESIAN_POINT ( 'NONE',  ( -1.742717375088950107E-15, 1375.426148861440197, 209.1218459572589836 ) ) ;
#76240=CARTESIAN_POINT ( 'NONE',  ( -10.07717734240000063, 1391.913060387289988, 214.9705334440889715 ) ) ;
#76241=CARTESIAN_POINT ( 'NONE',  ( -87.22158348405449146, 1384.827375891360134, 290.6397261970639647 ) ) ;
#76257=CARTESIAN_POINT ( 'NONE',  ( -54.44115314580000131, 1379.700200843730045, 248.9289766756589870 ) ) ;
#76293=CARTESIAN_POINT ( 'NONE',  ( -9.255471102502529135, 1389.295763922535798, 217.3525502945869903 ) ) ;
#76312=CARTESIAN_POINT ( 'NONE',  ( -44.65204099977980690, 1384.765860786410030, 250.8497032329840124 ) ) ;
#76321=CARTESIAN_POINT ( 'NONE',  ( -8.586603470991246212, 1382.365454073439651, 200.1294793584183935 ) ) ;
#76344=CARTESIAN_POINT ( 'NONE',  ( -48.05471153476000268, 1379.681133392060019, 241.5169778073720011 ) ) ;
#76350=CARTESIAN_POINT ( 'NONE',  ( -107.0802177269999902, 1378.913060387289988, 307.3184745608590447 ) ) ;
#76351=CARTESIAN_POINT ( 'NONE',  ( -109.6575798300000031, 1384.922737831749828, 311.3230295302589639 ) ) ;
#76376=CARTESIAN_POINT ( 'NONE',  ( -26.65670438309999923, 1379.321141781539836, 211.2412313610489889 ) ) ;
#76380=DIRECTION ( 'NONE',  ( -1.836970198721029688E-16, -1.000000000000000000, 0.000000000000000000 ) ) ;
#76399=CARTESIAN_POINT ( 'NONE',  ( -46.12437349460000036, 1389.616683096550105, 246.0195738906589895 ) ) ;
#76401=CARTESIAN_POINT ( 'NONE',  ( -69.10652963092418588, 1385.027354731980040, 294.0433430371250552 ) ) ;
#76411=CARTESIAN_POINT ( 'NONE',  ( -108.9087294810559996, 1383.070058043159861, 310.9164552416630158 ) ) ;
#76412=B_SPLINE_CURVE_WITH_KNOTS ( 'NONE', 5,
 ( #11671, #1635, #104069, #18945, #87849, #71063, #105185, #10573, #20061, #88381, #45847, #536, #68844, #102948, #60437 ),
 .UNSPECIFIED., .F., .F.,
 ( 6, 3, 3, 3, 6 ),
 ( 0.000000000000000000, 0.3446931986191029695, 0.5658372174535590826, 0.8241082499738381362, 1.000000000000000000 ),
 .UNSPECIFIED. ) ;
#76451=EDGE_CURVE ( 'NONE', #16403, #105885, #86037, .T. ) ;
#76460=CARTESIAN_POINT ( 'NONE',  ( -14.31906343784990021, 1380.323795378649947, 209.9058136714729983 ) ) ;
#76476=CARTESIAN_POINT ( 'NONE',  ( -110.0628895161599985, 1384.915043845459877, 296.9512959549039692 ) ) ;
#76504=CARTESIAN_POINT ( 'NONE',  ( -29.89848049817870290, 1384.555929490659992, 205.5315682105770065 ) ) ;
#76515=CARTESIAN_POINT ( 'NONE',  ( -68.14024846860000650, 1379.746849200649876, 278.7967730264589932 ) ) ;
#76524=VERTEX_POINT ( 'NONE', #107872 ) ;
#76537=CARTESIAN_POINT ( 'NONE',  ( -8.859979363206980096, 1384.988067842360124, 218.6842175230869714 ) ) ;
#76544=CARTESIAN_POINT ( 'NONE',  ( -113.4000000000000057, 1381.413060387289988, 304.2218459572590064 ) ) ;
#76546=CARTESIAN_POINT ( 'NONE',  ( -7.544890056106759779, 1384.926148859619843, 219.0875905756669795 ) ) ;
#76555=CARTESIAN_POINT ( 'NONE',  ( 2.283436972078669822E-15, 1391.413060387289988, 209.1218459572589836 ) ) ;
#76570=CARTESIAN_POINT ( 'NONE',  ( -61.79250326028719797, 1383.794347301399966, 283.5912797454389533 ) ) ;
#76580=CARTESIAN_POINT ( 'NONE',  ( -52.43938806090000071, 1381.597557294350281, 231.3376853649589862 ) ) ;
#76586=CARTESIAN_POINT ( 'NONE',  ( -113.4000000000000057, 1381.413060387289988, 304.2218459572590064 ) ) ;
#76591=CARTESIAN_POINT ( 'NONE',  ( -108.0946408660000060, 1381.519821111719921, 298.2388064062590729 ) ) ;
#76614=CARTESIAN_POINT ( 'NONE',  ( -106.5011323819999944, 1389.176690760049951, 308.8516233391590049 ) ) ;
#76665=CARTESIAN_POINT ( 'NONE',  ( -9.787614191920001261, 1388.284344778709965, 200.9830834995690054 ) ) ;
#76673=CARTESIAN_POINT ( 'NONE',  ( -12.13826128220000022, 1378.628687927729970, 212.1996395817189978 ) ) ;
#76679=CARTESIAN_POINT ( 'NONE',  ( -11.74761972249999964, 1388.317445593919956, 202.1816773684589919 ) ) ;
#76685=CARTESIAN_POINT ( 'NONE',  ( -8.859238207665629972, 1384.780024425459942, 218.6827953414510262 ) ) ;
#76700=CARTESIAN_POINT ( 'NONE',  ( -16.27387329549090111, 1383.857350287579948, 219.5485982243399974 ) ) ;
#76714=CARTESIAN_POINT ( 'NONE',  ( -109.8951077769999927, 1384.900382187740206, 297.0284516700590416 ) ) ;
#76717=CARTESIAN_POINT ( 'NONE',  ( -5.519031869189769068, 1391.701565166340060, 203.3041584978760170 ) ) ;
#76720=CARTESIAN_POINT ( 'NONE',  ( -5.932239102140000497, 1391.913060387289988, 215.1144410137189880 ) ) ;
#76725=CARTESIAN_POINT ( 'NONE',  ( -11.68975942279999991, 1391.913060387289988, 209.2396716380060013 ) ) ;
#76726=CARTESIAN_POINT ( 'NONE',  ( -77.91803962745299827, 1385.149028708040078, 280.1724417302780239 ) ) ;
#76768=FILL_AREA_STYLE ('',( #8442 ) ) ;
#76791=CARTESIAN_POINT ( 'NONE',  ( -12.03143819960000016, 1391.727509755350184, 211.6223019673990109 ) ) ;
#76792=CARTESIAN_POINT ( 'NONE',  ( -91.93393826891069409, 1384.846171626159958, 293.6354712203719828 ) ) ;
#76801=ORIENTED_EDGE ( 'NONE', *, *, #67205, .T. ) ;
#76811=CARTESIAN_POINT ( 'NONE',  ( -51.95708025780000128, 1379.690182529579943, 243.6310195730590067 ) ) ;
#76829=B_SPLINE_CURVE_WITH_KNOTS ( 'NONE', 3,
 ( #10988, #85457, #35075, #17687, #19361, #68703, #52453, #102808, #27234, #44041, #77637, #26103, #110675, #8755, #77096, #69818, #60293, #26664, #406, #44598, #78181, #70374, #103362, #34523, #94411, #9332, #60865, #51893, #86030, #35622, #94990, #53005, #18257, #87138, #9874, #10429, #104489, #45162, #106149, #106686, #37846, #80947, #64169, #29977, #105049, #72034, #11543, #96654, #55216, #89344, #12640, #22103, #21564, #13159, #46275, #47346, #36738, #64726, #80402, #3716, #12081, #4247, #19922, #81474, #4777, #98287, #79302, #29427, #54122, #46818, #73104, #55774, #54672, #45718, #38381, #97742, #72556, #89889, #63626, #21013, #38924, #63090, #70933, #107243, #71489, #30535, #2613, #98842, #56302, #90433, #28338, #62531, #88250, #79855, #3166, #37298, #105610, #28895, #97188, #20462, #88799, #65268, #23777, #57964, #92097, #101579, #101032, #92643, #14829, #15917, #5337, #33284, #49016, #83153, #91552, #99378, #22653, #48467, #39497, #73669, #99933, #6447, #56857, #15376, #41698, #109464, #23227, #14276, #6989, #66378, #49565, #83694, #40593, #74764, #32743, #107800, #50116, #41143, #75322, #31085, #100496, #66923, #24330, #108903, #32193, #108353, #58513, #84245, #90988, #7543, #75857, #82605, #5895, #57427, #110007, #67474, #24867, #65815, #40041, #74224, #59070, #13711, #47897, #82033, #31634, #54403, #3440, #2895, #19657, #276, #70661, #84787, #33841, #25974, #60173, #87998, #102141, #85903, #50656, #105890, #8085, #88535, #93727, #37572, #8631, #96937, #9210, #42254, #43370, #17005, #93193, #45990, #51769, #102678, #11284, #85334, #77518, #68031, #62823, #62252, #71208, #2350, #59614, #42806, #94291, #36464, #104777, #76401, #17569, #28063, #25419, #20204, #105328, #11819, #96378, #51205, #76966, #53860, #45449, #34402, #110555, #68575, #79590, #37014, #28621, #80121, #71772, #29169, #16462, #90716, #72295, #21833, #47086, #99105, #82326, #48187, #12355, #56031, #29713, #3992, #73384, #30811, #40315, #39776, #31361, #64448, #65545, #54941, #82868, #98564, #90157, #30255, #38116, #106427, #98011, #89069, #46545, #38661, #80679, #63897, #57148, #91275, #5624, #72837, #21282, #56582, #5061, #22382, #14001, #13438, #47628, #73935, #55491, #99654, #108066, #107520, #89616, #39207, #12907, #14555, #81756, #64988, #81211, #22944, #48744, #4526, #6161, #74498, #106970, #108627, #63359, #97475, #20745, #50940, #83970, #6713, #66653, #59354, #23510, #8911, #91817 ),
 .UNSPECIFIED., .F., .F.,
 ( 4, 3, 3, 3, 3, 3, 3, 3, 3, 3, 3, 3, 3, 3, 3, 3, 3, 3, 3, 3, 3, 3, 3, 3, 3, 3, 3, 3, 3, 3, 3, 3, 3, 3, 3, 3, 3, 3, 3, 3, 3, 3, 3, 3, 3, 3, 3, 3, 3, 3, 3, 3, 3, 3, 3, 3, 3, 3, 3, 3, 3, 3, 3, 3, 3, 3, 3, 3, 3, 3, 3, 3, 3, 3, 3, 3, 3, 3, 3, 3, 3, 3, 3, 3, 3, 3, 3, 3, 3, 3, 3, 3, 3, 3, 3, 3, 3, 3, 3, 3, 4 ),
 ( 9.527080348409999289, 10.85173027196099937, 12.00624473378430146, 13.10086034166340063, 14.14961175496640067, 15.14877182358010010, 15.39383910896309970, 16.42944771861520081, 17.50948676729140274, 18.64816147367130128, 19.92972531175479745, 21.39309245868300025, 23.20366259091170136, 24.59245591388290109, 25.84110766704660023, 26.97705335283380279, 27.58084801734310076, 28.68944630574549848, 29.82656121067200061, 30.99685979729480323, 32.20647895571269714, 33.49104441228929829, 34.83666280905310231, 36.25746581317260109, 37.80012760393510263, 39.36589684718460092, 40.85204067702190400, 41.39509552342049403, 43.75295810538389674, 46.16562766740489110, 48.42936579919658868, 50.56808164685719476, 52.48310125732749043, 54.31967719734500122, 56.09294667343839080, 57.81364711399808698, 59.48968560173540254, 61.10873929825010009, 62.70029911509010390, 64.25293939849369451, 65.53909258048099673, 67.16844705198229803, 68.87663427951409290, 70.69318331658230647, 72.67675589585680029, 75.06336699077600372, 77.83965603350679885, 79.89839901332899785, 81.75326913944610396, 83.48794843525729448, 85.13855407467239900, 86.69737124088230473, 88.21590074822410088, 89.68095808219059961, 90.91108773633949625, 92.82794843041369859, 94.79388189049979019, 96.79267130114249085, 98.79623022816639377, 100.7738431079329899, 102.7044857337120050, 104.5710202628480090, 106.3668334849150057, 108.1169125231769925, 109.8255655786209957, 111.4968565625370047, 113.1177619320860117, 114.7136499496349984, 116.2730054179010040, 117.6367619667960014, 119.0754927998699912, 120.5565149085459922, 122.0751441691740098, 123.5870575414840005, 125.0706667163910026, 126.5142087427740165, 127.9148134135910198, 129.2561388162960441, 130.5667318641620227, 131.8367184849859939, 132.4493970707720223, 133.5475295398549918, 134.6463778432060394, 135.7455120869569782, 136.8793330144310403, 137.9772763609580011, 139.0740946830690064, 140.1694335882050098, 141.2629533371109858, 142.3532320226559875, 143.4413191182189848, 144.5259477239419823, 144.8160795067510094, 146.5546788388820119, 148.3790043525229976, 150.2749373096100101, 152.1509483487260184, 153.9553471829370039, 155.6832911718549894, 157.3186866423189940, 157.6516401924140212 ),
 .UNSPECIFIED. ) ;
#76851=CARTESIAN_POINT ( 'NONE',  ( -8.949046086683678070, 1388.869870210199451, 217.7000893693110868 ) ) ;
#76867=CARTESIAN_POINT ( 'NONE',  ( -10.94176001355937977, 1391.017588921819652, 214.8528320132766112 ) ) ;
#76869=CARTESIAN_POINT ( 'NONE',  ( -74.53996386105208671, 1384.650779838590097, 299.6395783774970027 ) ) ;
#76870=CARTESIAN_POINT ( 'NONE',  ( -20.28996348272639949, 1384.951249660460007, 201.7330533080949806 ) ) ;
#76874=CARTESIAN_POINT ( 'NONE',  ( -107.9702631740000101, 1378.913060387289988, 299.5275268469590060 ) ) ;
#76890=CARTESIAN_POINT ( 'NONE',  ( -10.36756237719999874, 1382.682511944280122, 200.8304498154890041 ) ) ;
#76905=CARTESIAN_POINT ( 'NONE',  ( -31.28542702328589797, 1379.632103487770109, 219.4205719633520175 ) ) ;
#76936=CARTESIAN_POINT ( 'NONE',  ( -37.25828949241959265, 1379.646493637162166, 220.1838309194394583 ) ) ;
#76941=CARTESIAN_POINT ( 'NONE',  ( -103.8863835612550020, 1379.884582398730117, 304.0035884679699620 ) ) ;
#76964=CARTESIAN_POINT ( 'NONE',  ( -66.16583944359999236, 1390.700906735469971, 276.1376312171590257 ) ) ;
#76966=CARTESIAN_POINT ( 'NONE',  ( -72.47380510957108868, 1385.015833470149801, 297.6916867413240197 ) ) ;
#76973=ADVANCED_FACE ( 'NONE', ( #20982 ), #46485, .T. ) ;
#76978=DIRECTION ( 'NONE',  ( 1.000000000000000000, 0.000000000000000000, 0.000000000000000000 ) ) ;
#77033=CARTESIAN_POINT ( 'NONE',  ( -101.5621914980000042, 1376.194720364869909, 306.3892953801590124 ) ) ;
#77036=ORIENTED_EDGE ( 'NONE', *, *, #84290, .F. ) ;
#77041=CARTESIAN_POINT ( 'NONE',  ( -110.0629084955440078, 1384.909053975289908, 296.9513011978259556 ) ) ;
#77043=CIRCLE ( 'NONE', #68108, 2.500000000000002220 ) ;
#77065=CARTESIAN_POINT ( 'NONE',  ( -109.5441724480000119, 1375.366238318880050, 302.0293835567589440 ) ) ;
#77073=CARTESIAN_POINT ( 'NONE',  ( -30.61151124082590158, 1384.557641573209821, 205.9241274443010070 ) ) ;
#77081=CARTESIAN_POINT ( 'NONE',  ( -57.29365481403381466, 1379.717584333650848, 260.4218402486304171 ) ) ;
#77086=CARTESIAN_POINT ( 'NONE',  ( -68.54084681569999304, 1379.747861287210071, 279.6492226308589579 ) ) ;
#77094=CARTESIAN_POINT ( 'NONE',  ( -49.59345295620000371, 1385.124330617979922, 260.9076469794590025 ) ) ;
#77096=CARTESIAN_POINT ( 'NONE',  ( -13.28712287618670018, 1385.300651250900046, 219.1026202486000045 ) ) ;
#77141=CARTESIAN_POINT ( 'NONE',  ( -74.26730215954620462, 1383.781415895790133, 299.1588454321730524 ) ) ;
#77149=CARTESIAN_POINT ( 'NONE',  ( -53.30655931660000135, 1379.972319575679876, 259.1995162978590201 ) ) ;
#77160=CARTESIAN_POINT ( 'NONE',  ( -109.5839456589999941, 1383.369684524640206, 297.2159463091589942 ) ) ;
#77183=CARTESIAN_POINT ( 'NONE',  ( -108.0994041090000053, 1388.972225179880070, 310.0915140952590150 ) ) ;
#77222=CARTESIAN_POINT ( 'NONE',  ( -11.65026559816559981, 1391.913060387150153, 208.7216013930580232 ) ) ;
#77234=CARTESIAN_POINT ( 'NONE',  ( -4.167839424791409599E-16, 1389.896721459789887, 214.6127231082590185 ) ) ;
#77244=CARTESIAN_POINT ( 'NONE',  ( -8.039279795659998840, 1382.384107263689884, 218.6139994057390084 ) ) ;
#77250=CARTESIAN_POINT ( 'NONE',  ( -13.44625623449999985, 1389.878228146560105, 205.4975164690590077 ) ) ;
#77278=VERTEX_POINT ( 'NONE', #109692 ) ;
#77286=CARTESIAN_POINT ( 'NONE',  ( -12.80774525297199951, 1390.891660332020138, 210.6890168614469871 ) ) ;
#77290=CARTESIAN_POINT ( 'NONE',  ( -107.9736457860882268, 1380.698907176378498, 309.9509774194930856 ) ) ;
#77293=CARTESIAN_POINT ( 'NONE',  ( -11.42119214989999954, 1391.324142034819943, 204.4961053831890183 ) ) ;
#77294=CARTESIAN_POINT ( 'NONE',  ( -67.67823920127010240, 1385.100504050170002, 260.9636858420549856 ) ) ;
#77351=CARTESIAN_POINT ( 'NONE',  ( -107.2131581586909874, 1384.895988242240037, 297.0540560109790249 ) ) ;
#77369=CARTESIAN_POINT ( 'NONE',  ( -37.80579224959999607, 1379.643095642800063, 220.6117142568589884 ) ) ;
#77389=CARTESIAN_POINT ( 'NONE',  ( -109.1111611177930030, 1384.583257041720117, 311.2497810013429671 ) ) ;
#77418=CARTESIAN_POINT ( 'NONE',  ( -81.43278738633540570, 1384.635623096480003, 304.7600304791900498 ) ) ;
#77420=CARTESIAN_POINT ( 'NONE',  ( -26.92027982241999950, 1384.963071672040087, 204.0559658860740058 ) ) ;
#77440=CARTESIAN_POINT ( 'NONE',  ( -9.263518881979999620, 1384.040644720069849, 200.0636813112390087 ) ) ;
#77454=CARTESIAN_POINT ( 'NONE',  ( -62.63656304554481125, 1379.732098069620179, 270.6469071953959542 ) ) ;
#77460=CARTESIAN_POINT ( 'NONE',  ( -106.5585968837300044, 1390.939245634569943, 300.3884029622149683 ) ) ;
#77470=FILL_AREA_STYLE_COLOUR ( '', #109354 ) ;
#77476=ORIENTED_EDGE ( 'NONE', *, *, #81471, .F. ) ;
#77478=CARTESIAN_POINT ( 'NONE',  ( -5.013264327984152224, 1375.413060387289988, 203.5257471471711312 ) ) ;
#77489=CARTESIAN_POINT ( 'NONE',  ( -49.28295861101878472, 1379.685963475619246, 238.1969093270015776 ) ) ;
#77494=CARTESIAN_POINT ( 'NONE',  ( -105.3812835198930031, 1378.843491006310160, 304.0398711368210343 ) ) ;
#77516=CARTESIAN_POINT ( 'NONE',  ( -81.20151922889999696, 1386.553224299360181, 304.9219196665589493 ) ) ;
#77518=CARTESIAN_POINT ( 'NONE',  ( -65.34101701133390350, 1385.041919093109982, 289.2241435049139682 ) ) ;
#77528=CARTESIAN_POINT ( 'NONE',  ( -108.2558473347470027, 1382.950532872079975, 310.7470917612149606 ) ) ;
#77542=CARTESIAN_POINT ( 'NONE',  ( -109.7887639940000071, 1385.331325759269930, 297.0716752156589564 ) ) ;
#77558=CARTESIAN_POINT ( 'NONE',  ( -15.65684374876079943, 1384.875147521260033, 219.5768865249289945 ) ) ;
#77610=CARTESIAN_POINT ( 'NONE',  ( -105.7801839960000052, 1376.961008902830145, 301.4143074619590266 ) ) ;
#77611=CARTESIAN_POINT ( 'NONE',  ( -106.1624399561229950, 1378.913060387289988, 302.5126857932060034 ) ) ;
#77615=CARTESIAN_POINT ( 'NONE',  ( -73.11479823269999656, 1385.127942832860072, 272.3424178700590232 ) ) ;
#77616=CARTESIAN_POINT ( 'NONE',  ( -65.13305399213498958, 1384.705767306430062, 255.3553050933879831 ) ) ;
#77627=CARTESIAN_POINT ( 'NONE',  ( -68.35177030640001306, 1379.747234628189972, 279.2299283338589930 ) ) ;
#77635=CARTESIAN_POINT ( 'NONE',  ( -13.36456641330000039, 1385.300820372649923, 218.9430041755990146 ) ) ;
#77637=CARTESIAN_POINT ( 'NONE',  ( -12.19044366360270004, 1385.304304086989987, 218.9500151190139832 ) ) ;
#77681=CARTESIAN_POINT ( 'NONE',  ( -69.58852568934280214, 1383.785633056889992, 294.3347849598490029 ) ) ;
#77688=CARTESIAN_POINT ( 'NONE',  ( -82.19905968850000022, 1381.016078469080185, 303.3370635716590300 ) ) ;
#77702=CARTESIAN_POINT ( 'NONE',  ( -107.8378136989999945, 1382.531835676999890, 297.9003899234589881 ) ) ;
#77720=CARTESIAN_POINT ( 'NONE',  ( -110.0629901356764435, 1384.906028625631279, 296.9512903121827208 ) ) ;
#77724=CARTESIAN_POINT ( 'NONE',  ( -103.9064370230000094, 1389.684541055990167, 306.7300248541590122 ) ) ;
#77774=CARTESIAN_POINT ( 'NONE',  ( -3.078458344860000029, 1389.630721955109948, 203.0177346566789822 ) ) ;
#77785=CARTESIAN_POINT ( 'NONE',  ( -8.931786718119999691, 1380.912887613739940, 217.7591081930590065 ) ) ;
#77792=CARTESIAN_POINT ( 'NONE',  ( -10.50120379640000046, 1388.631521996640004, 201.9833518851789904 ) ) ;
#77804=CARTESIAN_POINT ( 'NONE',  ( -113.4000000000000057, 1389.413060387289988, 304.2218459572590064 ) ) ;
#77811=CARTESIAN_POINT ( 'NONE',  ( -11.51055856485790052, 1383.861746106490045, 218.7228895138829898 ) ) ;
#77820=CARTESIAN_POINT ( 'NONE',  ( -8.243035228590668950, 1386.658394140979681, 199.7856276493823486 ) ) ;
#77828=CARTESIAN_POINT ( 'NONE',  ( -12.97809200588160117, 1390.329422715150031, 212.5574397272170017 ) ) ;
#77831=CARTESIAN_POINT ( 'NONE',  ( -107.6978622682329814, 1380.365081504608042, 309.6627544237097709 ) ) ;
#77835=CARTESIAN_POINT ( 'NONE',  ( -67.25262833492540437, 1385.098311572419789, 260.0348044464020631 ) ) ;
#77896=CARTESIAN_POINT ( 'NONE',  ( -90.92465973820169722, 1384.842308400400043, 293.1021286165930064 ) ) ;
#77912=CARTESIAN_POINT ( 'NONE',  ( -110.0707497544257194, 1384.648932846942671, 296.9551064835548004 ) ) ;
#77914=CARTESIAN_POINT ( 'NONE',  ( -30.53571690079999712, 1379.628638755449856, 214.1212922363289977 ) ) ;
#77963=CARTESIAN_POINT ( 'NONE',  ( -68.78385482150279984, 1384.665972667470214, 293.6584164674959538 ) ) ;
#77964=CARTESIAN_POINT ( 'NONE',  ( -16.76289271049750340, 1384.945007802349892, 200.9261315889449975 ) ) ;
#77972=TOROIDAL_SURFACE ( 'NONE', #36815, 6.842541678089999913, 1.000000000000000000 ) ;
#77996=CARTESIAN_POINT ( 'NONE',  ( -65.80949023495340100, 1379.740780626450032, 276.1504492283160062 ) ) ;
#78002=CARTESIAN_POINT ( 'NONE',  ( -105.7961644359999980, 1379.239079028679953, 306.8423032396589747 ) ) ;
#78026=CARTESIAN_POINT ( 'NONE',  ( -48.92064667475605688, 1379.684638853033221, 237.5054648401685995 ) ) ;
#78032=CARTESIAN_POINT ( 'NONE',  ( -105.0203220942489963, 1379.361326776869873, 304.0304199180059754 ) ) ;
#78056=CARTESIAN_POINT ( 'NONE',  ( -89.79345263500000840, 1390.581174276010188, 301.0845629396590084 ) ) ;
#78069=FACE_OUTER_BOUND ( 'NONE', #83235, .T. ) ;
#78096=CARTESIAN_POINT ( 'NONE',  ( -19.47728386984950077, 1384.863915091259969, 220.7402890748070092 ) ) ;
#78150=CARTESIAN_POINT ( 'NONE',  ( -64.85694393360000731, 1378.892054699950222, 269.1292758489590256 ) ) ;
#78151=CARTESIAN_POINT ( 'NONE',  ( -106.0202621536679999, 1378.913060387289988, 302.8609204498379768 ) ) ;
#78156=CARTESIAN_POINT ( 'NONE',  ( -50.83427392639999454, 1384.622306023270085, 226.1831986462590010 ) ) ;
#78157=CARTESIAN_POINT ( 'NONE',  ( -63.63661578303909749, 1384.696032145409845, 252.0136171407070265 ) ) ;
#78159=CARTESIAN_POINT ( 'NONE',  ( -109.1462309409999989, 1385.214558625939844, 311.2612093662589814 ) ) ;
#78167=CARTESIAN_POINT ( 'NONE',  ( -68.73088892949999718, 1379.748097453069931, 280.1074355248589995 ) ) ;
#78178=CARTESIAN_POINT ( 'NONE',  ( -27.62594988560000075, 1384.837137189770147, 225.6315537474590371 ) ) ;
#78181=CARTESIAN_POINT ( 'NONE',  ( -14.28317992867999919, 1385.297258702939871, 219.2703623637189878 ) ) ;
#78192=CARTESIAN_POINT ( 'NONE',  ( -8.867335203187609594, 1385.164153589130137, 218.6750454735870051 ) ) ;
#78217=EDGE_CURVE ( 'NONE', #73589, #89045, #96554, .T. ) ;
#78227=CARTESIAN_POINT ( 'NONE',  ( -91.70122676012400120, 1383.769245710449923, 309.0451135184819691 ) ) ;
#78234=CARTESIAN_POINT ( 'NONE',  ( -73.68066259569999943, 1383.781794063629832, 298.8244620241590042 ) ) ;
#78245=CARTESIAN_POINT ( 'NONE',  ( -108.7558059640000039, 1382.069376407850086, 297.7710658298590261 ) ) ;
#78272=DIRECTION ( 'NONE',  ( -1.836970198721029688E-16, -1.000000000000000000, 0.000000000000000000 ) ) ;
#78308=CARTESIAN_POINT ( 'NONE',  ( -11.46335139447689855, 1391.913060387289988, 207.5095624942730126 ) ) ;
#78320=CARTESIAN_POINT ( 'NONE',  ( -3.078458351979999730, 1388.284543639960020, 200.7814874055890186 ) ) ;
#78333=CARTESIAN_POINT ( 'NONE',  ( -8.472397538460000987, 1381.589775986109998, 218.2249286227190055 ) ) ;
#78363=CARTESIAN_POINT ( 'NONE',  ( -27.67491638513010344, 1383.844931811260039, 225.5862836080119962 ) ) ;
#78373=CARTESIAN_POINT ( 'NONE',  ( -10.57956098816219459, 1390.295224638445688, 202.7063012876982668 ) ) ;
#78379=CARTESIAN_POINT ( 'NONE',  ( -14.32988524930309993, 1380.323806007950225, 209.8281070544639988 ) ) ;
#78385=CARTESIAN_POINT ( 'NONE',  ( -12.30520345314149822, 1377.738549314298552, 208.6947277391683144 ) ) ;
#78387=CARTESIAN_POINT ( 'NONE',  ( -11.15007135000000105, 1391.248055150329947, 203.8486859877390032 ) ) ;
#78388=CARTESIAN_POINT ( 'NONE',  ( -78.28007596846539684, 1385.150550643550105, 280.7138181926990228 ) ) ;
#78410=TOROIDAL_SURFACE ( 'NONE', #57006, 6.842541678089999913, 1.000000000000000000 ) ;
#78411=DIRECTION ( 'NONE',  ( -1.000000000000000000, 0.000000000000000000, 0.000000000000000000 ) ) ;
#78414=VECTOR ( 'NONE', #62767, 999.9999999999998863 ) ;
#78449=CARTESIAN_POINT ( 'NONE',  ( -100.3573076095590011, 1384.875324114890191, 296.3320123604629543 ) ) ;
#78466=CARTESIAN_POINT ( 'NONE',  ( -109.9754776966811392, 1384.008075049679974, 297.0180362684087640 ) ) ;
#78468=CARTESIAN_POINT ( 'NONE',  ( -21.16646057260000191, 1379.602502976239975, 209.5833567688460164 ) ) ;
#78472=CARTESIAN_POINT ( 'NONE',  ( -68.59216743299973018, 1379.747776907655634, 280.1820150774575495 ) ) ;
#78505=CARTESIAN_POINT ( 'NONE',  ( -12.31203607247529952, 1378.312412832470272, 208.4582867090369973 ) ) ;
#78509=EDGE_CURVE ( 'NONE', #46650, #110498, #96022, .T. ) ;
#78526=CARTESIAN_POINT ( 'NONE',  ( -64.31866039319710637, 1384.679996067239927, 287.7687853453900289 ) ) ;
#78527=CARTESIAN_POINT ( 'NONE',  ( -17.60051359271830052, 1384.946495389480106, 201.0930959932179860 ) ) ;
#78538=CARTESIAN_POINT ( 'NONE',  ( -106.7768089814430112, 1391.913060387289988, 306.1367433662150006 ) ) ;
#78543=CARTESIAN_POINT ( 'NONE',  ( -9.916501125940001771, 1380.324599945550062, 201.6733442065789745 ) ) ;
#78554=CARTESIAN_POINT ( 'NONE',  ( -64.29128857122019269, 1379.736509255219971, 273.6614271908390492 ) ) ;
#78561=CARTESIAN_POINT ( 'NONE',  ( -105.3679517439999955, 1379.024053303089886, 305.1804760158589716 ) ) ;
#78583=CARTESIAN_POINT ( 'NONE',  ( -7.769371101339999974, 1384.910032728360193, 218.9178649038489937 ) ) ;
#78587=CARTESIAN_POINT ( 'NONE',  ( -34.88314824369056311, 1379.640034327572494, 217.8691061211530382 ) ) ;
#78617=CARTESIAN_POINT ( 'NONE',  ( -97.51726726849999238, 1390.553429058280017, 303.6087006878590273 ) ) ;
#78629=CARTESIAN_POINT ( 'NONE',  ( -105.6749141713339952, 1378.070069343479872, 305.5932407599049725 ) ) ;
#78656=CARTESIAN_POINT ( 'NONE',  ( -22.14384457810140105, 1384.855528056009916, 221.9556210832379861 ) ) ;
#78662=EDGE_LOOP ( 'NONE', ( #83917, #38562, #63102, #92340, #25512, #90064, #5430, #85883, #107116 ) ) ;
#78713=CARTESIAN_POINT ( 'NONE',  ( -94.35247987469999487, 1379.531630663759870, 302.8771378034590498 ) ) ;
#78718=CARTESIAN_POINT ( 'NONE',  ( -106.7752590979999923, 1385.237353006989906, 297.1314966531590471 ) ) ;
#78719=CARTESIAN_POINT ( 'NONE',  ( -53.13991455628549687, 1384.634500711259989, 230.4819378445650102 ) ) ;
#78732=CARTESIAN_POINT ( 'NONE',  ( -67.70136529139999482, 1379.745769832329870, 277.8225302446590490 ) ) ;
#78733=CARTESIAN_POINT ( 'NONE',  ( -109.9849726248329915, 1384.916895159399928, 311.4561123681800154 ) ) ;
#78740=CARTESIAN_POINT ( 'NONE',  ( -32.09555170170000338, 1384.821019989420165, 229.9571600258589967 ) ) ;
#78789=CARTESIAN_POINT ( 'NONE',  ( -97.83732743130200049, 1383.765384414209848, 310.3688010583850314 ) ) ;
#78790=CARTESIAN_POINT ( 'NONE',  ( -109.2723729720279948, 1384.466068673930067, 311.2384636710350492 ) ) ;
#78797=CARTESIAN_POINT ( 'NONE',  ( -66.86281825880000440, 1379.216504766910020, 275.7591398340589990 ) ) ;
#78807=DIRECTION ( 'NONE',  ( 0.8090169943747088643, 0.000000000000000000, 0.5877852522928015411 ) ) ;
#78809=CARTESIAN_POINT ( 'NONE',  ( -107.2362392430000000, 1382.245772082230133, 298.1239918761589820 ) ) ;
#78811=DIRECTION ( 'NONE',  ( -0.05490754757727549923, 0.004515313913275745793, -0.9984812332534417356 ) ) ;
#78820=EDGE_LOOP ( 'NONE', ( #14909, #6283, #16831, #83727, #20662, #103484 ) ) ;
#78837=AXIS2_PLACEMENT_3D ( 'NONE', #101927, #93530, #25770 ) ;
#78866=ORIENTED_EDGE ( 'NONE', *, *, #92525, .T. ) ;
#78883=CARTESIAN_POINT ( 'NONE',  ( -11.66938051635290208, 1391.913060387229962, 209.0107206413649976 ) ) ;
#78893=CARTESIAN_POINT ( 'NONE',  ( -50.70014224199999830, 1389.561552466730063, 232.3334791991590009 ) ) ;
#78899=CARTESIAN_POINT ( 'NONE',  ( -14.01398736212220086, 1379.590348564800024, 211.9184487047760115 ) ) ;
#78917=CARTESIAN_POINT ( 'NONE',  ( -12.31911163787790109, 1378.288338451009849, 209.5493042496160001 ) ) ;
#78931=CARTESIAN_POINT ( 'NONE',  ( -35.19207028348809985, 1383.835214657470260, 234.1679424143649726 ) ) ;
#78937=VERTEX_POINT ( 'NONE', #95285 ) ;
#78940=EDGE_CURVE ( 'NONE', #88625, #43749, #48362, .T. ) ;
#78941=CARTESIAN_POINT ( 'NONE',  ( -10.18734585702747886, 1389.825619450207569, 202.1025026781494205 ) ) ;
#78946=ORIENTED_EDGE ( 'NONE', *, *, #1915, .T. ) ;
#78948=CARTESIAN_POINT ( 'NONE',  ( -13.37269592510800109, 1390.548568132430091, 209.7987342400010107 ) ) ;
#78957=CARTESIAN_POINT ( 'NONE',  ( -101.8647915021330022, 1385.225522266660164, 296.5844919615699951 ) ) ;
#79011=ORIENTED_EDGE ( 'NONE', *, *, #37130, .F. ) ;
#79038=CARTESIAN_POINT ( 'NONE',  ( -30.36057678899999601, 1379.678206996359904, 214.3682391549489807 ) ) ;
#79042=CARTESIAN_POINT ( 'NONE',  ( -67.68653639037678715, 1379.747580689172310, 278.9655481580869036 ) ) ;
#79061=CARTESIAN_POINT ( 'NONE',  ( -109.1312182564879976, 1384.932234318600194, 313.2646789733740320 ) ) ;
#79079=CARTESIAN_POINT ( 'NONE',  ( -7.616835117835059954, 1383.928091763239991, 219.0006089918529995 ) ) ;
#79091=CARTESIAN_POINT ( 'NONE',  ( -74.12207176259649088, 1384.651791245910090, 299.2615222811550098 ) ) ;
#79092=CARTESIAN_POINT ( 'NONE',  ( -29.17863452356749931, 1384.967235213910044, 205.1305293287510096 ) ) ;
#79098=CARTESIAN_POINT ( 'NONE',  ( -8.848352231939999868, 1384.927997118699750, 199.9247642750889895 ) ) ;
#79106=CARTESIAN_POINT ( 'NONE',  ( -106.6090143111130004, 1391.913060387289988, 305.6150165752750354 ) ) ;
#79110=CARTESIAN_POINT ( 'NONE',  ( -9.131333920219999456, 1383.714870296950039, 200.1584639485390085 ) ) ;
#79122=CARTESIAN_POINT ( 'NONE',  ( -67.15060528540000462, 1379.747519056979854, 278.1647121851589759 ) ) ;
#79135=CARTESIAN_POINT ( 'NONE',  ( -105.9863851607009906, 1378.913060388959821, 305.2978657741859934 ) ) ;
#79149=CARTESIAN_POINT ( 'NONE',  ( -7.545227633159999669, 1384.915097837209942, 219.0875773561589881 ) ) ;
#79154=CARTESIAN_POINT ( 'NONE',  ( -42.46926378087947995, 1379.662295881295449, 226.7269345055754854 ) ) ;
#79158=ORIENTED_EDGE ( 'NONE', *, *, #92525, .F. ) ;
#79167=CARTESIAN_POINT ( 'NONE',  ( -57.30544179059780419, 1379.717622275232316, 260.4455970689041351 ) ) ;
#79186=CARTESIAN_POINT ( 'NONE',  ( -98.66388059649999320, 1388.280417272740124, 297.3587652689590186 ) ) ;
#79197=CARTESIAN_POINT ( 'NONE',  ( -103.7134603450270021, 1379.995765815970117, 305.6207973536889995 ) ) ;
#79222=CARTESIAN_POINT ( 'NONE',  ( -22.88685215929439920, 1384.853117157140105, 222.3623658345020146 ) ) ;
#79275=CARTESIAN_POINT ( 'NONE',  ( -78.35932141380000360, 1379.348932152990074, 291.3894706377590182 ) ) ;
#79277=CARTESIAN_POINT ( 'NONE',  ( -106.2764360894749984, 1378.913060387289988, 302.2763280471240250 ) ) ;
#79287=CARTESIAN_POINT ( 'NONE',  ( -13.36083802519999963, 1384.539077642469920, 218.9649430346489964 ) ) ;
#79292=CARTESIAN_POINT ( 'NONE',  ( -66.43975051640001084, 1379.742919361219947, 275.2749399108590183 ) ) ;
#79300=CARTESIAN_POINT ( 'NONE',  ( -32.09327717010000214, 1384.955453299609871, 229.9590027138590074 ) ) ;
#79302=CARTESIAN_POINT ( 'NONE',  ( -26.97945814876269921, 1385.247242750549958, 225.1983066302449856 ) ) ;
#79341=DIRECTION ( 'NONE',  ( -1.000000000000000000, 0.000000000000000000, 0.000000000000000000 ) ) ;
#79345=CARTESIAN_POINT ( 'NONE',  ( -79.77560727129458940, 1383.777144559889848, 303.5005229431759517 ) ) ;
#79346=CARTESIAN_POINT ( 'NONE',  ( -109.8098934281339893, 1384.480849638239988, 311.3605537058619461 ) ) ;
#79353=CARTESIAN_POINT ( 'NONE',  ( -88.69635973610000690, 1381.890970305359815, 292.9935112231589756 ) ) ;
#79358=CARTESIAN_POINT ( 'NONE',  ( -109.1656556500000050, 1384.956445634750025, 297.1328572680590128 ) ) ;
#79383=FACE_OUTER_BOUND ( 'NONE', #84069, .T. ) ;
#79436=CARTESIAN_POINT ( 'NONE',  ( -39.74720592359999927, 1386.640108147219962, 212.4723510803390241 ) ) ;
#79442=CARTESIAN_POINT ( 'NONE',  ( -14.03675672165638311, 1379.586046047017817, 211.8650569067899880 ) ) ;
#79444=CARTESIAN_POINT ( 'NONE',  ( -7.880843563809999175, 1383.349707206300081, 218.7727698555990230 ) ) ;
#79465=CARTESIAN_POINT ( 'NONE',  ( -105.7715868071176004, 1391.141956858045887, 306.3730018047383510 ) ) ;
#79475=CARTESIAN_POINT ( 'NONE',  ( -22.22211278303320015, 1383.851195146140071, 221.8019234694140209 ) ) ;
#79485=CARTESIAN_POINT ( 'NONE',  ( -8.346053580011268735, 1386.932765083509366, 199.8874523339913765 ) ) ;
#79492=CARTESIAN_POINT ( 'NONE',  ( -12.31705391887590118, 1391.331872793070033, 211.5890497232870189 ) ) ;
#79501=CARTESIAN_POINT ( 'NONE',  ( -104.2741735075869940, 1385.231329888970095, 296.8622915881020390 ) ) ;
#79553=ADVANCED_FACE ( 'NONE', ( #62557 ), #44241, .T. ) ;
#79562=CARTESIAN_POINT ( 'NONE',  ( -108.8816724165859995, 1384.900720007879954, 297.1232481292220200 ) ) ;
#79577=CARTESIAN_POINT ( 'NONE',  ( -109.1450416020000063, 1385.242479493820156, 297.1468691531589457 ) ) ;
#79584=CARTESIAN_POINT ( 'NONE',  ( -29.90839080445297782, 1379.722162689491142, 217.8816187646463902 ) ) ;
#79587=EDGE_LOOP ( 'NONE', ( #55160, #75263, #103753, #4186 ) ) ;
#79590=CARTESIAN_POINT ( 'NONE',  ( -74.95997362772719441, 1385.008095471610204, 300.0149541100690271 ) ) ;
#79594=CARTESIAN_POINT ( 'NONE',  ( -8.162204519790000390, 1384.930475412839996, 199.6393846580689910 ) ) ;
#79609=ADVANCED_FACE ( 'NONE', ( #90880 ), #108789, .T. ) ;
#79620=CARTESIAN_POINT ( 'NONE',  ( -13.74068978706669952, 1379.630235450999862, 208.0692380938309896 ) ) ;
#79642=CARTESIAN_POINT ( 'NONE',  ( -103.2712462040139911, 1384.594671018880035, 311.0952753235899877 ) ) ;
#79643=CARTESIAN_POINT ( 'NONE',  ( -40.62403037922339877, 1384.991413212550015, 213.4871031860279800 ) ) ;
#79661=CARTESIAN_POINT ( 'NONE',  ( -13.53579909870000009, 1380.123783341879971, 205.1599962651189912 ) ) ;
#79672=CARTESIAN_POINT ( 'NONE',  ( -64.33487710937569659, 1379.738747083599947, 273.6361551471470079 ) ) ;
#79673=ORIENTED_EDGE ( 'NONE', *, *, #19247, .F. ) ;
#79693=CARTESIAN_POINT ( 'NONE',  ( -10.53295592549999959, 1391.913060387289988, 204.1405351054689845 ) ) ;
#79701=CARTESIAN_POINT ( 'NONE',  ( -7.545064063079999883, 1384.907232460160003, 219.0876311382089909 ) ) ;
#79704=CARTESIAN_POINT ( 'NONE',  ( -66.34541600742676337, 1379.742690955398075, 275.0820465578231619 ) ) ;
#79716=CARTESIAN_POINT ( 'NONE',  ( -32.12438293513578458, 1379.634397414435625, 220.1697278361670271 ) ) ;
#79722=DIRECTION ( 'NONE',  ( -3.247745162871014848E-19, -1.000000000000000000, -7.717164782866489769E-18 ) ) ;
#79733=CARTESIAN_POINT ( 'NONE',  ( -103.7270236659999938, 1386.773311355200121, 297.0694254661589753 ) ) ;
#79747=CARTESIAN_POINT ( 'NONE',  ( -106.2248512509999898, 1379.716103201010128, 307.8123243076590256 ) ) ;
#79774=CARTESIAN_POINT ( 'NONE',  ( -33.85357780581230003, 1384.813694486169879, 232.6238098525020064 ) ) ;
#79797=CARTESIAN_POINT ( 'NONE',  ( -47.85632535846249880, 1378.658246217350097, 243.6236061017949908 ) ) ;
#79807=CARTESIAN_POINT ( 'NONE',  ( -7.811670192970000315, 1384.136991477590072, 218.8584676683489931 ) ) ;
#79829=CARTESIAN_POINT ( 'NONE',  ( -64.29757574260000297, 1379.513720862740229, 269.4006999320590126 ) ) ;
#79831=CARTESIAN_POINT ( 'NONE',  ( -106.0563374611769945, 1378.913060387289988, 302.7607369287470078 ) ) ;
#79845=CARTESIAN_POINT ( 'NONE',  ( -66.60970852960001309, 1379.742673636729933, 275.7100306615589602 ) ) ;
#79855=CARTESIAN_POINT ( 'NONE',  ( -35.77507902226459890, 1385.205099667260129, 235.2908270135410191 ) ) ;
#79899=CARTESIAN_POINT ( 'NONE',  ( -84.93366321518800532, 1383.773587948340264, 306.4644327478220589 ) ) ;
#79900=CARTESIAN_POINT ( 'NONE',  ( -109.5468108793060082, 1383.526318514589775, 311.1941293573789835 ) ) ;
#79905=ORIENTED_EDGE ( 'NONE', *, *, #106358, .F. ) ;
#79906=CARTESIAN_POINT ( 'NONE',  ( -73.92520625790000111, 1379.263703378919899, 287.0831489011590065 ) ) ;
#79907=PLANE ( 'NONE',  #96213 ) ;
#79911=CARTESIAN_POINT ( 'NONE',  ( -109.3504194409999855, 1384.949684486699880, 297.1387111212590071 ) ) ;
#79923=DIRECTION ( 'NONE',  ( -1.000000000000000000, 0.000000000000000000, 0.000000000000000000 ) ) ;
#79979=CARTESIAN_POINT ( 'NONE',  ( -31.91283005400000050, 1386.630794634020049, 206.3242904142690008 ) ) ;
#80004=CARTESIAN_POINT ( 'NONE',  ( -109.8796183239999920, 1385.344994265080004, 297.0482512251589924 ) ) ;
#80007=CARTESIAN_POINT ( 'NONE',  ( -105.4653109980351076, 1391.248289814977625, 304.9316009898920470 ) ) ;
#80018=CARTESIAN_POINT ( 'NONE',  ( -21.83573956349999889, 1383.851617847329862, 221.6010342889879894 ) ) ;
#80026=CARTESIAN_POINT ( 'NONE',  ( -3.078458294050000266, 1383.868666969369770, 218.4015365393190109 ) ) ;
#80032=CARTESIAN_POINT ( 'NONE',  ( -9.309222779429999761, 1389.084088572969904, 217.3257696767689993 ) ) ;
#80040=CARTESIAN_POINT ( 'NONE',  ( -90.07212409636069594, 1385.192969068609955, 292.6181576655579875 ) ) ;
#80058=CARTESIAN_POINT ( 'NONE',  ( -8.021592841849999544, 1384.982153790620032, 218.7868050085690186 ) ) ;
#80062=CARTESIAN_POINT ( 'NONE',  ( -103.6168536339999946, 1379.900079317219934, 303.2097866628589600 ) ) ;
#80121=CARTESIAN_POINT ( 'NONE',  ( -76.22128121885890550, 1385.004381994479900, 301.0818327933589558 ) ) ;
#80131=CARTESIAN_POINT ( 'NONE',  ( -11.66658784013729999, 1391.913060387289988, 209.7120188154370339 ) ) ;
#80148=CARTESIAN_POINT ( 'NONE',  ( -13.57853027955069969, 1379.569703739710121, 207.8817176012079813 ) ) ;
#80155=CARTESIAN_POINT ( 'NONE',  ( -7.606524257758859875, 1383.989784261539853, 219.0105849715669990 ) ) ;
#80173=CARTESIAN_POINT ( 'NONE',  ( -91.22755695539819953, 1384.616955451200056, 309.0857609642320085 ) ) ;
#80175=CARTESIAN_POINT ( 'NONE',  ( -29.90545723663199951, 1384.968601192589858, 205.5110789169119982 ) ) ;
#80176=CARTESIAN_POINT ( 'NONE',  ( -5.364792434415069700, 1374.934204522590107, 214.8728634718659976 ) ) ;
#80183=CARTESIAN_POINT ( 'NONE',  ( -8.848156404039999146, 1384.935949319609790, 199.9247822318290275 ) ) ;
#80191=CARTESIAN_POINT ( 'NONE',  ( -106.5816461138369959, 1391.913060387289988, 305.5142355297590484 ) ) ;
#80195=CARTESIAN_POINT ( 'NONE',  ( -12.46974414340000159, 1379.786009550329936, 205.4121433733889717 ) ) ;
#80207=CARTESIAN_POINT ( 'NONE',  ( -68.39881485729999611, 1379.747709036749939, 279.9507912016590012 ) ) ;
#80214=CARTESIAN_POINT ( 'NONE',  ( -109.3083906640000009, 1384.947550057740045, 311.2644960252590067 ) ) ;
#80236=CARTESIAN_POINT ( 'NONE',  ( -7.769424639409999500, 1384.914898569509887, 218.9178468150989829 ) ) ;
#80240=CARTESIAN_POINT ( 'NONE',  ( -13.20210775350000176, 1379.610108467780037, 208.3538038533539805 ) ) ;
#80241=CARTESIAN_POINT ( 'NONE',  ( -66.84334151430192605, 1379.743858467100608, 276.0920115519006686 ) ) ;
#80264=CARTESIAN_POINT ( 'NONE',  ( -103.8568841305003190, 1379.883889493366269, 304.0042906413861488 ) ) ;
#80276=CARTESIAN_POINT ( 'NONE',  ( -106.7468999319999909, 1388.280083271419926, 298.2446700897589835 ) ) ;
#80287=CARTESIAN_POINT ( 'NONE',  ( -107.1583685770000045, 1380.648470457769918, 309.2260028292590164 ) ) ;
#80312=CARTESIAN_POINT ( 'NONE',  ( -27.25125854287810157, 1384.838333352839982, 225.4489716181609822 ) ) ;
#80330=DIRECTION ( 'NONE',  ( 1.835183309750130004E-16, 1.000000000000000000, 1.599799320660000123E-19 ) ) ;
#80338=CARTESIAN_POINT ( 'NONE',  ( -70.83845563213419894, 1379.712669723569888, 285.7529926274859804 ) ) ;
#80348=CARTESIAN_POINT ( 'NONE',  ( -7.540598407700000116, 1384.733204023860026, 219.0853623458990000 ) ) ;
#80357=CARTESIAN_POINT ( 'NONE',  ( 12.33128373348028184, 1390.939237335599955, 208.6028876581396503 ) ) ;
#80368=AXIS2_PLACEMENT_3D ( 'NONE', #75181, #61008, #44190 ) ;
#80374=CARTESIAN_POINT ( 'NONE',  ( -101.8495347479999964, 1374.485289779690220, 303.2301490391590164 ) ) ;
#80379=CARTESIAN_POINT ( 'NONE',  ( -98.86936394900000380, 1384.986782500260006, 296.2451545551589902 ) ) ;
#80391=CARTESIAN_POINT ( 'NONE',  ( -65.41912593600000037, 1379.740434417399683, 273.1837229148590609 ) ) ;
#80400=CARTESIAN_POINT ( 'NONE',  ( -89.65362972180000156, 1384.619809472219913, 308.7387643915590161 ) ) ;
#80401=ORIENTED_EDGE ( 'NONE', *, *, #4893, .F. ) ;
#80402=CARTESIAN_POINT ( 'NONE',  ( -24.85901358151489760, 1385.256427123100138, 223.5815164292420150 ) ) ;
#80435=CARTESIAN_POINT ( 'NONE',  ( -103.5847285859999971, 1379.882004272549921, 303.6035322816589996 ) ) ;
#80449=CARTESIAN_POINT ( 'NONE',  ( -83.79005405282170216, 1383.774350621089980, 305.8889031002050274 ) ) ;
#80450=CARTESIAN_POINT ( 'NONE',  ( -109.8447538101560070, 1383.797388995159963, 311.3561482245430057 ) ) ;
#80455=CARTESIAN_POINT ( 'NONE',  ( -96.58293600380000044, 1381.030388059910138, 308.7257624848589899 ) ) ;
#80460=CARTESIAN_POINT ( 'NONE',  ( -109.5358690449999983, 1384.943159195940098, 297.1231912513590032 ) ) ;
#80471=CARTESIAN_POINT ( 'NONE',  ( -107.2899050854710055, 1379.886892357829993, 309.1794776302379546 ) ) ;
#80560=CARTESIAN_POINT ( 'NONE',  ( -109.8984563230000049, 1385.013959313279884, 297.0294149341589787 ) ) ;
#80570=CARTESIAN_POINT ( 'NONE',  ( -25.20965598612449909, 1383.847833833380037, 223.6406741977980062 ) ) ;
#80579=CARTESIAN_POINT ( 'NONE',  ( -20.79832720279999947, 1379.854941608700074, 216.4077191293589806 ) ) ;
#80586=CARTESIAN_POINT ( 'NONE',  ( -10.72558049390000079, 1390.998992605100057, 215.2615596033689940 ) ) ;
#80587=CARTESIAN_POINT ( 'NONE',  ( -10.57298823631211526, 1391.449726738521349, 215.2582967309260766 ) ) ;
#80595=CARTESIAN_POINT ( 'NONE',  ( -96.47871924218719641, 1385.211633195850027, 295.4357730181330339 ) ) ;
#80620=CARTESIAN_POINT ( 'NONE',  ( -106.3258853770000059, 1381.775203003109937, 298.5533487220590132 ) ) ;
#80638=ORIENTED_EDGE ( 'NONE', *, *, #22945, .T. ) ;
#80639=CARTESIAN_POINT ( 'NONE',  ( 2.405030274568579469E-16, 1384.770513348110171, 199.6218459572590120 ) ) ;
#80641=ORIENTED_EDGE ( 'NONE', *, *, #108446, .T. ) ;
#80653=AXIS2_PLACEMENT_3D ( 'NONE', #37702, #79722, #4117 ) ;
#80657=ORIENTED_EDGE ( 'NONE', *, *, #85625, .F. ) ;
#80671=CARTESIAN_POINT ( 'NONE',  ( -106.1577809140989928, 1391.913060435339958, 304.2026313505140251 ) ) ;
#80672=CARTESIAN_POINT ( 'NONE',  ( -68.07780588645262299, 1379.747638516087818, 279.5234925689441070 ) ) ;
#80679=CARTESIAN_POINT ( 'NONE',  ( -88.81082328880501109, 1384.972301615300012, 308.2983196932370333 ) ) ;
#80727=CARTESIAN_POINT ( 'NONE',  ( -93.65288495826759174, 1384.612519065399965, 309.7350186990149723 ) ) ;
#80728=CARTESIAN_POINT ( 'NONE',  ( -44.16285280505819344, 1385.000714628640026, 217.3125100336829973 ) ) ;
#80734=ORIENTED_EDGE ( 'NONE', *, *, #96614, .T. ) ;
#80735=CARTESIAN_POINT ( 'NONE',  ( -109.8253217000000035, 1384.908747186490018, 311.3807772092590085 ) ) ;
#80743=CARTESIAN_POINT ( 'NONE',  ( -107.2344095241460025, 1391.913060387289988, 307.1919084200470138 ) ) ;
#80747=CARTESIAN_POINT ( 'NONE',  ( -12.26760366359999921, 1381.106678608419998, 202.8726028786589950 ) ) ;
#80760=CARTESIAN_POINT ( 'NONE',  ( -67.83249339340770234, 1379.746683816080122, 279.1961202499749675 ) ) ;
#80766=CARTESIAN_POINT ( 'NONE',  ( -109.6582946740000040, 1384.935989956509957, 311.3230066222590153 ) ) ;
#80791=CARTESIAN_POINT ( 'NONE',  ( -68.16989581615023042, 1379.746757633565267, 278.7814004105860022 ) ) ;
#80796=CARTESIAN_POINT ( 'NONE',  ( -66.13828525536300162, 1384.712330930560029, 257.5898851940499981 ) ) ;
#80822=CARTESIAN_POINT ( 'NONE',  ( -109.9987472859999968, 1389.231820704839947, 308.7519488593589472 ) ) ;
#80833=CARTESIAN_POINT ( 'NONE',  ( -104.2932360906780076, 1380.188221978170077, 306.6001351807259994 ) ) ;
#80862=CARTESIAN_POINT ( 'NONE',  ( -30.60972296751670285, 1384.826188984249939, 228.7072743885399859 ) ) ;
#80864=CARTESIAN_POINT ( 'NONE',  ( -105.3716458700000089, 1379.306619424940209, 302.1984682570590053 ) ) ;
#80886=CARTESIAN_POINT ( 'NONE',  ( -60.74530810509999412, 1376.530688957809843, 271.1243785565590088 ) ) ;
#80896=CARTESIAN_POINT ( 'NONE',  ( -105.5745580539999935, 1391.578493776289861, 304.2150181189589944 ) ) ;
#80917=CARTESIAN_POINT ( 'NONE',  ( -13.09461299200390094, 1380.098038397369919, 209.6821016411979883 ) ) ;
#80920=CARTESIAN_POINT ( 'NONE',  ( -50.85477211400000641, 1375.010081756269983, 242.1550097575589859 ) ) ;
#80926=CARTESIAN_POINT ( 'NONE',  ( -94.50989921500000435, 1384.972694751829977, 294.8597475345590055 ) ) ;
#80932=CARTESIAN_POINT ( 'NONE',  ( -13.36052273939999857, 1384.881792980340151, 218.9673617354289945 ) ) ;
#80937=CARTESIAN_POINT ( 'NONE',  ( -67.96433663839999895, 1379.748578009009861, 278.4994408155590122 ) ) ;
#80945=CARTESIAN_POINT ( 'NONE',  ( -81.17714880479999806, 1384.872208132610012, 304.9620800596590016 ) ) ;
#80947=CARTESIAN_POINT ( 'NONE',  ( -20.99389299076310067, 1385.272353955699828, 221.3600716116459921 ) ) ;
#80975=CARTESIAN_POINT ( 'NONE',  ( -106.0221095560000037, 1391.653194082120081, 301.9380359125589735 ) ) ;
#80981=DIRECTION ( 'NONE',  ( -1.836970198721029688E-16, -1.000000000000000000, 0.000000000000000000 ) ) ;
#80993=CARTESIAN_POINT ( 'NONE',  ( -109.5761286768430125, 1384.171525062670071, 311.2610357945890200 ) ) ;
#81001=FACE_OUTER_BOUND ( 'NONE', #47325, .T. ) ;
#81006=CARTESIAN_POINT ( 'NONE',  ( -109.4427638259999895, 1384.881580825830042, 297.1256396965589488 ) ) ;
#81043=CARTESIAN_POINT ( 'NONE',  ( -23.72302164034240235, 1384.541713701390108, 202.8184092090419881 ) ) ;
#81071=CARTESIAN_POINT ( 'NONE',  ( -9.113128543256529213, 1384.565653361969908, 199.9635744024730002 ) ) ;
#81106=CARTESIAN_POINT ( 'NONE',  ( -46.55794552509269835, 1383.817606665970061, 254.2825134048519828 ) ) ;
#81114=CARTESIAN_POINT ( 'NONE',  ( -39.75532303620000363, 1384.581637800209819, 212.4630896483189701 ) ) ;
#81120=CARTESIAN_POINT ( 'NONE',  ( -8.424900129770140467, 1387.809024083920121, 218.2696960641690112 ) ) ;
#81131=CARTESIAN_POINT ( 'NONE',  ( -68.75983579849153671, 1379.748052159727195, 280.1905170100664577 ) ) ;
#81144=CARTESIAN_POINT ( 'NONE',  ( -109.1320112420000044, 1384.953741877159700, 311.2644403302589353 ) ) ;
#81154=CARTESIAN_POINT ( 'NONE',  ( -8.299200653989998955, 1385.160822377860086, 218.6946808916390239 ) ) ;
#81174=CARTESIAN_POINT ( 'NONE',  ( -3.078458355159999993, 1384.635588543570066, 199.6791145954990156 ) ) ;
#81178=CARTESIAN_POINT ( 'NONE',  ( -106.3126565290000087, 1379.599899938080171, 307.8895711306589646 ) ) ;
#81203=FACE_OUTER_BOUND ( 'NONE', #94820, .T. ) ;
#81204=CARTESIAN_POINT ( 'NONE',  ( -52.42853552574362652, 1379.742143312621693, 249.9106425968767553 ) ) ;
#81211=CARTESIAN_POINT ( 'NONE',  ( -99.13733263931901263, 1384.948377550129862, 310.7311109629659427 ) ) ;
#81213=CARTESIAN_POINT ( 'NONE',  ( -10.27296164000000012, 1387.820157591719862, 201.2959240949089974 ) ) ;
#81216=ORIENTED_EDGE ( 'NONE', *, *, #72721, .F. ) ;
#81256=CARTESIAN_POINT ( 'NONE',  ( -92.84358858088950228, 1384.613997830719882, 309.5363385667750435 ) ) ;
#81257=CARTESIAN_POINT ( 'NONE',  ( -42.51724257030390675, 1384.996239121569943, 215.4468276199860099 ) ) ;
#81263=ORIENTED_EDGE ( 'NONE', *, *, #70155, .F. ) ;
#81264=CARTESIAN_POINT ( 'NONE',  ( -109.4837766770000087, 1384.913273580270015, 311.2841394952590122 ) ) ;
#81275=CARTESIAN_POINT ( 'NONE',  ( -10.78481250609999975, 1379.886398380170021, 203.0395362228890122 ) ) ;
#81288=TOROIDAL_SURFACE ( 'NONE', #75947, 7.499828603750000156, 0.5000000000000000000 ) ;
#81289=CARTESIAN_POINT ( 'NONE',  ( -67.64859488819530497, 1379.745247417349901, 278.9922900543069773 ) ) ;
#81300=CARTESIAN_POINT ( 'NONE',  ( -107.2277229851110008, 1378.913060387289988, 307.4948507977209715 ) ) ;
#81308=CARTESIAN_POINT ( 'NONE',  ( -10.81222349729999976, 1391.793768475530214, 204.0084625770589923 ) ) ;
#81316=CARTESIAN_POINT ( 'NONE',  ( -66.36196940094187369, 1379.742730262553778, 275.1157302125421893 ) ) ;
#81321=CARTESIAN_POINT ( 'NONE',  ( -60.61372366948459955, 1384.676785248499982, 245.3352954287460079 ) ) ;
#81382=CARTESIAN_POINT ( 'NONE',  ( -36.40840158213870126, 1384.803230251859986, 236.2568994546979866 ) ) ;
#81384=CARTESIAN_POINT ( 'NONE',  ( -105.3073167809999973, 1379.015836308379903, 304.0377958964590448 ) ) ;
#81405=CARTESIAN_POINT ( 'NONE',  ( -61.17467505917599624, 1379.375923620560116, 270.9160354019339820 ) ) ;
#81417=CARTESIAN_POINT ( 'NONE',  ( -8.860690249450000167, 1384.665722157209984, 218.6783682169690053 ) ) ;
#81423=DIRECTION ( 'NONE',  ( -1.000000000000000000, 0.000000000000000000, 0.000000000000000000 ) ) ;
#81441=CARTESIAN_POINT ( 'NONE',  ( -57.85314987360000316, 1379.895658628149931, 259.2190729278590311 ) ) ;
#81443=CONICAL_SURFACE ( 'NONE', #40287, 0.9999999999999857891, 0.7853981633970000820 ) ;
#81458=CARTESIAN_POINT ( 'NONE',  ( -59.24835266110000020, 1384.395332261929980, 279.9182260145590249 ) ) ;
#81462=CARTESIAN_POINT ( 'NONE',  ( -54.39340494969999895, 1379.701756400480008, 248.9505162619590237 ) ) ;
#81471=EDGE_CURVE ( 'NONE', #105885, #48821, #20291, .T. ) ;
#81472=CARTESIAN_POINT ( 'NONE',  ( -106.4197298790000019, 1384.588767362379940, 311.3121942672589739 ) ) ;
#81474=CARTESIAN_POINT ( 'NONE',  ( -26.15713872745329738, 1385.250841378830046, 224.5366954647260229 ) ) ;
#81478=TOROIDAL_SURFACE ( 'NONE', #33209, 11.26398391340000060, 1.000000000000000000 ) ;
#81501=CARTESIAN_POINT ( 'NONE',  ( -107.6645298440000005, 1388.788267583639936, 298.6282682945589499 ) ) ;
#81518=CARTESIAN_POINT ( 'NONE',  ( -8.888758267720000106, 1385.314821192629779, 218.6605176881890031 ) ) ;
#81526=CARTESIAN_POINT ( 'NONE',  ( -109.9987473139999992, 1380.796323439529942, 299.4245717883589464 ) ) ;
#81531=CARTESIAN_POINT ( 'NONE',  ( -109.8947179409999961, 1384.912517356189937, 297.0284612775590176 ) ) ;
#81578=EDGE_CURVE ( 'NONE', #108323, #60994, #90885, .T. ) ;
#81587=ORIENTED_EDGE ( 'NONE', *, *, #108446, .F. ) ;
#81596=CARTESIAN_POINT ( 'NONE',  ( -68.77833046130001549, 1379.747972053160083, 280.2623328013589799 ) ) ;
#81643=EDGE_CURVE ( 'NONE', #7882, #94821, #106964, .T. ) ;
#81645=CARTESIAN_POINT ( 'NONE',  ( -51.45124350130279822, 1383.809539065679928, 264.3240461168200000 ) ) ;
#81653=CARTESIAN_POINT ( 'NONE',  ( -16.29753011569999899, 1382.961179775240225, 200.7913250421689781 ) ) ;
#81659=CARTESIAN_POINT ( 'NONE',  ( -11.02704084530000017, 1390.246027334430210, 215.0626141722390230 ) ) ;
#81670=CARTESIAN_POINT ( 'NONE',  ( -67.40081635460001053, 1379.748791505480085, 277.3949072269590488 ) ) ;
#81682=CARTESIAN_POINT ( 'NONE',  ( -109.3508372059999942, 1385.551281695979924, 311.2426504422589915 ) ) ;
#81686=B_SPLINE_CURVE_WITH_KNOTS ( 'NONE', 3,
 ( #18652, #45009, #247, #10267, #52301, #53972, #86426, #61814, #35473, #9716, #68547, #78587, #102647, #44443, #27627, #51740, #60707, #69664, #25947, #60142, #76936, #95937, #19197, #79154, #1903, #36041, #42776, #86978, #43882, #9176, #43341, #78026, #62365, #52851, #96490, #2463, #1333, #103787, #77489, #27088, #61272, #70229, #53399, #95387, #88104, #87549, #789, #10838, #34374, #104334, #28180, #94262, #26510, #17538, #36579, #70777, #104889, #85874, #34918, #69104, #103205, #22489, #46659, #56133, #105445, #4631, #107636, #3560, #11931, #28733, #47736, #71887, #90267, #106002, #65098, #13005, #13550, #30370, #107081, #64011, #56690, #98122, #11393, #46110, #79704, #62939, #97590, #81316, #29278, #55607, #80241, #81871, #89731, #63471, #20862, #89183, #106535, #97050, #29824, #99210, #45563, #55057, #54518, #5172, #37682, #12477, #80791, #20313, #21397, #4098, #38222, #38769, #3009, #30919, #37132, #88653, #72404, #47191, #72943, #64559, #98678 ),
 .UNSPECIFIED., .F., .F.,
 ( 4, 2, 2, 2, 2, 2, 1, 1, 1, 1, 1, 2, 2, 2, 2, 2, 2, 2, 1, 1, 1, 1, 1, 2, 2, 2, 2, 2, 2, 2, 1, 1, 1, 1, 1, 1, 2, 2, 2, 2, 2, 1, 1, 1, 1, 1, 1, 2, 2, 2, 2, 1, 1, 1, 1, 1, 1, 2, 2, 2, 1, 1, 1, 1, 1, 2, 2, 2, 2, 2, 1, 1, 1, 1, 2, 2, 1, 1, 2, 4 ),
 ( 0.000000000000000000, 0.06250000000015401569, 0.1250000000003080314, 0.1875000000004620471, 0.2187500000005390688, 0.2343750000005775658, 0.2421875000005963841, 0.2460937500006055434, 0.2480468750006098733, 0.2490234375006122602, 0.2495117187506134815, 0.2497558593756140644, 0.2500000000006146750, 0.3125000000006831757, 0.3750000000007517320, 0.4375000000008202328, 0.4687500000008548717, 0.4843750000008721912, 0.4921875000008812950, 0.4960937500008858470, 0.4980468750008876788, 0.4990234375008891221, 0.4995117187508901768, 0.4997558593758907319, 0.5000000000008912870, 0.5625000000010081935, 0.6250000000011251000, 0.6875000000012428947, 0.7187500000013026247, 0.7343750000013316015, 0.7421875000013461454, 0.7460937500013532508, 0.7480468750013579138, 0.7490234375013611334, 0.7495117187513627988, 0.7497558593763636869, 0.7498779296888640200, 0.7500000000013644641, 0.8125000000014666046, 0.8437500000015185631, 0.8593750000015447643, 0.8671875000015588641, 0.8710937500015667467, 0.8730468750015695223, 0.8740234375015699664, 0.8745117187515702994, 0.8747558593765693002, 0.8748779296890687451, 0.8750000000015680790, 0.9062500000013085089, 0.9218750000011778356, 0.9296875000011124435, 0.9335937500010798029, 0.9355468750010625945, 0.9365234375010541568, 0.9370117187510489387, 0.9372558593760461632, 0.9373779296885438317, 0.9375000000010415002, 0.9531250000007589485, 0.9609375000006168399, 0.9648437500005457856, 0.9667968750005112577, 0.9677734375004941603, 0.9682617187504866108, 0.9685058593754828360, 0.9687500000004790612, 0.9765625000003641532, 0.9804687500003066436, 0.9814453125002918776, 0.9824218750002771117, 0.9843750000002472467, 0.9882812500001895151, 0.9885253906251861844, 0.9886474609376846301, 0.9887695312501830758, 0.9892578125001750822, 0.9902343750001582068, 0.9921875000001258993, 1.000000000000000000 ),
 .UNSPECIFIED. ) ;
#81694=CARTESIAN_POINT ( 'NONE',  ( -8.578981978779999906, 1385.024532827439998, 218.6678019865190095 ) ) ;
#81708=VERTEX_POINT ( 'NONE', #7196 ) ;
#81714=CARTESIAN_POINT ( 'NONE',  ( -16.32897964160000370, 1384.525298249519892, 200.5993092285889929 ) ) ;
#81756=CARTESIAN_POINT ( 'NONE',  ( -97.79264536580190281, 1384.951517786579871, 310.5502822603710342 ) ) ;
#81757=CARTESIAN_POINT ( 'NONE',  ( -8.049886528540000086, 1385.314864400589840, 199.5718903080289977 ) ) ;
#81804=CARTESIAN_POINT ( 'NONE',  ( -12.29457997419999948, 1378.306942845010099, 210.0158913818380029 ) ) ;
#81805=CARTESIAN_POINT ( 'NONE',  ( -104.5732689346720008, 1384.592179270920042, 311.1645418064740056 ) ) ;
#81806=CARTESIAN_POINT ( 'NONE',  ( -62.90092488694899941, 1385.075852493079992, 250.3550165034500026 ) ) ;
#81817=CARTESIAN_POINT ( 'NONE',  ( -109.6501487310000016, 1384.584076603700169, 311.3100189002590241 ) ) ;
#81837=CARTESIAN_POINT ( 'NONE',  ( -67.79781760454831385, 1379.745846262460191, 279.2210569798610322 ) ) ;
#81871=CARTESIAN_POINT ( 'NONE',  ( -67.16270863874164831, 1379.744581544945504, 276.7363381173806829 ) ) ;
#81875=CARTESIAN_POINT ( 'NONE',  ( -68.09224033998870595, 1384.725039953799978, 261.8692284254199762 ) ) ;
#81894=EDGE_CURVE ( 'NONE', #46650, #108404, #73666, .T. ) ;
#81904=CARTESIAN_POINT ( 'NONE',  ( -106.7715504409999880, 1386.777196091089991, 297.2705617508589739 ) ) ;
#81906=CARTESIAN_POINT ( 'NONE',  ( -7.966035888499998663, 1384.903651512129727, 199.4892911144889922 ) ) ;
#81910=CARTESIAN_POINT ( 'NONE',  ( -109.6086345746109885, 1383.178240054900016, 311.2147542219479988 ) ) ;
#81920=CIRCLE ( 'NONE', #96238, 2.000010725851112170 ) ;
#81923=AXIS2_PLACEMENT_3D ( 'NONE', #94731, #59496, #84120 ) ;
#81933=CARTESIAN_POINT ( 'NONE',  ( 7.499999999999998224, 1374.913060387289988, 209.1218459572589836 ) ) ;
#81941=CARTESIAN_POINT ( 'NONE',  ( -109.9698195215979979, 1384.452562162210143, 311.4357956501490321 ) ) ;
#81943=CARTESIAN_POINT ( 'NONE',  ( -29.04272165705700459, 1384.831948739079962, 227.0851056154090202 ) ) ;
#81965=CARTESIAN_POINT ( 'NONE',  ( -67.87968102602539489, 1379.746884770850102, 281.0430582061820246 ) ) ;
#81976=CARTESIAN_POINT ( 'NONE',  ( -7.647431551520000426, 1383.749817281759988, 218.9711582107190111 ) ) ;
#81994=CARTESIAN_POINT ( 'NONE',  ( -109.9496004110956449, 1385.529525279795052, 311.4216302621462660 ) ) ;
#82002=CARTESIAN_POINT ( 'NONE',  ( -37.47102956639999860, 1376.102040661649880, 218.9879198341890003 ) ) ;
#82014=VERTEX_POINT ( 'NONE', #46342 ) ;
#82017=CARTESIAN_POINT ( 'NONE',  ( -89.68054741670000851, 1384.049504871620229, 308.6620857943589726 ) ) ;
#82022=CARTESIAN_POINT ( 'NONE',  ( -62.19530719199999425, 1379.731596365480073, 266.2974022992590335 ) ) ;
#82030=CARTESIAN_POINT ( 'NONE',  ( -106.4194572870000002, 1384.702728600540013, 311.3224507522589306 ) ) ;
#82031=CARTESIAN_POINT ( 'NONE',  ( -32.24223533869999869, 1386.864980676749838, 229.8438144294590018 ) ) ;
#82033=CARTESIAN_POINT ( 'NONE',  ( -54.44628037483680316, 1385.095773140109941, 270.7265002573269612 ) ) ;
#82059=CARTESIAN_POINT ( 'NONE',  ( -105.9703572220000041, 1389.071254289390254, 299.6216621737590344 ) ) ;
#82065=CARTESIAN_POINT ( 'NONE',  ( -105.5164974550000068, 1378.552361626299898, 303.6894019292590201 ) ) ;
#82078=CARTESIAN_POINT ( 'NONE',  ( -105.8349242470570033, 1383.760197502439951, 311.0348730228309932 ) ) ;
#82086=CARTESIAN_POINT ( 'NONE',  ( -89.71137825399999599, 1383.770488589559818, 308.5740051020589476 ) ) ;
#82090=ORIENTED_EDGE ( 'NONE', *, *, #11205, .T. ) ;
#82110=ORIENTED_EDGE ( 'NONE', *, *, #65263, .T. ) ;
#82137=EDGE_LOOP ( 'NONE', ( #99081, #79158 ) ) ;
#82143=CARTESIAN_POINT ( 'NONE',  ( -9.721399282128558639, 1384.510033814309963, 200.0150085476490176 ) ) ;
#82157=CARTESIAN_POINT ( 'NONE',  ( -68.75569806500000425, 1379.747887185579884, 280.1327824861590443 ) ) ;
#82174=CARTESIAN_POINT ( 'NONE',  ( -14.07280436816861169, 1379.603689006211425, 211.7284150537196865 ) ) ;
#82205=CARTESIAN_POINT ( 'NONE',  ( -44.03378961160060356, 1383.821754830599957, 249.2544531064709759 ) ) ;
#82217=CARTESIAN_POINT ( 'NONE',  ( -16.11330378180000267, 1381.436043544759968, 201.9289277945890149 ) ) ;
#82227=CARTESIAN_POINT ( 'NONE',  ( -8.802958355110462207, 1385.645181018859830, 218.6119752371670018 ) ) ;
#82229=DIRECTION ( 'NONE',  ( -0.02344842167732799632, -0.9996113240391217847, 0.01507887176138064667 ) ) ;
#82233=CARTESIAN_POINT ( 'NONE',  ( -104.2256462149999976, 1380.095225975270068, 301.7641063316589793 ) ) ;
#82240=CARTESIAN_POINT ( 'NONE',  ( -68.73088892949999718, 1379.748097453069931, 280.1074355248589995 ) ) ;
#82252=CARTESIAN_POINT ( 'NONE',  ( -109.2617005650000124, 1385.525553972230000, 311.2346411152590235 ) ) ;
#82287=CARTESIAN_POINT ( 'NONE',  ( -25.91586689989999925, 1384.961148014880109, 203.4475886829490037 ) ) ;
#82306=ORIENTED_EDGE ( 'NONE', *, *, #9979, .F. ) ;
#82313=CARTESIAN_POINT ( 'NONE',  ( -109.6853916682353969, 1383.138375255104620, 297.1883635206749545 ) ) ;
#82326=CARTESIAN_POINT ( 'NONE',  ( -79.98142976928239989, 1384.994008373050065, 303.8518676267449905 ) ) ;
#82327=CARTESIAN_POINT ( 'NONE',  ( -8.884967209949998335, 1388.039969697709921, 200.4370767659389969 ) ) ;
#82368=CARTESIAN_POINT ( 'NONE',  ( -105.2215450167301611, 1381.056857365499354, 308.6470483461520189 ) ) ;
#82377=CARTESIAN_POINT ( 'NONE',  ( -66.36738586336869616, 1385.093736160859862, 258.0857209453200198 ) ) ;
#82389=CARTESIAN_POINT ( 'NONE',  ( -109.9698191200000110, 1384.452558329679960, 311.4357953482589778 ) ) ;
#82405=CARTESIAN_POINT ( 'NONE',  ( -5.511153256349429874, 1374.913063729909936, 203.3075733038869828 ) ) ;
#82413=CARTESIAN_POINT ( 'NONE',  ( -68.49931456876349500, 1379.747368005260114, 280.0909653425130159 ) ) ;
#82423=CARTESIAN_POINT ( 'NONE',  ( -106.4040135799809974, 1378.913060387319774, 306.2480672476809787 ) ) ;
#82444=CARTESIAN_POINT ( 'NONE',  ( -68.46546297202630171, 1384.727450216739953, 262.6729272380309794 ) ) ;
#82453=ORIENTED_EDGE ( 'NONE', *, *, #4984, .T. ) ;
#82456=LINE ( 'NONE', #39895, #104662 ) ;
#82475=ORIENTED_EDGE ( 'NONE', *, *, #26821, .F. ) ;
#82476=FACE_OUTER_BOUND ( 'NONE', #103458, .T. ) ;
#82482=CARTESIAN_POINT ( 'NONE',  ( -109.2286396907909989, 1384.893028202680171, 295.1336651452069759 ) ) ;
#82514=CARTESIAN_POINT ( 'NONE',  ( -50.29015339553740205, 1384.738658365939955, 262.3372466638650167 ) ) ;
#82515=CARTESIAN_POINT ( 'NONE',  ( -106.5621319268489913, 1391.913060387289988, 302.9116844650990288 ) ) ;
#82519=CARTESIAN_POINT ( 'NONE',  ( -105.1828009239999915, 1379.114047142900063, 303.4308355331590406 ) ) ;
#82531=CARTESIAN_POINT ( 'NONE',  ( -12.20553011617109895, 1378.355942198320008, 210.8952815345800218 ) ) ;
#82541=CARTESIAN_POINT ( 'NONE',  ( 7.644361507415789768E-14, 1380.413087040579967, 210.0680626132329962 ) ) ;
#82572=CARTESIAN_POINT ( 'NONE',  ( -109.9089029649868081, 1385.746877553887089, 311.3956508573958786 ) ) ;
#82574=CARTESIAN_POINT ( 'NONE',  ( -12.34620125349839803, 1378.802061108420048, 209.1451513645090188 ) ) ;
#82579=CARTESIAN_POINT ( 'NONE',  ( -43.21650806019999891, 1379.188238639419978, 226.3493147681589903 ) ) ;
#82590=CARTESIAN_POINT ( 'NONE',  ( -62.13634214319999671, 1384.087241931920062, 284.7267046562590167 ) ) ;
#82603=CARTESIAN_POINT ( 'NONE',  ( -37.56150324949999941, 1389.587769209160115, 214.8459643147290024 ) ) ;
#82605=CARTESIAN_POINT ( 'NONE',  ( -51.77010361138839301, 1385.111386686199921, 265.3579611613769771 ) ) ;
#82626=CIRCLE ( 'NONE', #43318, 11.34254167809999991 ) ;
#82632=CARTESIAN_POINT ( 'NONE',  ( -103.8748163430000062, 1389.962982481139989, 303.0082707663589758 ) ) ;
#82635=CARTESIAN_POINT ( 'NONE',  ( -105.6555295450000074, 1391.469163183259980, 302.6449347093590063 ) ) ;
#82638=CARTESIAN_POINT ( 'NONE',  ( -105.5440549909999959, 1378.571989651840113, 303.3348456324590074 ) ) ;
#82653=CARTESIAN_POINT ( 'NONE',  ( -113.4000000000000057, 1384.913060387289988, 297.2218459572590064 ) ) ;
#82680=ADVANCED_FACE ( 'NONE', ( #12041 ), #37283, .F. ) ;
#82683=CARTESIAN_POINT ( 'NONE',  ( -8.605915169659999364, 1384.661630203050208, 199.8779420664789939 ) ) ;
#82704=CARTESIAN_POINT ( 'NONE',  ( -23.30935844142160107, 1384.540784663000068, 202.6730237965640242 ) ) ;
#82742=CARTESIAN_POINT ( 'NONE',  ( -5.932239102140000497, 1391.913060387289988, 203.1292509007990077 ) ) ;
#82752=CARTESIAN_POINT ( 'NONE',  ( -12.31942453897649870, 1378.266144378809940, 209.5228905148699994 ) ) ;
#82767=CARTESIAN_POINT ( 'NONE',  ( -46.90474178049270648, 1383.817032368400078, 254.9874098474779771 ) ) ;
#82775=CARTESIAN_POINT ( 'NONE',  ( -22.59757997700000232, 1381.457731642620047, 203.6687691534690146 ) ) ;
#82779=CARTESIAN_POINT ( 'NONE',  ( -7.952410203839279212, 1386.346058257690174, 218.7420460867409986 ) ) ;
#82784=CARTESIAN_POINT ( 'NONE',  ( -105.7905112890000083, 1378.790852282349988, 301.9387464688589944 ) ) ;
#82787=B_SPLINE_CURVE_WITH_KNOTS ( 'NONE', 5,
 ( #16913, #102039, #67382, #93097, #7992, #25326, #42713, #76867, #34300 ),
 .UNSPECIFIED., .F., .F.,
 ( 6, 3, 6 ),
 ( 0.000000000000000000, 0.5465110906119712286, 1.000000000000000000 ),
 .UNSPECIFIED. ) ;
#82789=CARTESIAN_POINT ( 'NONE',  ( -108.0420188247079949, 1385.240018349089951, 297.1067560861690708 ) ) ;
#82800=CARTESIAN_POINT ( 'NONE',  ( -108.8468125590000000, 1386.218237515659894, 311.0462259532590110 ) ) ;
#82805=DIRECTION ( 'NONE',  ( -1.836970198721029688E-16, -1.000000000000000000, 0.000000000000000000 ) ) ;
#82812=VERTEX_POINT ( 'NONE', #80357 ) ;
#82822=ORIENTED_EDGE ( 'NONE', *, *, #72103, .T. ) ;
#82829=CARTESIAN_POINT ( 'NONE',  ( -37.21348786970000333, 1384.710338601940066, 210.1738723234790029 ) ) ;
#82837=EDGE_CURVE ( 'NONE', #76524, #46346, #49835, .T. ) ;
#82861=CARTESIAN_POINT ( 'NONE',  ( -106.0073915721780082, 1391.832578719599951, 305.5439016709390216 ) ) ;
#82868=CARTESIAN_POINT ( 'NONE',  ( -84.84319801522730131, 1384.981735787840080, 306.6237177180889830 ) ) ;
#82869=CARTESIAN_POINT ( 'NONE',  ( -8.875238279790000462, 1385.500419937470042, 199.9517188858189911 ) ) ;
#82898=CARTESIAN_POINT ( 'NONE',  ( 8.432239102140002274, 1391.413060387289988, 209.1218459572589836 ) ) ;
#82910=CARTESIAN_POINT ( 'NONE',  ( -103.6795216995605244, 1379.963998356777893, 305.2549191247096587 ) ) ;
#82915=CARTESIAN_POINT ( 'NONE',  ( -13.51802790139999999, 1379.878742302120145, 211.2357070591689876 ) ) ;
#82917=CARTESIAN_POINT ( 'NONE',  ( -56.07992718850910308, 1385.043137000280012, 235.9174924357720045 ) ) ;
#82928=CARTESIAN_POINT ( 'NONE',  ( -7.544733521240000407, 1384.899971913130003, 219.0877090842990071 ) ) ;
#82929=CARTESIAN_POINT ( 'NONE',  ( -109.3101328239999930, 1384.844761704930079, 311.2642414982589685 ) ) ;
#82946=CARTESIAN_POINT ( 'NONE',  ( -109.1321487942470014, 1384.869787291219836, 311.2644937792119322 ) ) ;
#82948=CARTESIAN_POINT ( 'NONE',  ( -68.49543879489779385, 1379.747280870290069, 280.0944112600439553 ) ) ;
#82950=VERTEX_POINT ( 'NONE', #58877 ) ;
#82951=CARTESIAN_POINT ( 'NONE',  ( -9.403799494689495830, 1380.327828722814047, 217.1736609539314031 ) ) ;
#82987=CARTESIAN_POINT ( 'NONE',  ( -76.82492145107710257, 1384.777666236809864, 278.4853710401239937 ) ) ;
#82998=DIRECTION ( 'NONE',  ( 0.4198226673190290081, -7.712017286126290910E-17, 0.9076061524720597795 ) ) ;
#83025=CARTESIAN_POINT ( 'NONE',  ( -57.85314987360000316, 1379.895658628149931, 259.2190729278590311 ) ) ;
#83040=CARTESIAN_POINT ( 'NONE',  ( -9.929617209772274578, 1390.129315142706446, 216.4882401067509932 ) ) ;
#83043=CARTESIAN_POINT ( 'NONE',  ( -1.836970198721029983E-15, 1374.913060387289988, 209.1218459572589836 ) ) ;
#83057=CARTESIAN_POINT ( 'NONE',  ( -44.13200274799689993, 1384.768345979450032, 249.8261944712759828 ) ) ;
#83085=CARTESIAN_POINT ( 'NONE',  ( -33.87536109878649881, 1377.779994812849964, 222.3620478696320220 ) ) ;
#83087=CARTESIAN_POINT ( 'NONE',  ( -48.20259525819999880, 1379.738770688249815, 241.4393370626590070 ) ) ;
#83109=VERTEX_POINT ( 'NONE', #71725 ) ;
#83118=CARTESIAN_POINT ( 'NONE',  ( -12.60784501594030083, 1379.596188776910139, 209.4492041108660203 ) ) ;
#83121=CARTESIAN_POINT ( 'NONE',  ( -37.01195473260000313, 1379.865299478330144, 219.4187096254589733 ) ) ;
#83135=CARTESIAN_POINT ( 'NONE',  ( -81.19483833489999824, 1384.346490510059994, 304.9342802076590146 ) ) ;
#83150=CARTESIAN_POINT ( 'NONE',  ( -78.59200839480000411, 1388.281368029709938, 283.6153604521589386 ) ) ;
#83153=CARTESIAN_POINT ( 'NONE',  ( -41.37939134543219666, 1385.174059347740013, 244.5779111204580261 ) ) ;
#83180=CARTESIAN_POINT ( 'NONE',  ( -108.8860473499999983, 1387.891312791299924, 297.6832540484590481 ) ) ;
#83182=CARTESIAN_POINT ( 'NONE',  ( -105.5443734370000044, 1391.490361483879951, 303.4240186844589857 ) ) ;
#83230=CARTESIAN_POINT ( 'NONE',  ( -8.369061852370000665, 1384.792577061449947, 199.7768212591290080 ) ) ;
#83235=EDGE_LOOP ( 'NONE', ( #109969, #70428, #23719, #85456, #83414 ) ) ;
#83251=CARTESIAN_POINT ( 'NONE',  ( -45.99657213052490334, 1384.603192663479831, 219.5987073974170016 ) ) ;
#83301=CARTESIAN_POINT ( 'NONE',  ( -109.1588850255340049, 1385.157736184130044, 297.1405484719870174 ) ) ;
#83303=CARTESIAN_POINT ( 'NONE',  ( -109.3504185190000015, 1384.949684454260023, 297.1387114502589952 ) ) ;
#83312=CARTESIAN_POINT ( 'NONE',  ( -13.15550074822679960, 1379.513481804130151, 208.2695128736829986 ) ) ;
#83315=CARTESIAN_POINT ( 'NONE',  ( -53.29909992077880077, 1383.806574426890165, 268.0697932026679950 ) ) ;
#83324=CARTESIAN_POINT ( 'NONE',  ( -66.17857789960000048, 1380.533260727070001, 264.6360122460590105 ) ) ;
#83333=CARTESIAN_POINT ( 'NONE',  ( -106.1566356689999964, 1380.912478904339878, 299.4828590531589612 ) ) ;
#83349=CARTESIAN_POINT ( 'NONE',  ( -109.9182707039999940, 1385.320420619579863, 311.4131465352589885 ) ) ;
#83358=CARTESIAN_POINT ( 'NONE',  ( -14.38571989283190078, 1379.606419413119966, 208.0590348354299692 ) ) ;
#83376=CARTESIAN_POINT ( 'NONE',  ( -84.13302388679998955, 1385.053691251499913, 288.0534502569590245 ) ) ;
#83386=AXIS2_PLACEMENT_3D ( 'NONE', #13904, #31826, #48091 ) ;
#83412=CARTESIAN_POINT ( 'NONE',  ( -11.86940574820000016, 1378.451602169099942, 212.7299449014490165 ) ) ;
#83414=ORIENTED_EDGE ( 'NONE', *, *, #63323, .F. ) ;
#83418=CARTESIAN_POINT ( 'NONE',  ( -8.762939274969999914, 1387.561927349079951, 200.2973833142889930 ) ) ;
#83427=CARTESIAN_POINT ( 'NONE',  ( -109.1387513648781038, 1387.705443260920674, 297.5371259159040278 ) ) ;
#83447=CARTESIAN_POINT ( 'NONE',  ( -109.7181425929999961, 1384.896750758799953, 297.0862127012590008 ) ) ;
#83449=CARTESIAN_POINT ( 'NONE',  ( -5.433843300389891162, 1391.480867605429921, 203.3409103162060205 ) ) ;
#83452=CARTESIAN_POINT ( 'NONE',  ( -104.1632271132076539, 1380.312642488052916, 306.9056418433917770 ) ) ;
#83457=CARTESIAN_POINT ( 'NONE',  ( -12.57230900989999967, 1379.603104922460261, 209.9510306230349954 ) ) ;
#83459=CARTESIAN_POINT ( 'NONE',  ( -55.78789393184250400, 1385.041865729660230, 235.3527397816559983 ) ) ;
#83471=CARTESIAN_POINT ( 'NONE',  ( -109.6605131529999824, 1384.774622188049989, 311.3207091772589479 ) ) ;
#83483=AXIS2_PLACEMENT_3D ( 'NONE', #16587, #41284, #56999 ) ;
#83486=CARTESIAN_POINT ( 'NONE',  ( -109.1334478349630075, 1384.772525000819996, 311.2620895989360292 ) ) ;
#83488=CARTESIAN_POINT ( 'NONE',  ( -68.55293641758220247, 1379.747413382150171, 280.1582828589500309 ) ) ;
#83490=CARTESIAN_POINT ( 'NONE',  ( -8.196710778187490831, 1382.211539317200504, 218.4653390582963368 ) ) ;
#83523=CARTESIAN_POINT ( 'NONE',  ( -10.55745637339999909, 1391.553749436410044, 215.2492821215389824 ) ) ;
#83524=CARTESIAN_POINT ( 'NONE',  ( -82.21554644036051229, 1384.805079599279907, 285.8412598054820251 ) ) ;
#83560=CARTESIAN_POINT ( 'NONE',  ( -109.9467939726550014, 1384.263593440159866, 311.4193346354339837 ) ) ;
#83592=CARTESIAN_POINT ( 'NONE',  ( -47.10372409975749974, 1384.754037987969923, 255.7871177528320175 ) ) ;
#83593=CARTESIAN_POINT ( 'NONE',  ( -107.0320685023289968, 1391.913060387289988, 301.6402820273519865 ) ) ;
#83602=CARTESIAN_POINT ( 'NONE',  ( -8.744618109030934505, 1382.059479685067572, 200.2933607043580366 ) ) ;
#83624=CARTESIAN_POINT ( 'NONE',  ( -25.21612278913649874, 1380.250372108039983, 214.0628279411979804 ) ) ;
#83627=CARTESIAN_POINT ( 'NONE',  ( -29.78513307010349820, 1379.623410526950011, 218.0480817708150028 ) ) ;
#83656=CARTESIAN_POINT ( 'NONE',  ( -108.6472038312455339, 1388.244902418070296, 310.5484619707673346 ) ) ;
#83663=CARTESIAN_POINT ( 'NONE',  ( -11.54050778800000110, 1380.034650811800020, 207.7392432702189922 ) ) ;
#83675=CARTESIAN_POINT ( 'NONE',  ( -87.00440039350000632, 1383.772198133360007, 307.5612418777589596 ) ) ;
#83692=CARTESIAN_POINT ( 'NONE',  ( -72.14102753049999706, 1388.281750947200180, 272.8737667914590475 ) ) ;
#83694=CARTESIAN_POINT ( 'NONE',  ( -45.77496769243909824, 1385.147792078759949, 253.0719673062270090 ) ) ;
#83704=CARTESIAN_POINT ( 'NONE',  ( -8.023175132090001327, 1384.900545175629986, 218.7875346266789904 ) ) ;
#83723=CARTESIAN_POINT ( 'NONE',  ( -108.2398228239999867, 1388.716949575770059, 298.2120931944590438 ) ) ;
#83727=ORIENTED_EDGE ( 'NONE', *, *, #37704, .F. ) ;
#83747=CARTESIAN_POINT ( 'NONE',  ( -14.01398736212220086, 1379.590348564800024, 211.9184487047760115 ) ) ;
#83759=CIRCLE ( 'NONE', #53334, 12.26364123839999998 ) ;
#83779=CARTESIAN_POINT ( 'NONE',  ( -8.371033538129999840, 1384.892342672460245, 199.7750077441390033 ) ) ;
#83798=CARTESIAN_POINT ( 'NONE',  ( -101.8495347479999964, 1379.485289779529921, 303.2301490391590164 ) ) ;
#83801=CARTESIAN_POINT ( 'NONE',  ( -33.28386102025609716, 1384.564240416580105, 207.5449807085249745 ) ) ;
#83813=CARTESIAN_POINT ( 'NONE',  ( -68.78703070794840357, 1379.747968482269926, 280.2966647601920158 ) ) ;
#83815=DIRECTION ( 'NONE',  ( 0.0001174300971986191948, -0.01238049094271260857, -0.9999233518896285533 ) ) ;
#83818=ORIENTED_EDGE ( 'NONE', *, *, #5942, .T. ) ;
#83840=CIRCLE ( 'NONE', #73144, 2.500000000000002220 ) ;
#83855=EDGE_LOOP ( 'NONE', ( #59217, #34995, #103777 ) ) ;
#83864=CARTESIAN_POINT ( 'NONE',  ( -67.25368799669159614, 1383.788001927330015, 291.4842415952459760 ) ) ;
#83872=CARTESIAN_POINT ( 'NONE',  ( -62.11202123059999991, 1379.179948843659986, 266.5711502991589441 ) ) ;
#83875=VERTEX_POINT ( 'NONE', #32832 ) ;
#83883=CARTESIAN_POINT ( 'NONE',  ( -106.8601319760000052, 1381.472917120250031, 298.7909924236589632 ) ) ;
#83903=CARTESIAN_POINT ( 'NONE',  ( -105.5726867909999953, 1391.548264773439996, 305.3922420788589420 ) ) ;
#83917=ORIENTED_EDGE ( 'NONE', *, *, #42847, .F. ) ;
#83935=CARTESIAN_POINT ( 'NONE',  ( -79.49029774420000649, 1385.156174356060092, 282.9512253370589860 ) ) ;
#83945=CARTESIAN_POINT ( 'NONE',  ( -10.25368860849440011, 1391.913060387289988, 204.2726074216130030 ) ) ;
#83965=CARTESIAN_POINT ( 'NONE',  ( -11.75382108840000051, 1380.709723816700034, 215.6909694682190093 ) ) ;
#83970=CARTESIAN_POINT ( 'NONE',  ( -107.0590093890329939, 1384.929322890390040, 311.2486562067720115 ) ) ;
#83972=CARTESIAN_POINT ( 'NONE',  ( -12.61023785360000105, 1389.243603996410002, 203.7013712461890123 ) ) ;
#83985=CARTESIAN_POINT ( 'NONE',  ( -108.2312007977781150, 1388.989242186072715, 298.2560762306327433 ) ) ;
#84010=CARTESIAN_POINT ( 'NONE',  ( -103.7301809698822836, 1380.001629040962371, 305.5444498813670293 ) ) ;
#84018=CARTESIAN_POINT ( 'NONE',  ( -52.55142712537259797, 1385.028519113429866, 229.4265120724080020 ) ) ;
#84029=CARTESIAN_POINT ( 'NONE',  ( -109.6599402350000076, 1384.850943695260185, 311.3226715812589873 ) ) ;
#84046=CARTESIAN_POINT ( 'NONE',  ( -68.50706126879998692, 1379.747743051580073, 280.0840774303590024 ) ) ;
#84069=EDGE_LOOP ( 'NONE', ( #72122, #86595, #27285, #15542, #93819, #87347 ) ) ;
#84080=CARTESIAN_POINT ( 'NONE',  ( -11.05867130699999912, 1391.913060387289988, 212.4652102573489856 ) ) ;
#84081=CARTESIAN_POINT ( 'NONE',  ( -80.64106813425020448, 1384.797475026949996, 283.9371454116219979 ) ) ;
#84096=CARTESIAN_POINT ( 'NONE',  ( -50.69029307030000098, 1379.698255449190128, 241.2869840843590055 ) ) ;
#84120=DIRECTION ( 'NONE',  ( -1.000000000000000000, 1.836970198721029688E-16, 0.000000000000000000 ) ) ;
#84130=CARTESIAN_POINT ( 'NONE',  ( -8.917314821172499961, 1388.823621879021857, 217.7347579895273952 ) ) ;
#84148=CARTESIAN_POINT ( 'NONE',  ( -42.70309239024810211, 1384.775110267059972, 247.0700973881439779 ) ) ;
#84149=CARTESIAN_POINT ( 'NONE',  ( -106.4253901501439969, 1391.913060387279984, 303.6850724643759918 ) ) ;
#84152=CARTESIAN_POINT ( 'NONE',  ( -107.1236086970000088, 1379.003802515750067, 300.1442006366590363 ) ) ;
#84156=CARTESIAN_POINT ( 'NONE',  ( -11.74116011270453441, 1378.248599687866090, 205.3698352297566032 ) ) ;
#84165=CARTESIAN_POINT ( 'NONE',  ( -12.02588869021349893, 1377.660024128230134, 211.7516534935400045 ) ) ;
#84178=CARTESIAN_POINT ( 'NONE',  ( 9.768019850709098135E-14, 1379.967725634990074, 211.0169302589330016 ) ) ;
#84180=CARTESIAN_POINT ( 'NONE',  ( -36.36302950906589615, 1379.637461949829913, 223.8613856847539978 ) ) ;
#84192=AXIS2_PLACEMENT_3D ( 'NONE', #83043, #6336, #64065 ) ;
#84197=( NAMED_UNIT ( * ) SI_UNIT ( $, .STERADIAN. ) SOLID_ANGLE_UNIT ( ) );
#84215=CARTESIAN_POINT ( 'NONE',  ( -18.76550561599999867, 1375.296266888390164, 210.4015402955490117 ) ) ;
#84219=CARTESIAN_POINT ( 'NONE',  ( -105.5765988122880117, 1378.244841141890220, 304.0458102224590107 ) ) ;
#84227=CARTESIAN_POINT ( 'NONE',  ( -113.4000000000000057, 1384.298466609749994, 311.1795487272589753 ) ) ;
#84243=CARTESIAN_POINT ( 'NONE',  ( -50.67894630349999829, 1388.315910739649780, 260.4082215553589776 ) ) ;
#84245=CARTESIAN_POINT ( 'NONE',  ( -50.80630162021439844, 1385.117156927359929, 263.3851759514899982 ) ) ;
#84256=CARTESIAN_POINT ( 'NONE',  ( -8.581120891109998539, 1384.889202694100277, 218.6696492785689827 ) ) ;
#84273=CARTESIAN_POINT ( 'NONE',  ( -109.8137238629999928, 1386.503517745790077, 297.1124110337590309 ) ) ;
#84290=EDGE_CURVE ( 'NONE', #16403, #50191, #71377, .T. ) ;
#84307=CARTESIAN_POINT ( 'NONE',  ( -12.30803116578610101, 1378.373984365000069, 209.8366931216010016 ) ) ;
#84320=DIRECTION ( 'NONE',  ( -1.836970198721029688E-16, -1.000000000000000000, 0.000000000000000000 ) ) ;
#84326=CARTESIAN_POINT ( 'NONE',  ( -8.613169722380000337, 1384.571784085250101, 199.8866694092689897 ) ) ;
#84334=CARTESIAN_POINT ( 'NONE',  ( -12.54019733330000008, 1391.397793261360221, 209.7548870936209937 ) ) ;
#84346=CARTESIAN_POINT ( 'NONE',  ( -109.5441724459999904, 1374.744572155790138, 302.6503169382589817 ) ) ;
#84351=CARTESIAN_POINT ( 'NONE',  ( -41.90775481675180458, 1384.588829037659934, 214.8211095916259978 ) ) ;
#84354=CARTESIAN_POINT ( 'NONE',  ( -109.0826469409999930, 1385.476187853860210, 311.2341188642590168 ) ) ;
#84366=CARTESIAN_POINT ( 'NONE',  ( -68.28255781740000430, 1379.747652651810085, 279.1103140797590072 ) ) ;
#84419=EDGE_CURVE ( 'NONE', #66359, #83109, #66069, .T. ) ;
#84423=CARTESIAN_POINT ( 'NONE',  ( -53.93025590565110150, 1383.805580870739959, 269.3293466918710237 ) ) ;
#84431=CARTESIAN_POINT ( 'NONE',  ( -51.33305125110000233, 1379.090210325960015, 243.4729415681590012 ) ) ;
#84437=CARTESIAN_POINT ( 'NONE',  ( -8.659690377148740126, 1385.678185119990076, 218.6116173138180159 ) ) ;
#84442=CARTESIAN_POINT ( 'NONE',  ( -107.7092647940000063, 1381.097588197639880, 298.6008682247589832 ) ) ;
#84462=CARTESIAN_POINT ( 'NONE',  ( -104.1918408169999992, 1389.706606718110152, 306.6384001822589767 ) ) ;
#84497=CARTESIAN_POINT ( 'NONE',  ( -11.27879581752189964, 1391.913060387259975, 206.8130796129140094 ) ) ;
#84500=ORIENTED_EDGE ( 'NONE', *, *, #11341, .F. ) ;
#84519=CARTESIAN_POINT ( 'NONE',  ( -13.44109269829999853, 1379.757631704399955, 212.9304593775090098 ) ) ;
#84526=CARTESIAN_POINT ( 'NONE',  ( -12.36341556440000033, 1392.311023796360132, 208.2952674222930227 ) ) ;
#84531=CARTESIAN_POINT ( 'NONE',  ( -9.069281542731840062, 1383.978804767730253, 218.5605570552479833 ) ) ;
#84562=CARTESIAN_POINT ( 'NONE',  ( -105.2598989700874199, 1381.083690021850998, 308.6936584762340203 ) ) ;
#84569=CARTESIAN_POINT ( 'NONE',  ( -76.07878363630570107, 1385.141112864619799, 277.2891741808400639 ) ) ;
#84570=CARTESIAN_POINT ( 'NONE',  ( -10.82459666645259944, 1391.913060387289988, 212.9211246486700304 ) ) ;
#84594=CARTESIAN_POINT ( 'NONE',  ( -68.65709740368080816, 1379.747649760600098, 280.2671915801650471 ) ) ;
#84596=CARTESIAN_POINT ( 'NONE',  ( -8.732807974784785543, 1381.269952321672918, 217.9317737700656039 ) ) ;
#84625=CARTESIAN_POINT ( 'NONE',  ( -12.31951492099999967, 1391.575075857879938, 211.0344521122790127 ) ) ;
#84626=CARTESIAN_POINT ( 'NONE',  ( -98.12353807537789407, 1384.868073826160071, 295.8671642013550240 ) ) ;
#84635=EDGE_CURVE ( 'NONE', #47452, #83109, #15657, .T. ) ;
#84644=CARTESIAN_POINT ( 'NONE',  ( -56.68565291850000420, 1379.730069603700031, 254.3216308741590410 ) ) ;
#84676=CARTESIAN_POINT ( 'NONE',  ( -8.071897329778668251, 1387.339191243697087, 218.5828327136565008 ) ) ;
#84677=B_SPLINE_CURVE_WITH_KNOTS ( 'NONE', 3,
 ( #108663, #83449, #6744, #7850, #76717, #76167, #86215, #69450, #85105, #59390, #42018, #8953 ),
 .UNSPECIFIED., .F., .F.,
 ( 4, 2, 2, 2, 2, 4 ),
 ( 0.08322961861458730293, 0.09974321616496879817, 0.1194478573530819987, 0.1410535409231579995, 0.1638632366236909832, 0.1642061257107060024 ),
 .UNSPECIFIED. ) ;
#84695=CARTESIAN_POINT ( 'NONE',  ( -57.27374972444740564, 1384.706877432339979, 276.1255075189790205 ) ) ;
#84696=CARTESIAN_POINT ( 'NONE',  ( -24.13664782116140017, 1384.958061910630022, 202.9396497235290155 ) ) ;
#84703=CARTESIAN_POINT ( 'NONE',  ( -11.50806463233310772, 1378.506956290408880, 204.6827186876646181 ) ) ;
#84724=CARTESIAN_POINT ( 'NONE',  ( -28.23626297441629873, 1380.228258317559948, 215.8353171725599964 ) ) ;
#84727=CARTESIAN_POINT ( 'NONE',  ( -52.24721073780899872, 1379.695346391380099, 249.9998916442930010 ) ) ;
#84733=CARTESIAN_POINT ( 'NONE',  ( -107.4962408000000096, 1378.913060387289988, 308.3050959158589990 ) ) ;
#84734=CARTESIAN_POINT ( 'NONE',  ( -109.1309838779999950, 1384.924111747649931, 311.2646842872590014 ) ) ;
#84760=CARTESIAN_POINT ( 'NONE',  ( -11.59474938729999849, 1379.412984648580050, 207.1178716384889924 ) ) ;
#84772=DIRECTION ( 'NONE',  ( -0.1262450234450830377, -0.9881880602473954722, -0.08687089063570453684 ) ) ;
#84785=CARTESIAN_POINT ( 'NONE',  ( -61.70697236710000055, 1389.529122514739811, 255.3348362324589971 ) ) ;
#84787=CARTESIAN_POINT ( 'NONE',  ( -56.94714792227870248, 1385.081906637989960, 275.5148282826739887 ) ) ;
#84797=CARTESIAN_POINT ( 'NONE',  ( -106.7969504679039972, 1381.490362223440115, 309.5173506577110061 ) ) ;
#84810=CARTESIAN_POINT ( 'NONE',  ( -109.4729007030000076, 1386.928382911489962, 297.3007661288589816 ) ) ;
#84834=ORIENTED_EDGE ( 'NONE', *, *, #42848, .T. ) ;
#84841=CARTESIAN_POINT ( 'NONE',  ( -12.30243638853569976, 1378.355143918360227, 209.9197086792210030 ) ) ;
#84868=CARTESIAN_POINT ( 'NONE',  ( -12.55604107059999919, 1391.387401865550146, 208.6966032511679714 ) ) ;
#84870=B_SPLINE_SURFACE_WITH_KNOTS ( 'NONE', 5, 3, ( 
 ( #62514, #70359, #55757, #97726 ),
 ( #19345, #3149, #55201, #28323 ),
 ( #97174, #12624, #46256, #45146 ),
 ( #46802, #104472, #2597, #20447 ),
 ( #106672, #61957, #79287, #80932 ),
 ( #53545, #29962, #88785, #96636 ),
 ( #12066, #37829, #36722, #19906 ),
 ( #45703, #37281, #72015, #4230 ),
 ( #10412, #38364, #64154, #98273 ),
 ( #44582, #74747, #31618, #14262 ),
 ( #40576, #14815, #56841, #74205 ),
 ( #22636, #92083, #6431, #108885 ),
 ( #31068, #32178, #65249, #47329 ),
 ( #66362, #91537, #64709, #48452 ),
 ( #73651, #56284, #108335, #15357 ),
 ( #90414, #98827, #23763, #38907 ),
 ( #65796, #99360, #41126, #107229 ),
 ( #100481, #90973, #81458, #109449 ),
 ( #101017, #82590, #5881, #40025 ),
 ( #66909, #4763, #22087, #99917 ),
 ( #23212, #32729, #49550, #57412 ),
 ( #13144, #13694, #75306, #24315 ),
 ( #49002, #73089, #83135, #30519 ),
 ( #83675, #57950, #6972, #89875 ),
 ( #47880, #82017, #5322, #39481 ),
 ( #107783, #16991, #103804, #34388 ),
 ( #102126, #59055, #43356, #92625 ),
 ( #24853, #69682, #17554, #51755 ),
 ( #43898, #15900, #75845, #50100 ),
 ( #93176, #102661, #84227, #7527 ) ),
 .UNSPECIFIED., .F., .F., .F.,
 ( 6, 3, 3, 3, 3, 3, 3, 3, 3, 6 ),
 ( 4, 4 ),
 ( 0.000000000000000000, 15.39383910899999997, 27.58084801740000103, 41.39509552349999666, 65.53909258059999843, 90.91108773649999364, 117.6367619669999982, 132.4493970709999928, 144.8160795070000120, 161.8240513320000105 ),
 ( 0.000000000000000000, 2.092690777440000094 ),
 .UNSPECIFIED. ) ;
#84882=CARTESIAN_POINT ( 'NONE',  ( -105.7140364039999980, 1374.461008904089795, 303.4364470169589936 ) ) ;
#84891=CARTESIAN_POINT ( 'NONE',  ( -36.31252284909629680, 1384.572199005869834, 209.7182559141370177 ) ) ;
#84898=CARTESIAN_POINT ( 'NONE',  ( -50.84265507320838395, 1379.695343721229619, 247.3880999093737216 ) ) ;
#84902=CARTESIAN_POINT ( 'NONE',  ( -68.58568551959999127, 1379.747647795449893, 279.7303794029589881 ) ) ;
#84920=CARTESIAN_POINT ( 'NONE',  ( 3.550311703873260096E-15, 1384.899971913130003, 209.1218459572589836 ) ) ;
#84955=CARTESIAN_POINT ( 'NONE',  ( -59.11443824985749984, 1383.797908678129943, 279.0809373516989922 ) ) ;
#84964=CARTESIAN_POINT ( 'NONE',  ( -62.34512127969999540, 1383.170447440649923, 249.3521481918589870 ) ) ;
#84974=CARTESIAN_POINT ( 'NONE',  ( -108.4073513729999974, 1382.402421960810216, 297.8403850943590214 ) ) ;
#84984=VERTEX_POINT ( 'NONE', #2487 ) ;
#84997=CARTESIAN_POINT ( 'NONE',  ( -107.5745933759999957, 1387.689086384770007, 310.1919576522590205 ) ) ;
#85029=ORIENTED_EDGE ( 'NONE', *, *, #70207, .T. ) ;
#85033=CARTESIAN_POINT ( 'NONE',  ( -109.9849726248329915, 1384.916895159399928, 311.4561123681800154 ) ) ;
#85047=ORIENTED_EDGE ( 'NONE', *, *, #59839, .T. ) ;
#85059=CARTESIAN_POINT ( 'NONE',  ( -13.71395948329999825, 1379.587229639339967, 211.8543337660190105 ) ) ;
#85061=ORIENTED_EDGE ( 'NONE', *, *, #20027, .T. ) ;
#85066=AXIS2_PLACEMENT_3D ( 'NONE', #82898, #13467, #47112 ) ;
#85067=CARTESIAN_POINT ( 'NONE',  ( -12.29063212139999983, 1392.314905091580158, 209.7402030487879756 ) ) ;
#85088=CARTESIAN_POINT ( 'NONE',  ( -12.38799748877169904, 1383.860969130600097, 218.8265414708790217 ) ) ;
#85103=CARTESIAN_POINT ( 'NONE',  ( -109.3502800569999920, 1384.878668106390023, 297.1387558422589450 ) ) ;
#85105=CARTESIAN_POINT ( 'NONE',  ( -5.858855997865759946, 1391.912605642699873, 203.1598715823440102 ) ) ;
#85114=CARTESIAN_POINT ( 'NONE',  ( -11.07587008949999863, 1391.913060426370066, 205.3995214137289906 ) ) ;
#85115=CARTESIAN_POINT ( 'NONE',  ( -73.07129608938419096, 1385.127337429350064, 271.9867951422679653 ) ) ;
#85116=CARTESIAN_POINT ( 'NONE',  ( -10.28246376656830030, 1391.913060387289988, 213.9844737885490247 ) ) ;
#85128=EDGE_CURVE ( 'NONE', #22898, #8871, #101824, .T. ) ;
#85146=CIRCLE ( 'NONE', #99449, 3.500000000000003109 ) ;
#85157=CARTESIAN_POINT ( 'NONE',  ( -13.44717672499990080, 1379.564256771150212, 208.3953959236740161 ) ) ;
#85162=ORIENTED_EDGE ( 'NONE', *, *, #55850, .F. ) ;
#85171=CARTESIAN_POINT ( 'NONE',  ( -14.18336309970609932, 1380.133888219859955, 210.8530608805870088 ) ) ;
#85179=CARTESIAN_POINT ( 'NONE',  ( -10.33117234729999900, 1391.913060387289988, 214.5016767380689942 ) ) ;
#85180=CARTESIAN_POINT ( 'NONE',  ( -90.34139317962680593, 1384.840033543810023, 292.7666966122710051 ) ) ;
#85196=CARTESIAN_POINT ( 'NONE',  ( -50.59433295680000242, 1379.743302990699931, 241.3342481622590014 ) ) ;
#85239=CARTESIAN_POINT ( 'NONE',  ( -12.12980996005155276, 1377.655037718360973, 211.2214414945090937 ) ) ;
#85244=CARTESIAN_POINT ( 'NONE',  ( -65.34430217836160182, 1384.676577935759951, 289.2243165953830157 ) ) ;
#85245=CARTESIAN_POINT ( 'NONE',  ( -13.05275046466420008, 1384.938348676199894, 200.3351238176559832 ) ) ;
#85247=CARTESIAN_POINT ( 'NONE',  ( -107.5335879240000025, 1378.913060387289988, 300.4967944802589841 ) ) ;
#85251=CARTESIAN_POINT ( 'NONE',  ( -8.374671775625037284, 1382.833066931880694, 199.9155290017601772 ) ) ;
#85260=CARTESIAN_POINT ( 'NONE',  ( -7.540514764990074781, 1385.122439251179685, 219.0844776276921380 ) ) ;
#85262=CARTESIAN_POINT ( 'NONE',  ( -9.123736442209999353, 1384.508619151449921, 199.9712811190890136 ) ) ;
#85273=CARTESIAN_POINT ( 'NONE',  ( -26.01288487611240186, 1379.670732920850014, 215.3165728412730004 ) ) ;
#85307=CARTESIAN_POINT ( 'NONE',  ( -11.64847922969999949, 1377.842188321789990, 206.5023625028690049 ) ) ;
#85332=CARTESIAN_POINT ( 'NONE',  ( -73.21223786119999488, 1390.654864019360048, 287.6042314150589618 ) ) ;
#85334=CARTESIAN_POINT ( 'NONE',  ( -65.00424250889579980, 1385.043326950109986, 288.7494347189460200 ) ) ;
#85346=CARTESIAN_POINT ( 'NONE',  ( -109.1575033200779927, 1383.485187780409888, 311.0614977769220673 ) ) ;
#85386=ORIENTED_EDGE ( 'NONE', *, *, #100031, .T. ) ;
#85393=CARTESIAN_POINT ( 'NONE',  ( -41.40570855549999862, 1380.117442312619914, 227.6002677670589947 ) ) ;
#85398=CARTESIAN_POINT ( 'NONE',  ( -101.5349560225229908, 1377.092447604730069, 306.6887311473950035 ) ) ;
#85410=CARTESIAN_POINT ( 'NONE',  ( -7.983409256419999878, 1384.364947284539767, 199.5220205512890175 ) ) ;
#85417=CARTESIAN_POINT ( 'NONE',  ( -113.4000000000000057, 1384.913060387289988, 304.2218459572590064 ) ) ;
#85427=CIRCLE ( 'NONE', #62218, 1.000000000000000000 ) ;
#85430=CARTESIAN_POINT ( 'NONE',  ( -113.4000000000000057, 1374.413060387289988, 304.2218459572590064 ) ) ;
#85436=CARTESIAN_POINT ( 'NONE',  ( -45.26921098079020567, 1384.600480252990110, 218.6804048096429938 ) ) ;
#85438=CARTESIAN_POINT ( 'NONE',  ( -103.5806803890000083, 1389.940350142260058, 304.1776731731589507 ) ) ;
#85443=CARTESIAN_POINT ( 'NONE',  ( -66.48613725193760615, 1379.743195139351428, 277.3348019686743555 ) ) ;
#85448=CARTESIAN_POINT ( 'NONE',  ( -68.72596496900000318, 1379.747818773470044, 280.0427953276590074 ) ) ;
#85455=CARTESIAN_POINT ( 'NONE',  ( -8.743385264969999682, 1384.893486076239924, 218.5827849380889916 ) ) ;
#85456=ORIENTED_EDGE ( 'NONE', *, *, #70207, .F. ) ;
#85457=CARTESIAN_POINT ( 'NONE',  ( -9.272580261226769593, 1385.313636453000072, 218.6819139582640048 ) ) ;
#85503=CARTESIAN_POINT ( 'NONE',  ( -72.62010951785889290, 1383.782830401899901, 297.5846722543229816 ) ) ;
#85512=CARTESIAN_POINT ( 'NONE',  ( -58.17684086589999737, 1383.136550875339935, 240.1300462906590099 ) ) ;
#85517=CARTESIAN_POINT ( 'NONE',  ( -5.513264357029999729, 1374.913060387289988, 209.1218459572589836 ) ) ;
#85524=CARTESIAN_POINT ( 'NONE',  ( -108.3070719650000058, 1383.318204079829911, 297.4475841893589632 ) ) ;
#85546=CARTESIAN_POINT ( 'NONE',  ( -108.1994964509999875, 1388.325478153710037, 310.2320290272589887 ) ) ;
#85574=ORIENTED_EDGE ( 'NONE', *, *, #81471, .T. ) ;
#85596=FACE_OUTER_BOUND ( 'NONE', #105859, .T. ) ;
#85605=AXIS2_PLACEMENT_3D ( 'NONE', #76239, #40425, #110386 ) ;
#85606=CARTESIAN_POINT ( 'NONE',  ( -13.29669133360000188, 1379.596949712730066, 212.3329758012989714 ) ) ;
#85614=CARTESIAN_POINT ( 'NONE',  ( -11.73166134470000088, 1389.808667801499951, 203.8872188440389834 ) ) ;
#85620=CARTESIAN_POINT ( 'NONE',  ( -8.860022299467271267, 1384.827477254669930, 218.6840310215359864 ) ) ;
#85625=EDGE_CURVE ( 'NONE', #7502, #89045, #98593, .T. ) ;
#85637=CARTESIAN_POINT ( 'NONE',  ( -9.129808743239919977, 1383.863787745319996, 218.5279288296370055 ) ) ;
#85650=CARTESIAN_POINT ( 'NONE',  ( -109.7178215300000090, 1384.906467897089897, 297.0861894953589513 ) ) ;
#85655=CARTESIAN_POINT ( 'NONE',  ( -14.24367202074330052, 1390.369523491529890, 210.8398262857290035 ) ) ;
#85658=ADVANCED_FACE ( 'NONE', ( #8802 ), #48199, .T. ) ;
#85663=CARTESIAN_POINT ( 'NONE',  ( -10.54817843220000029, 1391.913060387289988, 204.8953073741390085 ) ) ;
#85665=CARTESIAN_POINT ( 'NONE',  ( -75.33569739729779258, 1385.137803142289840, 276.0448183544650647 ) ) ;
#85697=EDGE_CURVE ( 'NONE', #69449, #82812, #75011, .T. ) ;
#85709=CARTESIAN_POINT ( 'NONE',  ( -13.00682114438060033, 1379.342060573179879, 208.5822149791590334 ) ) ;
#85722=CARTESIAN_POINT ( 'NONE',  ( -14.21053568732289918, 1380.204026121820107, 210.6677758705890255 ) ) ;
#85730=CARTESIAN_POINT ( 'NONE',  ( -106.3822989043390095, 1384.893588603729995, 297.0069513608490297 ) ) ;
#85750=CARTESIAN_POINT ( 'NONE',  ( -30.49138227950000157, 1379.618898258369882, 214.1838697673789795 ) ) ;
#85757=EDGE_LOOP ( 'NONE', ( #64867, #92957, #106179, #54628 ) ) ;
#85766=CARTESIAN_POINT ( 'NONE',  ( -9.095046486179999334, 1384.897268781169942, 199.9428014140690095 ) ) ;
#85801=CARTESIAN_POINT ( 'NONE',  ( -113.4235965852909089, 1381.413060387289988, 305.2215675190763591 ) ) ;
#85808=CARTESIAN_POINT ( 'NONE',  ( -81.83957670781239813, 1384.634800382709955, 305.0019059595069848 ) ) ;
#85809=CARTESIAN_POINT ( 'NONE',  ( -19.40613836968019967, 1384.949689164209985, 201.5054105275870029 ) ) ;
#85828=CARTESIAN_POINT ( 'NONE',  ( -10.06333680959999910, 1381.959595553830241, 201.2992880703589833 ) ) ;
#85829=DIRECTION ( 'NONE',  ( 1.836970198721029688E-16, 1.000000000000000000, 0.000000000000000000 ) ) ;
#85843=CARTESIAN_POINT ( 'NONE',  ( -66.98815419365290325, 1379.745645132190020, 277.9424776583130097 ) ) ;
#85849=CARTESIAN_POINT ( 'NONE',  ( -107.8262839200000087, 1378.913060387289988, 308.7442743352589787 ) ) ;
#85858=SURFACE_STYLE_USAGE ( .BOTH. , #68531 ) ;
#85874=CARTESIAN_POINT ( 'NONE',  ( -59.11633403356870531, 1379.721728728080507, 259.3841856975482187 ) ) ;
#85875=CARTESIAN_POINT ( 'NONE',  ( -3.771520285720000309, 1375.389610323599982, 209.1218458698340044 ) ) ;
#85880=CARTESIAN_POINT ( 'NONE',  ( -105.3976796612010105, 1378.878460358250095, 305.0048818320939858 ) ) ;
#85883=ORIENTED_EDGE ( 'NONE', *, *, #97392, .F. ) ;
#85888=B_SPLINE_CURVE_WITH_KNOTS ( 'NONE', 3,
 ( #39311, #100315, #107618, #65079, #90809, #26921, #103623, #60545, #53242, #26347, #1739, #95773, #17938, #94106, #95225, #34761, #85157, #76221, #9552, #61643, #35314, #68394, #25790, #85709, #103049, #101948, #94666, #19039, #42070, #8443, #42616, #61110, #59989, #18487, #82, #67837, #25235, #52134, #52684, #43721, #102500, #27458, #7898, #93549, #9004, #43178 ),
 .UNSPECIFIED., .F., .F.,
 ( 4, 3, 3, 3, 3, 3, 3, 3, 3, 3, 3, 3, 3, 3, 3, 4 ),
 ( -2.000000000000000000, -1.899921065871490011, -1.768492324960689865, -1.635042478424219903, -1.500382481119959976, -1.363810208304299998, -1.226238695583030003, -1.087938997751350056, -0.9492313653944000063, -0.8106048422210849758, -0.6725266165283070308, -0.5353410715184310220, -0.3993255339347789867, -0.2646837051581960587, -0.1315499660857459840, 0.000000000000000000 ),
 .UNSPECIFIED. ) ;
#85901=CARTESIAN_POINT ( 'NONE',  ( -94.50571792069999333, 1385.206310935810052, 294.8715553429590273 ) ) ;
#85903=CARTESIAN_POINT ( 'NONE',  ( -58.94950924095840605, 1385.071407265270182, 279.1407438311780425 ) ) ;
#85917=CARTESIAN_POINT ( 'NONE',  ( -107.5108399970000050, 1380.713577291549882, 309.5364694182589460 ) ) ;
#85932=CARTESIAN_POINT ( 'NONE',  ( -109.6086437639999929, 1385.304251137460142, 297.1179079228590467 ) ) ;
#85936=VERTEX_POINT ( 'NONE', #67941 ) ;
#85949=CARTESIAN_POINT ( 'NONE',  ( -14.00956919615309992, 1384.879701807039964, 219.2459905235510007 ) ) ;
#85980=AXIS2_PLACEMENT_3D ( 'NONE', #106359, #82805, #22875 ) ;
#86001=CARTESIAN_POINT ( 'NONE',  ( -105.7397521540000014, 1379.153471392710117, 302.6503159780590408 ) ) ;
#86007=CARTESIAN_POINT ( 'NONE',  ( -25.90756897309999829, 1384.546519395709765, 203.4684288897289832 ) ) ;
#86008=CARTESIAN_POINT ( 'NONE',  ( -64.27641931829590760, 1384.700183869020066, 253.4426907645700453 ) ) ;
#86020=CARTESIAN_POINT ( 'NONE',  ( -68.45122535890000393, 1379.747412755049936, 279.4374878893589766 ) ) ;
#86028=CARTESIAN_POINT ( 'NONE',  ( -49.58513492879999518, 1384.996931083360096, 260.9114759950589928 ) ) ;
#86030=CARTESIAN_POINT ( 'NONE',  ( -16.54629027219139914, 1385.289268194029773, 219.7699943765580031 ) ) ;
#86037=B_SPLINE_CURVE_WITH_KNOTS ( 'NONE', 3,
 ( #100015, #31159, #74299, #89970 ),
 .UNSPECIFIED., .F., .F.,
 ( 4, 4 ),
 ( 0.08090687173989799530, 0.08222331860531204017 ),
 .UNSPECIFIED. ) ;
#86077=CARTESIAN_POINT ( 'NONE',  ( -64.82673933009961331, 1383.790673287549907, 288.1958069606300228 ) ) ;
#86086=CARTESIAN_POINT ( 'NONE',  ( -78.60087703010000837, 1380.062901053669975, 298.2649052036589978 ) ) ;
#86096=CARTESIAN_POINT ( 'NONE',  ( -109.9794884180000167, 1384.897685350450047, 296.9898195259589784 ) ) ;
#86119=CARTESIAN_POINT ( 'NONE',  ( -105.5485668489999966, 1388.544618357170066, 309.1779867852590655 ) ) ;
#86127=CARTESIAN_POINT ( 'NONE',  ( -10.77443953700000101, 1387.520226337789836, 201.1700256806890081 ) ) ;
#86153=( GEOMETRIC_REPRESENTATION_CONTEXT ( 3 ) GLOBAL_UNCERTAINTY_ASSIGNED_CONTEXT ( ( #93887 ) ) GLOBAL_UNIT_ASSIGNED_CONTEXT ( ( #41656, #109963, #84197 ) ) REPRESENTATION_CONTEXT ( 'NONE', 'WORKASPACE' ) );
#86157=CARTESIAN_POINT ( 'NONE',  ( -11.42304708970420002, 1391.913060387289988, 207.3451802848499881 ) ) ;
#86168=CARTESIAN_POINT ( 'NONE',  ( -3.078458355219999998, 1384.919541752539999, 199.6700055799090023 ) ) ;
#86184=CARTESIAN_POINT ( 'NONE',  ( -12.11107905609999946, 1390.909553154740024, 205.6216718233689846 ) ) ;
#86188=CARTESIAN_POINT ( 'NONE',  ( -8.893072318575100610, 1384.473093328959976, 218.6576864550619916 ) ) ;
#86202=CARTESIAN_POINT ( 'NONE',  ( -11.80945589138680063, 1383.861482993130039, 218.7560470375080115 ) ) ;
#86215=CARTESIAN_POINT ( 'NONE',  ( -5.663447254089099658, 1391.839989632750076, 203.2423981696859983 ) ) ;
#86216=CARTESIAN_POINT ( 'NONE',  ( -14.48038155212669942, 1380.012369224539952, 208.7075723164790304 ) ) ;
#86224=CARTESIAN_POINT ( 'NONE',  ( -11.84218506250000047, 1391.913060323489844, 208.2592681188410211 ) ) ;
#86225=CARTESIAN_POINT ( 'NONE',  ( -69.05597640560989703, 1385.107553815650135, 263.9271920575239392 ) ) ;
#86226=CARTESIAN_POINT ( 'NONE',  ( -9.809994025999090539, 1391.913060387289988, 214.8154631801960193 ) ) ;
#86227=CARTESIAN_POINT ( 'NONE',  ( -16.79549422457180796, 1379.712786052571118, 208.6606538604273453 ) ) ;
#86254=ADVANCED_FACE ( 'NONE', ( #104281 ), #8923, .F. ) ;
#86289=CARTESIAN_POINT ( 'NONE',  ( -95.37154346148018647, 1384.858690459429909, 295.0689016550999781 ) ) ;
#86304=CARTESIAN_POINT ( 'NONE',  ( -103.5806803890000083, 1389.940350142260058, 304.1776731731589507 ) ) ;
#86308=CARTESIAN_POINT ( 'NONE',  ( -44.16865037990000076, 1379.703007072680066, 229.5410392623589928 ) ) ;
#86352=ADVANCED_FACE ( 'NONE', ( #30316 ), #75057, .F. ) ;
#86360=CARTESIAN_POINT ( 'NONE',  ( -67.08513696692429562, 1384.671056508349920, 291.5503426151730650 ) ) ;
#86379=CARTESIAN_POINT ( 'NONE',  ( -8.219561042539998752, 1383.199823560049936, 199.7615019773890026 ) ) ;
#86392=CARTESIAN_POINT ( 'NONE',  ( -66.40710909386241667, 1379.744920543010039, 277.0421639454029901 ) ) ;
#86417=EDGE_LOOP ( 'NONE', ( #54441, #6676, #36294, #18956 ) ) ;
#86426=CARTESIAN_POINT ( 'NONE',  ( -29.97702574129686681, 1379.627454049267953, 213.8718541879157442 ) ) ;
#86442=EDGE_CURVE ( 'NONE', #84984, #33852, #21421, .T. ) ;
#86447=ADVANCED_FACE ( 'NONE', ( #21077 ), #89384, .T. ) ;
#86455=CARTESIAN_POINT ( 'NONE',  ( -89.65022158889999560, 1384.970293222339933, 308.7482827413589348 ) ) ;
#86465=CARTESIAN_POINT ( 'NONE',  ( -109.2031378463979934, 1382.831926674700071, 310.9887859676099993 ) ) ;
#86493=CARTESIAN_POINT ( 'NONE',  ( -17.86631035801030265, 1384.868769857020197, 220.1729067581420054 ) ) ;
#86499=B_SPLINE_CURVE_WITH_KNOTS ( 'NONE', 3,
 ( #51829, #9266, #43426, #61903, #36126, #20398, #10357, #29358, #97129, #104423, #71968, #38310, #11477, #54603, #19292, #88185 ),
 .UNSPECIFIED., .F., .F.,
 ( 4, 3, 3, 3, 3, 4 ),
 ( -3.958893044225889835, -3.921419384640000061, -3.778841049641950001, -3.535848525436170231, -3.369511780086619890, -3.112795738848540328 ),
 .UNSPECIFIED. ) ;
#86519=CARTESIAN_POINT ( 'NONE',  ( -105.6049799648840093, 1378.109173369829932, 306.7703173994800068 ) ) ;
#86551=CARTESIAN_POINT ( 'NONE',  ( -78.82321741190000353, 1375.585673336139962, 290.9639565911590466 ) ) ;
#86556=CARTESIAN_POINT ( 'NONE',  ( -85.86261655710001151, 1384.821806127680020, 289.6800030968590249 ) ) ;
#86557=CARTESIAN_POINT ( 'NONE',  ( -56.35913123646120226, 1384.651571263749929, 236.4900000120020138 ) ) ;
#86559=CARTESIAN_POINT ( 'NONE',  ( -106.7877995600000105, 1387.660326901150029, 310.1072176132589675 ) ) ;
#86570=CARTESIAN_POINT ( 'NONE',  ( -68.11985932390000187, 1379.748509173530010, 278.8066904925590279 ) ) ;
#86580=CARTESIAN_POINT ( 'NONE',  ( -19.17386968219999943, 1384.864972699589771, 220.5237385319589976 ) ) ;
#86593=CARTESIAN_POINT ( 'NONE',  ( -8.871221972256710941, 1385.201631638590015, 218.6720694474429934 ) ) ;
#86595=ORIENTED_EDGE ( 'NONE', *, *, #66480, .T. ) ;
#86600=CARTESIAN_POINT ( 'NONE',  ( -121.3977480003905782, 1384.926148861439970, 304.3966123716357401 ) ) ;
#86619=B_SPLINE_SURFACE_WITH_KNOTS ( 'NONE', 5, 5, ( 
 ( #49133, #13282, #14938, #99493, #40159, #64843 ),
 ( #6561, #40712, #32847, #83813, #74342, #58629 ),
 ( #109034, #81596, #67039, #56425, #56982, #74884 ),
 ( #108469, #66500, #47473, #109577, #73785, #4900 ),
 ( #100605, #23887, #15486, #31753, #49684, #41267 ),
 ( #75441, #90555, #13835, #48020, #82157, #31205 ),
 ( #78167, #60282, #102261, #24987, #26655, #50767 ),
 ( #51311, #67588, #34513, #17122, #85448, #102796 ),
 ( #25541, #60854, #101695, #59731, #93851, #26093 ),
 ( #1480, #8746, #92760, #42929, #69807, #68691 ),
 ( #50238, #94402, #33958, #103925, #68153, #939 ),
 ( #17680, #59191, #84902, #93311, #9863, #395 ),
 ( #8194, #77086, #44031, #16571, #42360, #35063 ),
 ( #18247, #51884, #86020, #16038, #9320, #43484 ),
 ( #33392, #103353, #77627, #69244, #35612, #52442 ),
 ( #27224, #84366, #94979, #7655, #41811, #75968 ),
 ( #86570, #110120, #76515, #110665, #72545, #46807 ),
 ( #80937, #72021, #97178, #71479, #63614, #105038 ),
 ( #28328, #45707, #54112, #89333, #106676, #96642 ),
 ( #44587, #54660, #4235, #53551, #61962, #78732 ),
 ( #10978, #29414, #45152, #38369, #63079, #106137 ),
 ( #28883, #97730, #36727, #37287, #61404, #96076 ),
 ( #52994, #95526, #27770, #18798, #20451, #87127 ),
 ( #12630, #21001, #104477, #79845, #88240, #62520 ),
 ( #88789, #19351, #10417, #87698, #12070, #79292 ),
 ( #2602, #55205, #105600, #70922, #19911, #11532 ),
 ( #70363, #2047, #46262, #36180, #3154, #80391 ),
 ( #3705, #37835, #22091, #89879, #47334, #7397 ),
 ( #33140, #24718, #21551, #109863, #42110, #29966 ),
 ( #56290, #98832, #30524, #16863, #65254, #64159 ),
 ( #8483, #41562, #33685, #98277, #67329, #82022 ),
 ( #55763, #24176, #16319, #75717, #73094, #90418 ),
 ( #59476, #49960, #50520, #13698, #31073, #93586 ),
 ( #107233, #84644, #7941, #67880, #101426, #58915 ),
 ( #93046, #5326, #58364, #81462, #76257, #110406 ),
 ( #51066, #101989, #99366, #42657, #76811, #25275 ),
 ( #85196, #13149, #84096, #4768, #38911, #64715 ),
 ( #47884, #15759, #39486, #73657, #107788, #92490 ),
 ( #61689, #86308, #102535, #2339, #68989, #10717 ),
 ( #103090, #18528, #1781, #36451, #104767, #86859 ),
 ( #17417, #9046, #87986, #77369, #43762, #19646 ),
 ( #44888, #19078, #95811, #52724, #45436, #10151 ),
 ( #11274, #79038, #9591, #70649, #85750, #77914 ),
 ( #44324, #70101, #51615, #25827, #28051, #62241 ),
 ( #43220, #26390, #60028, #78468, #53282, #94146 ),
 ( #670, #103663, #87421, #35918, #34801, #60585 ),
 ( #96367, #104214, #53849, #94705, #1220, #127 ),
 ( #17981, #34250, #68433, #52176, #27501, #35355 ) ),
 .UNSPECIFIED., .F., .F., .F.,
 ( 6, 3, 3, 3, 3, 3, 3, 3, 3, 3, 3, 3, 3, 3, 3, 6 ),
 ( 6, 6 ),
 ( 182.2335547110000107, 182.4224514059999933, 182.6488836039999910, 182.8753158020000171, 183.5360872660000098, 184.5201209679999863, 185.9951582379999877, 188.2072972830000026, 191.5252565730000072, 196.5020170729999904, 209.5656953139999814, 231.9595200839999904, 250.6438719679999849, 278.7167119989999833, 297.4396013979999793, 313.5600086899999610 ),
 ( 0.000000000000000000, 0.5000000000000000000 ),
 .UNSPECIFIED. ) ;
#86624=CARTESIAN_POINT ( 'NONE',  ( -88.09424512964220355, 1383.771532610089935, 307.8360115022359764 ) ) ;
#86631=CARTESIAN_POINT ( 'NONE',  ( -60.95159128010000416, 1380.984161914990182, 278.9881612236590058 ) ) ;
#86642=CARTESIAN_POINT ( 'NONE',  ( -109.8920056810000005, 1383.809063189439939, 297.0622304906589761 ) ) ;
#86644=DIRECTION ( 'NONE',  ( 0.01243399051534999945, -0.9999091450434870465, -0.005205529585659179545 ) ) ;
#86710=EDGE_CURVE ( 'NONE', #96052, #49801, #86499, .T. ) ;
#86718=CARTESIAN_POINT ( 'NONE',  ( -113.4000000000000057, 1390.939237335599955, 304.2218459572590064 ) ) ;
#86719=CARTESIAN_POINT ( 'NONE',  ( -17.53487789670000296, 1386.947750201170038, 219.7453638570590044 ) ) ;
#86730=CARTESIAN_POINT ( 'NONE',  ( -8.578849961799997814, 1381.727047392470013, 218.1308605599590180 ) ) ;
#86732=AXIS2_PLACEMENT_3D ( 'NONE', #109756, #108092, #41459 ) ;
#86758=CARTESIAN_POINT ( 'NONE',  ( -9.878584958427840235, 1383.863156290969982, 218.5760999266929900 ) ) ;
#86766=CARTESIAN_POINT ( 'NONE',  ( -4.273368017822010083E-16, 1381.377992659140091, 201.0499806489090133 ) ) ;
#86780=CARTESIAN_POINT ( 'NONE',  ( -11.55178806880000053, 1391.830795966499863, 205.9355060421790142 ) ) ;
#86781=CARTESIAN_POINT ( 'NONE',  ( -70.27838710172480319, 1385.113716173099874, 266.4821626989880201 ) ) ;
#86783=CARTESIAN_POINT ( 'NONE',  ( -62.81000518919999109, 1379.749407722699971, 268.0377337381589768 ) ) ;
#86806=CARTESIAN_POINT ( 'NONE',  ( -68.75512860862529863, 1379.747884653289930, 280.3306324661879785 ) ) ;
#86842=CARTESIAN_POINT ( 'NONE',  ( -95.64847269556051401, 1384.859662006189865, 295.1635381067140429 ) ) ;
#86859=CARTESIAN_POINT ( 'NONE',  ( -42.12884346819999593, 1379.660956442229917, 225.9714894042589890 ) ) ;
#86892=CARTESIAN_POINT ( 'NONE',  ( -14.37880041125569974, 1379.596399452129845, 208.0441480758460102 ) ) ;
#86893=TOROIDAL_SURFACE ( 'NONE', #43738, 11.26398391340000060, 1.000000000000000000 ) ;
#86910=DIRECTION ( 'NONE',  ( -1.000000000000000000, 0.000000000000000000, 0.000000000000000000 ) ) ;
#86915=CARTESIAN_POINT ( 'NONE',  ( -68.14837186395048718, 1384.667842634059980, 292.8870578847530055 ) ) ;
#86932=CARTESIAN_POINT ( 'NONE',  ( -8.988624297290000342, 1382.710527411900102, 200.4007720520790201 ) ) ;
#86945=CARTESIAN_POINT ( 'NONE',  ( -62.58397168594589743, 1379.733354689810085, 270.6756891441229982 ) ) ;
#86978=CARTESIAN_POINT ( 'NONE',  ( -47.55859677702834176, 1379.679709275042569, 234.9829726369564469 ) ) ;
#86997=CARTESIAN_POINT ( 'NONE',  ( -2.541451598548929826E-15, 1375.913060387289988, 209.1218459572589836 ) ) ;
#87005=( BOUNDED_CURVE ( )  B_SPLINE_CURVE ( 3, ( #107412, #65443, #56480, #90052 ),
 .UNSPECIFIED., .F., .T. ) 
 B_SPLINE_CURVE_WITH_KNOTS ( ( 4, 4 ),
 ( 1.611169255404983236, 1.690789859815214458 ),
 .UNSPECIFIED. ) 
 CURVE ( )  GEOMETRIC_REPRESENTATION_ITEM ( )  RATIONAL_B_SPLINE_CURVE ( ( 1.000000000000000000, 0.9994717830474746378, 0.9994717830474746378, 1.000000000000000000 ) ) 
 REPRESENTATION_ITEM ( '' )  );
#87007=CARTESIAN_POINT ( 'NONE',  ( -94.13685229450000236, 1388.280613784919979, 295.9239280321589831 ) ) ;
#87013=AXIS2_PLACEMENT_3D ( 'NONE', #7364, #40962, #25243 ) ;
#87018=CARTESIAN_POINT ( 'NONE',  ( -108.4979148419599966, 1382.105573316219989, 310.5376726789369854 ) ) ;
#87049=CARTESIAN_POINT ( 'NONE',  ( -9.246645418283801376, 1384.892010108799923, 218.7062641367850233 ) ) ;
#87107=CARTESIAN_POINT ( 'NONE',  ( -88.16707050029999948, 1379.270434038089888, 298.5681932088589861 ) ) ;
#87108=ADVANCED_FACE ( 'NONE', ( #3328 ), #92932, .F. ) ;
#87113=CARTESIAN_POINT ( 'NONE',  ( -109.9987473180000137, 1385.244513981200043, 297.1847073398589600 ) ) ;
#87114=CARTESIAN_POINT ( 'NONE',  ( -58.24002330138049643, 1384.662383407990092, 240.2918130150210061 ) ) ;
#87127=CARTESIAN_POINT ( 'NONE',  ( -66.98943634389999602, 1379.744194872529988, 276.3872057256589869 ) ) ;
#87136=CARTESIAN_POINT ( 'NONE',  ( -32.09787761819999474, 1385.089932967300001, 229.9554828700589724 ) ) ;
#87138=CARTESIAN_POINT ( 'NONE',  ( -18.21948982384089888, 1385.283089966090074, 220.2654309255580074 ) ) ;
#87151=CARTESIAN_POINT ( 'NONE',  ( -5.519031869190039963, 1391.701565166340060, 214.9395334166419786 ) ) ;
#87186=CARTESIAN_POINT ( 'NONE',  ( -90.09176604164480295, 1383.770261446130007, 308.5472844327179587 ) ) ;
#87187=CARTESIAN_POINT ( 'NONE',  ( 1.106990746626510029E-15, 1390.939237335599955, 209.1218459572589836 ) ) ;
#87193=CARTESIAN_POINT ( 'NONE',  ( -81.52042378539999845, 1379.302443467629928, 294.8143971615589862 ) ) ;
#87204=CARTESIAN_POINT ( 'NONE',  ( -109.3876690420000131, 1382.506854422480046, 297.3616832378589834 ) ) ;
#87265=CARTESIAN_POINT ( 'NONE',  ( -11.67377857781220030, 1391.913060387289988, 209.5093625368419907 ) ) ;
#87277=CARTESIAN_POINT ( 'NONE',  ( -31.75214877180000528, 1390.937306157359899, 216.9912452226689936 ) ) ;
#87302=CARTESIAN_POINT ( 'NONE',  ( -12.31857035642650011, 1378.312663573310147, 209.5823498162050100 ) ) ;
#87303=ADVANCED_FACE ( 'NONE', ( #73701 ), #8006, .F. ) ;
#87317=CARTESIAN_POINT ( 'NONE',  ( -34.02204320874939469, 1383.836828112509920, 232.5604475453570217 ) ) ;
#87325=DIRECTION ( 'NONE',  ( 0.02615379780595215864, -0.9996573249755578150, -0.001100673901560477895 ) ) ;
#87326=CARTESIAN_POINT ( 'NONE',  ( -9.376059709543110700E-16, 1379.808971210409936, 214.0914956899389949 ) ) ;
#87332=CARTESIAN_POINT ( 'NONE',  ( -14.34064265566260055, 1380.320133270729912, 209.7503807163919873 ) ) ;
#87339=CARTESIAN_POINT ( 'NONE',  ( -11.89096413900000115, 1391.913060356950155, 208.7476111290540075 ) ) ;
#87340=CARTESIAN_POINT ( 'NONE',  ( -98.26796998229559676, 1385.216402604680070, 295.9131571092459581 ) ) ;
#87343=CARTESIAN_POINT ( 'NONE',  ( -63.89205165820000332, 1379.749420737849960, 270.3321189449590065 ) ) ;
#87347=ORIENTED_EDGE ( 'NONE', *, *, #104128, .F. ) ;
#87369=AXIS2_PLACEMENT_3D ( 'NONE', #92315, #58187, #23991 ) ;
#87403=CARTESIAN_POINT ( 'NONE',  ( -11.87928044310000075, 1391.913060387289988, 209.7224407804460213 ) ) ;
#87411=ORIENTED_EDGE ( 'NONE', *, *, #20788, .F. ) ;
#87421=CARTESIAN_POINT ( 'NONE',  ( -18.83042350510000063, 1379.621298762690003, 208.9674219452180068 ) ) ;
#87485=CARTESIAN_POINT ( 'NONE',  ( -66.72900126439060386, 1384.672153193259874, 291.0917829019970213 ) ) ;
#87486=CARTESIAN_POINT ( 'NONE',  ( -29.54457669783570140, 1384.967922959629959, 205.3221292075180031 ) ) ;
#87491=CARTESIAN_POINT ( 'NONE',  ( -5.292751683389999684, 1386.092796132480089, 214.8417591471989851 ) ) ;
#87492=CARTESIAN_POINT ( 'NONE',  ( -8.848268338060000460, 1384.931973698940055, 199.9247712804389892 ) ) ;
#87502=CARTESIAN_POINT ( 'NONE',  ( -12.89895815099780130, 1379.435140844680063, 211.3213831571520132 ) ) ;
#87506=B_SPLINE_CURVE_WITH_KNOTS ( 'NONE', 3,
 ( #62318, #80743, #2961, #63423, #89137, #4052, #19146, #53353, #44958, #11886, #53923, #104839, #78538, #28688, #1852, #105394, #88604, #35987, #79106, #11343, #80191, #54466, #37078, #46058, #37633, #38178, #71838, #103733, #27032, #71281, #28126, #70175, #104286, #61221 ),
 .UNSPECIFIED., .F., .F.,
 ( 4, 3, 3, 3, 3, 3, 3, 3, 3, 3, 3, 4 ),
 ( 4.497076618296339975E-07, 0.8097585624606019605, 1.639511105808459934, 2.030720938957220056, 2.898872277768610228, 3.784635505398759925, 4.221522473682940202, 4.606556899451190290, 5.525126413775890200, 6.438844840059180008, 6.927804315340000407, 7.850516048179999373 ),
 .UNSPECIFIED. ) ;
#87515=CARTESIAN_POINT ( 'NONE',  ( -62.61021140161710008, 1379.731611446759871, 270.6613306315579734 ) ) ;
#87545=CARTESIAN_POINT ( 'NONE',  ( -7.769368482660000019, 1384.919440823630111, 218.9178397582889772 ) ) ;
#87548=FACE_OUTER_BOUND ( 'NONE', #27428, .T. ) ;
#87549=CARTESIAN_POINT ( 'NONE',  ( -57.39613275940437376, 1379.715796048977836, 255.4829930585067927 ) ) ;
#87561=CARTESIAN_POINT ( 'NONE',  ( -57.32900025239892727, 1379.717698082794413, 260.4930733565817604 ) ) ;
#87570=DIRECTION ( 'NONE',  ( 0.9076061524720596685, 1.962993793439040551E-32, -0.4198226673190293412 ) ) ;
#87580=CARTESIAN_POINT ( 'NONE',  ( -92.73157688390000430, 1386.757379292640053, 294.2674297909590564 ) ) ;
#87593=CARTESIAN_POINT ( 'NONE',  ( -104.9983700835409905, 1380.418911759009916, 307.4638771597370237 ) ) ;
#87605=DIRECTION ( 'NONE',  ( -0.9076355166982633671, -0.02210890796429692759, -0.4191765320440813958 ) ) ;
#87618=CARTESIAN_POINT ( 'NONE',  ( -10.97681301304650070, 1384.887672684300014, 218.8427800890989943 ) ) ;
#87671=ORIENTED_EDGE ( 'NONE', *, *, #74750, .T. ) ;
#87673=CARTESIAN_POINT ( 'NONE',  ( -88.74645359839999514, 1377.077971548199912, 297.4629295155589830 ) ) ;
#87675=EDGE_CURVE ( 'NONE', #26117, #99683, #67675, .T. ) ;
#87698=CARTESIAN_POINT ( 'NONE',  ( -66.40232362439998326, 1379.742130965479873, 275.2934539270590335 ) ) ;
#87699=CARTESIAN_POINT ( 'NONE',  ( -109.9852647598198843, 1384.923065380487742, 311.4561663452018934 ) ) ;
#87706=EDGE_CURVE ( 'NONE', #50191, #76524, #13609, .T. ) ;
#87707=CARTESIAN_POINT ( 'NONE',  ( -54.13050464459999489, 1384.845572836569772, 270.3682627440589954 ) ) ;
#87734=CARTESIAN_POINT ( 'NONE',  ( 0.000000000000000000, 1384.913060387289988, 209.1218459572589836 ) ) ;
#87755=CARTESIAN_POINT ( 'NONE',  ( -95.22212654925510833, 1383.767033602980064, 309.9034185838269764 ) ) ;
#87756=CARTESIAN_POINT ( 'NONE',  ( -109.4402575644460001, 1383.302147128139950, 311.1271210982910134 ) ) ;
#87763=CARTESIAN_POINT ( 'NONE',  ( -82.36118214929999226, 1380.660938380089874, 289.8805188183589507 ) ) ;
#87764=DIRECTION ( 'NONE',  ( -1.836970198721029688E-16, -1.000000000000000000, 0.000000000000000000 ) ) ;
#87768=CARTESIAN_POINT ( 'NONE',  ( -109.3492338110000048, 1384.921838666169833, 297.1385152072589904 ) ) ;
#87847=DIRECTION ( 'NONE',  ( 1.836970198721029688E-16, 1.000000000000000000, 0.000000000000000000 ) ) ;
#87848=CARTESIAN_POINT ( 'NONE',  ( -27.75968971620000048, 1386.892151378640165, 225.4868526693589956 ) ) ;
#87849=CARTESIAN_POINT ( 'NONE',  ( -13.29657497211445794, 1389.765381873174420, 214.2158378427034222 ) ) ;
#87856=CARTESIAN_POINT ( 'NONE',  ( -8.982902946400001198, 1383.064277652569899, 218.2826811425790083 ) ) ;
#87885=CARTESIAN_POINT ( 'NONE',  ( -26.54368091973730159, 1383.846278271480060, 224.6430921072530111 ) ) ;
#87893=CARTESIAN_POINT ( 'NONE',  ( -9.835690489261324387, 1389.390132783129729, 201.5977833131792920 ) ) ;
#87909=CARTESIAN_POINT ( 'NONE',  ( -100.7263133942470006, 1385.222699183060058, 296.4096551585109864 ) ) ;
#87912=ORIENTED_EDGE ( 'NONE', *, *, #85128, .T. ) ;
#87935=CARTESIAN_POINT ( 'NONE',  ( -109.0547027409999998, 1384.148091023459756, 297.1846209902590203 ) ) ;
#87967=CARTESIAN_POINT ( 'NONE',  ( -12.40508161610000037, 1391.584463596800106, 210.3939176184290147 ) ) ;
#87983=CARTESIAN_POINT ( 'NONE',  ( -109.0712831559999927, 1385.610640481809924, 297.1783689030590381 ) ) ;
#87986=CARTESIAN_POINT ( 'NONE',  ( -37.75146778639999923, 1379.660437608350094, 220.6592702495590004 ) ) ;
#87998=CARTESIAN_POINT ( 'NONE',  ( -58.27342821996139577, 1385.074879826650204, 277.9421718526420477 ) ) ;
#88031=CARTESIAN_POINT ( 'NONE',  ( -7.543275436179440518, 1384.798777593330215, 219.0854894083749969 ) ) ;
#88044=CARTESIAN_POINT ( 'NONE',  ( -109.0035882723349943, 1384.583473043429876, 311.2498069574970714 ) ) ;
#88045=CARTESIAN_POINT ( 'NONE',  ( -47.75334323544549875, 1385.011498351640057, 221.9354493742870034 ) ) ;
#88051=CARTESIAN_POINT ( 'NONE',  ( -7.966031924080000159, 1384.919940016020064, 199.4892488166489670 ) ) ;
#88062=CARTESIAN_POINT ( 'NONE',  ( -12.26635723510000098, 1379.122879128199884, 206.2237812648789941 ) ) ;
#88074=CARTESIAN_POINT ( 'NONE',  ( -63.34523448999999573, 1379.747030511940238, 271.7626510974590133 ) ) ;
#88095=ORIENTED_EDGE ( 'NONE', *, *, #88529, .F. ) ;
#88097=ORIENTED_EDGE ( 'NONE', *, *, #15882, .T. ) ;
#88104=CARTESIAN_POINT ( 'NONE',  ( -56.30397432574992678, 1379.711908693320993, 253.0148838135297638 ) ) ;
#88117=CARTESIAN_POINT ( 'NONE',  ( -48.14807380225922628, 1379.685700880162813, 242.2423365738800101 ) ) ;
#88119=CARTESIAN_POINT ( 'NONE',  ( -113.4000000000000057, 1379.013060387289897, 304.2218459572590064 ) ) ;
#88135=CARTESIAN_POINT ( 'NONE',  ( -98.84258614210000360, 1386.766722940489899, 296.3872529111589529 ) ) ;
#88146=CARTESIAN_POINT ( 'NONE',  ( -106.1744482317629945, 1381.515665816750015, 309.3820691888080319 ) ) ;
#88170=CARTESIAN_POINT ( 'NONE',  ( -23.36861497038490043, 1384.851536731240003, 222.6440924076069905 ) ) ;
#88185=CARTESIAN_POINT ( 'NONE',  ( -109.9857364230449974, 1384.899971927750130, 311.4562996732899478 ) ) ;
#88190=CARTESIAN_POINT ( 'NONE',  ( -60.47573540665300129, 1377.428416197120214, 271.2551842102760133 ) ) ;
#88194=ORIENTED_EDGE ( 'NONE', *, *, #98017, .F. ) ;
#88199=CARTESIAN_POINT ( 'NONE',  ( -105.5826496779999957, 1391.887501467710081, 304.2218457088590071 ) ) ;
#88207=CARTESIAN_POINT ( 'NONE',  ( 2.285841285774699520E-15, 1391.426148861440197, 209.1218459572589836 ) ) ;
#88222=CARTESIAN_POINT ( 'NONE',  ( -12.33252012447020185, 1378.517259983480017, 208.8147234695160250 ) ) ;
#88223=CARTESIAN_POINT ( 'NONE',  ( -70.57508978779999609, 1378.817654444100071, 279.4267215249590208 ) ) ;
#88240=CARTESIAN_POINT ( 'NONE',  ( -66.62763224750000290, 1379.742540601970177, 275.7011351548590028 ) ) ;
#88248=CARTESIAN_POINT ( 'NONE',  ( -76.10119759110000359, 1384.646775243249976, 301.2182732922589707 ) ) ;
#88249=ORIENTED_EDGE ( 'NONE', *, *, #72103, .F. ) ;
#88250=CARTESIAN_POINT ( 'NONE',  ( -35.41017701237090165, 1385.207010604219931, 234.7551950391080027 ) ) ;
#88254=DIRECTION ( 'NONE',  ( -0.4198226673190288971, 7.712017286126290910E-17, -0.9076061524720597795 ) ) ;
#88291=CARTESIAN_POINT ( 'NONE',  ( -94.92604110475619450, 1383.767219722170239, 309.8421315003910195 ) ) ;
#88293=CARTESIAN_POINT ( 'NONE',  ( -109.3255347603840022, 1384.025522620290076, 311.1851463503860487 ) ) ;
#88298=CARTESIAN_POINT ( 'NONE',  ( -93.71265355510000461, 1380.723683565119927, 297.1406752587590177 ) ) ;
#88310=CARTESIAN_POINT ( 'NONE',  ( -109.1655177890000061, 1384.872414444939977, 297.1329087538589420 ) ) ;
#88380=CARTESIAN_POINT ( 'NONE',  ( -23.00221949109999997, 1384.956020836430071, 202.3857052141389943 ) ) ;
#88381=CARTESIAN_POINT ( 'NONE',  ( -10.42770192888281144, 1387.487768598823777, 217.7251358788310256 ) ) ;
#88388=CARTESIAN_POINT ( 'NONE',  ( -10.37222135890000096, 1380.909514438620135, 216.5949044049989993 ) ) ;
#88401=CARTESIAN_POINT ( 'NONE',  ( -12.31697047491260122, 1378.344771059540108, 209.6432931632009797 ) ) ;
#88418=CARTESIAN_POINT ( 'NONE',  ( -30.94934575091909679, 1383.840876600240108, 228.8241727730240029 ) ) ;
#88428=CARTESIAN_POINT ( 'NONE',  ( -9.420327913192419800, 1388.839158060524824, 201.0591600557601453 ) ) ;
#88435=CARTESIAN_POINT ( 'NONE',  ( -10.42777903026719954, 1387.487736158059988, 217.7251714971619947 ) ) ;
#88445=CARTESIAN_POINT ( 'NONE',  ( -103.8521778202700006, 1385.230324909849969, 296.8200838699809765 ) ) ;
#88454=AXIS2_PLACEMENT_3D ( 'NONE', #54127, #88254, #3170 ) ;
#88491=CARTESIAN_POINT ( 'NONE',  ( -16.33302336319999881, 1384.944327755149970, 200.5749513780490076 ) ) ;
#88528=CARTESIAN_POINT ( 'NONE',  ( -48.20259525661973043, 1379.738770687325086, 241.4393370634903988 ) ) ;
#88529=EDGE_CURVE ( 'NONE', #46346, #16403, #25969, .T. ) ;
#88535=CARTESIAN_POINT ( 'NONE',  ( -60.29112477526700076, 1385.064694404370130, 281.4546780721300365 ) ) ;
#88545=CARTESIAN_POINT ( 'NONE',  ( -12.54019733330000008, 1391.397793261360221, 209.7548870936209937 ) ) ;
#88587=CARTESIAN_POINT ( 'NONE',  ( -92.03485832854140369, 1384.615476698869998, 309.3200307111670213 ) ) ;
#88588=CARTESIAN_POINT ( 'NONE',  ( -49.41110956018160749, 1385.017027258259986, 224.3527585868430094 ) ) ;
#88604=CARTESIAN_POINT ( 'NONE',  ( -106.6417041771089913, 1391.913060387289988, 305.7294994898900313 ) ) ;
#88608=CARTESIAN_POINT ( 'NONE',  ( -12.71390971709999995, 1379.576682373769927, 206.2215170013890031 ) ) ;
#88621=CARTESIAN_POINT ( 'NONE',  ( -67.56980796919920351, 1379.745055568280122, 278.8799826345460815 ) ) ;
#88625=VERTEX_POINT ( 'NONE', #52239 ) ;
#88626=CARTESIAN_POINT ( 'NONE',  ( -105.7942891969999977, 1378.913060387289988, 304.0474106464590136 ) ) ;
#88650=CARTESIAN_POINT ( 'NONE',  ( -7.769002072320000174, 1384.928845199370016, 218.9178307580690159 ) ) ;
#88653=CARTESIAN_POINT ( 'NONE',  ( -68.48903935974368551, 1379.747406510886776, 279.4606711651055662 ) ) ;
#88683=CARTESIAN_POINT ( 'NONE',  ( -113.4000000000000057, 1388.279812043220090, 298.3521000786590207 ) ) ;
#88695=CARTESIAN_POINT ( 'NONE',  ( -105.5885868690189966, 1378.666813780319899, 305.5093639108209800 ) ) ;
#88712=ORIENTED_EDGE ( 'NONE', *, *, #37893, .F. ) ;
#88719=CARTESIAN_POINT ( 'NONE',  ( -34.25392201084810040, 1384.812092138909975, 233.1617710834259753 ) ) ;
#88739=CARTESIAN_POINT ( 'NONE',  ( -55.42473571849600233, 1377.502816453089963, 260.3293090052349612 ) ) ;
#88749=CARTESIAN_POINT ( 'NONE',  ( -8.127570150269997740, 1383.933791805179908, 218.6735113165989901 ) ) ;
#88770=CONICAL_SURFACE ( 'NONE', #103038, 0.9999999999999857891, 0.7853981633970000820 ) ;
#88773=CARTESIAN_POINT ( 'NONE',  ( -94.91986059570000123, 1378.602426990669983, 300.7314404810590531 ) ) ;
#88778=CARTESIAN_POINT ( 'NONE',  ( -98.86863956199999848, 1385.102662047930153, 296.2487962393589669 ) ) ;
#88785=CARTESIAN_POINT ( 'NONE',  ( -17.46864620450000061, 1384.529923560180123, 219.9544858071590170 ) ) ;
#88789=CARTESIAN_POINT ( 'NONE',  ( -66.34652574609999931, 1379.749084393009980, 275.3210452576589660 ) ) ;
#88799=CARTESIAN_POINT ( 'NONE',  ( -37.94803686207870186, 1385.193463608850152, 238.6440774005280048 ) ) ;
#88822=FACE_OUTER_BOUND ( 'NONE', #108980, .T. ) ;
#88827=B_SPLINE_CURVE_WITH_KNOTS ( 'NONE', 3,
 ( #105365, #28656, #20236, #88031, #53896, #10762, #96972, #105926, #104259, #11315, #89104, #54438, #61732, #10193, #95855, #20779, #80155, #79079, #1824, #71806, #3476, #29205, #44368, #4021, #27550, #54979, #46578, #71243, #35959, #2385, #11854 ),
 .UNSPECIFIED., .F., .F.,
 ( 4, 3, 3, 3, 3, 3, 3, 3, 3, 3, 4 ),
 ( -27.07213034079750003, -26.91076046188110027, -26.52795488250579936, -26.13083096461109989, -25.74235510102220204, -25.70743013386550047, -25.40268465535810094, -25.05323574494259731, -24.71773051742599847, -24.43806349879320194, -24.41308947361219950 ),
 .UNSPECIFIED. ) ;
#88829=CARTESIAN_POINT ( 'NONE',  ( -105.5765755770000141, 1378.244848860319962, 304.0471334908590393 ) ) ;
#88842=CARTESIAN_POINT ( 'NONE',  ( -89.68991106499699129, 1383.770515819449884, 308.4149094695740132 ) ) ;
#88844=CARTESIAN_POINT ( 'NONE',  ( -109.2165961150899989, 1384.279859431989962, 311.2110007195050230 ) ) ;
#88854=CARTESIAN_POINT ( 'NONE',  ( -110.0636336660000012, 1384.926148863469962, 296.9511392543589636 ) ) ;
#88924=CARTESIAN_POINT ( 'NONE',  ( -9.117370426725258881, 1384.541028373849940, 199.9667117751619685 ) ) ;
#88928=CARTESIAN_POINT ( 'NONE',  ( -14.07701606803241923, 1379.612174084935305, 211.7004875632037226 ) ) ;
#88945=CARTESIAN_POINT ( 'NONE',  ( -109.3532201929999985, 1385.076312201809969, 297.1413702938589836 ) ) ;
#88957=CARTESIAN_POINT ( 'NONE',  ( -23.95151507931580070, 1383.849269534789983, 222.8015749634270151 ) ) ;
#88966=CARTESIAN_POINT ( 'NONE',  ( -6.053292825790000720, 1379.821371071459907, 214.0283920821290167 ) ) ;
#88973=CARTESIAN_POINT ( 'NONE',  ( -11.11381666019869918, 1389.577331926439911, 215.4847763224689743 ) ) ;
#88982=CARTESIAN_POINT ( 'NONE',  ( -88.76030199668080911, 1385.188808422029979, 291.7738006920690168 ) ) ;
#88984=CARTESIAN_POINT ( 'NONE',  ( -68.57300709150000273, 1379.748249346600005, 279.7358748726589965 ) ) ;
#88988=CARTESIAN_POINT ( 'NONE',  ( -109.1645132478509908, 1384.901512804259937, 297.1326343494729940 ) ) ;
#89045=VERTEX_POINT ( 'NONE', #17342 ) ;
#89062=CARTESIAN_POINT ( 'NONE',  ( -68.31098214250890521, 1379.747686652805669, 279.8373429272113526 ) ) ;
#89066=EDGE_LOOP ( 'NONE', ( #89764, #58743 ) ) ;
#89069=CARTESIAN_POINT ( 'NONE',  ( -87.61701047141821164, 1384.975105123960020, 307.8438091251570086 ) ) ;
#89104=CARTESIAN_POINT ( 'NONE',  ( -7.573230445929720389, 1384.232072112190053, 219.0440869779680213 ) ) ;
#89119=CARTESIAN_POINT ( 'NONE',  ( -89.61547716558578713, 1384.619918949700150, 308.5733451897559689 ) ) ;
#89120=CARTESIAN_POINT ( 'NONE',  ( -43.09652149413830102, 1384.997786203090072, 216.0876167203250020 ) ) ;
#89137=CARTESIAN_POINT ( 'NONE',  ( -107.0758886263459999, 1391.913060387289988, 306.8605669363920470 ) ) ;
#89141=CARTESIAN_POINT ( 'NONE',  ( -12.98386958510000078, 1379.322232870260223, 207.9132534626290010 ) ) ;
#89153=CARTESIAN_POINT ( 'NONE',  ( -67.36707325840760063, 1379.746113040620003, 278.5175139230419745 ) ) ;
#89158=CARTESIAN_POINT ( 'NONE',  ( -105.1701064949999989, 1379.114530330549997, 304.0350749897590390 ) ) ;
#89159=CARTESIAN_POINT ( 'NONE',  ( -109.9851113750000025, 1384.920600747060007, 311.4561369192589950 ) ) ;
#89181=CARTESIAN_POINT ( 'NONE',  ( -8.581307173289999923, 1384.896522470129867, 218.6696871042690020 ) ) ;
#89183=CARTESIAN_POINT ( 'NONE',  ( -67.60155324206988325, 1379.745550781364045, 277.6215540139086784 ) ) ;
#89188=CARTESIAN_POINT ( 'NONE',  ( -57.84584034184130275, 1384.660072621870086, 239.4800334103370005 ) ) ;
#89217=DIRECTION ( 'NONE',  ( 0.07283688039883663701, -0.01177923247455932992, 0.9972743045602228129 ) ) ;
#89229=CARTESIAN_POINT ( 'NONE',  ( -106.2303729149999896, 1379.004472240850191, 307.4679664830589445 ) ) ;
#89254=CARTESIAN_POINT ( 'NONE',  ( -35.02326960185389737, 1384.808974036340032, 234.2283971188210216 ) ) ;
#89278=CARTESIAN_POINT ( 'NONE',  ( -86.98686869178300185, 1379.577998201610171, 300.8196123566030451 ) ) ;
#89281=CARTESIAN_POINT ( 'NONE',  ( -14.02644022332259865, 1379.579259008480221, 211.8354623865689916 ) ) ;
#89290=CARTESIAN_POINT ( 'NONE',  ( -7.544733521269999521, 1384.899971913130003, 219.0877090843589770 ) ) ;
#89313=EDGE_LOOP ( 'NONE', ( #14806, #74590, #47083, #32978, #67439 ) ) ;
#89315=CARTESIAN_POINT ( 'NONE',  ( -42.70366651140000158, 1379.809904802510118, 226.7036006354589972 ) ) ;
#89333=CARTESIAN_POINT ( 'NONE',  ( -67.90588950680000835, 1379.745915699690158, 278.2978613680589888 ) ) ;
#89342=CARTESIAN_POINT ( 'NONE',  ( -109.9987472809999929, 1384.808520183549945, 311.2744866012590137 ) ) ;
#89344=CARTESIAN_POINT ( 'NONE',  ( -22.65830243868510152, 1385.265625594450057, 222.2095871976100057 ) ) ;
#89384=CONICAL_SURFACE ( 'NONE', #67907, 8.000000000000003553, 0.02617993877989872875 ) ;
#89391=ADVANCED_BREP_SHAPE_REPRESENTATION ( '', ( #46279, #21632 ), #46788 ) ;
#89394=CARTESIAN_POINT ( 'NONE',  ( -109.2564495476770077, 1383.425552342079982, 311.0677364371869658 ) ) ;
#89401=ORIENTED_EDGE ( 'NONE', *, *, #526, .F. ) ;
#89412=DIRECTION ( 'NONE',  ( -1.836970198721024757E-16, -1.000000000000000000, -1.001483571081361959E-32 ) ) ;
#89457=ORIENTED_EDGE ( 'NONE', *, *, #39389, .T. ) ;
#89465=EDGE_CURVE ( 'NONE', #90041, #13675, #14386, .T. ) ;
#89502=CARTESIAN_POINT ( 'NONE',  ( -109.8888322889999927, 1385.262561173820131, 297.0413350713590148 ) ) ;
#89511=CARTESIAN_POINT ( 'NONE',  ( -30.76149245344669936, 1383.841116178839911, 228.6174415704900014 ) ) ;
#89519=CARTESIAN_POINT ( 'NONE',  ( -28.66947223450000237, 1379.875917421989925, 220.8353055514589869 ) ) ;
#89527=CARTESIAN_POINT ( 'NONE',  ( -10.82440957829840045, 1387.838188296759881, 217.4113806752309870 ) ) ;
#89536=CARTESIAN_POINT ( 'NONE',  ( -101.1010672691480181, 1385.223634408800081, 296.4705977010279980 ) ) ;
#89538=CARTESIAN_POINT ( 'NONE',  ( -68.27348358399999029, 1379.748432006229905, 279.1146441202590722 ) ) ;
#89550=CARTESIAN_POINT ( 'NONE',  ( -109.1248564459999955, 1385.804671263960017, 311.1746157432589825 ) ) ;
#89558=CARTESIAN_POINT ( 'NONE',  ( -8.024497890290000157, 1385.179405298659958, 218.7778930676890070 ) ) ;
#89590=CARTESIAN_POINT ( 'NONE',  ( -107.6348030694729943, 1384.897191107869958, 297.0734579783350000 ) ) ;
#89596=ORIENTED_EDGE ( 'NONE', *, *, #107944, .F. ) ;
#89598=CARTESIAN_POINT ( 'NONE',  ( 0.000000000000000000, 1384.913060387289988, 209.1218459572589836 ) ) ;
#89616=CARTESIAN_POINT ( 'NONE',  ( -95.18267266084710343, 1384.957561219689978, 310.0846393943140242 ) ) ;
#89617=CARTESIAN_POINT ( 'NONE',  ( -8.291911044340000814, 1385.641098659349836, 199.7466504416589999 ) ) ;
#89631=CARTESIAN_POINT ( 'NONE',  ( 3.552713678799999608E-15, 1384.913060387289988, 209.1218459572589836 ) ) ;
#89658=PLANE ( 'NONE',  #74212 ) ;
#89663=CARTESIAN_POINT ( 'NONE',  ( -99.83863661568889825, 1384.601139973999807, 310.8064402255530467 ) ) ;
#89664=CARTESIAN_POINT ( 'NONE',  ( -41.61181380557460585, 1384.993891243530015, 214.4858607009509797 ) ) ;
#89671=CARTESIAN_POINT ( 'NONE',  ( -109.3079486820000028, 1384.885661341739933, 311.2646263232589376 ) ) ;
#89685=CARTESIAN_POINT ( 'NONE',  ( -11.78917987459999850, 1378.809900039579816, 205.3323986359689854 ) ) ;
#89697=CARTESIAN_POINT ( 'NONE',  ( -68.32464321669628760, 1379.746866834220100, 279.9001328348240349 ) ) ;
#89698=ORIENTED_EDGE ( 'NONE', *, *, #33624, .F. ) ;
#89731=CARTESIAN_POINT ( 'NONE',  ( -67.31567742948190869, 1379.744923755474019, 277.0446396347198856 ) ) ;
#89735=CARTESIAN_POINT ( 'NONE',  ( -60.86138114716440128, 1384.678333052500193, 245.8750988077819954 ) ) ;
#89764=ORIENTED_EDGE ( 'NONE', *, *, #17302, .T. ) ;
#89765=CARTESIAN_POINT ( 'NONE',  ( -8.371550284740001402, 1384.904409945399948, 199.7750102909289751 ) ) ;
#89787=ADVANCED_FACE ( 'NONE', ( #97478 ), #36714, .F. ) ;
#89801=CARTESIAN_POINT ( 'NONE',  ( -33.01652097059809421, 1384.817001746299866, 231.5368980879269998 ) ) ;
#89804=CARTESIAN_POINT ( 'NONE',  ( -106.2219607800000176, 1378.969459979150088, 301.4482640438590693 ) ) ;
#89826=CARTESIAN_POINT ( 'NONE',  ( -86.31866470790001244, 1376.287402133280011, 302.0943157429590542 ) ) ;
#89830=EDGE_LOOP ( 'NONE', ( #90080, #40721, #5867, #77476 ) ) ;
#89833=DIRECTION ( 'NONE',  ( 1.836970198721029688E-16, 1.000000000000000000, -1.262177448353620010E-31 ) ) ;
#89837=CARTESIAN_POINT ( 'NONE',  ( -8.021758511559999860, 1384.613687009050182, 218.7789206626590044 ) ) ;
#89858=EDGE_CURVE ( 'NONE', #1545, #68662, #100247, .T. ) ;
#89860=CARTESIAN_POINT ( 'NONE',  ( -13.69973612571159904, 1380.327653692039803, 209.8720025058139811 ) ) ;
#89864=CARTESIAN_POINT ( 'NONE',  ( -57.14396138109999868, 1375.865580479029859, 252.3469708248590280 ) ) ;
#89875=CARTESIAN_POINT ( 'NONE',  ( -86.93521348900000589, 1384.624802884190103, 307.7215772890590415 ) ) ;
#89879=CARTESIAN_POINT ( 'NONE',  ( -65.06949576879998176, 1379.738499687689909, 272.5769493850589811 ) ) ;
#89887=CARTESIAN_POINT ( 'NONE',  ( -73.55227667629998223, 1384.892239458130007, 298.9565473808590355 ) ) ;
#89889=CARTESIAN_POINT ( 'NONE',  ( -30.24061963389690177, 1385.232462148140030, 228.2819463136630134 ) ) ;
#89914=CARTESIAN_POINT ( 'NONE',  ( -104.4841888330000046, 1390.137343023919811, 303.0785894239589879 ) ) ;
#89916=CARTESIAN_POINT ( 'NONE',  ( -105.4624709189999834, 1391.255327103129957, 304.2078109453590287 ) ) ;
#89923=CARTESIAN_POINT ( 'NONE',  ( 1.106990746626510029E-15, 1390.939237335599955, 209.1218459572589836 ) ) ;
#89934=( BOUNDED_CURVE ( )  B_SPLINE_CURVE ( 3, ( #52799, #8010, #85260, #102598 ),
 .UNSPECIFIED., .F., .F. ) 
 B_SPLINE_CURVE_WITH_KNOTS ( ( 4, 4 ),
 ( 6.131270930140640729, 6.235467248071880242 ),
 .UNSPECIFIED. ) 
 CURVE ( )  GEOMETRIC_REPRESENTATION_ITEM ( )  RATIONAL_B_SPLINE_CURVE ( ( 1.000000000000000000, 0.9990954652306247574, 0.9990954652306247574, 1.000000000000000000 ) ) 
 REPRESENTATION_ITEM ( '' )  );
#89938=CARTESIAN_POINT ( 'NONE',  ( -109.9987472829999859, 1382.340119938149883, 310.6123152972590447 ) ) ;
#89945=CARTESIAN_POINT ( 'NONE',  ( -8.039615859688613142, 1383.830106102227774, 199.5870606692544982 ) ) ;
#89970=CARTESIAN_POINT ( 'NONE',  ( -5.013264356492538099, 1375.413060387289761, 214.7179447576738482 ) ) ;
#89994=CARTESIAN_POINT ( 'NONE',  ( -24.13074931272349843, 1384.542629409289930, 202.9617085307660034 ) ) ;
#90018=CARTESIAN_POINT ( 'NONE',  ( -9.123213394318430147, 1384.511223218079977, 199.9709075427289804 ) ) ;
#90041=VERTEX_POINT ( 'NONE', #108644 ) ;
#90049=CARTESIAN_POINT ( 'NONE',  ( -39.22814701120859127, 1383.829334103110114, 240.4562005770879978 ) ) ;
#90052=CARTESIAN_POINT ( 'NONE',  ( -9.094910673856409389, 1384.931050598509955, 199.9427862989620053 ) ) ;
#90058=CARTESIAN_POINT ( 'NONE',  ( -25.83964422380000059, 1382.988494219330050, 203.6397759949089732 ) ) ;
#90064=ORIENTED_EDGE ( 'NONE', *, *, #72721, .T. ) ;
#90065=CARTESIAN_POINT ( 'NONE',  ( -9.447981863928919921, 1387.027753276099929, 218.0739194378299999 ) ) ;
#90076=CARTESIAN_POINT ( 'NONE',  ( -68.78243321479477856, 1379.747970891648492, 280.2954871354117472 ) ) ;
#90080=ORIENTED_EDGE ( 'NONE', *, *, #93484, .F. ) ;
#90088=CARTESIAN_POINT ( 'NONE',  ( -109.4227531280000107, 1386.586214323900094, 311.1300201212590082 ) ) ;
#90098=CARTESIAN_POINT ( 'NONE',  ( -8.310258910639999996, 1385.293885163340065, 218.6824948903590098 ) ) ;
#90110=CARTESIAN_POINT ( 'NONE',  ( -13.15516954878490097, 1379.513185257769919, 208.2695793304900178 ) ) ;
#90119=CARTESIAN_POINT ( 'NONE',  ( -16.33178904099999684, 1384.664735002020052, 200.5821943269089900 ) ) ;
#90149=CARTESIAN_POINT ( 'NONE',  ( -106.1880180564230045, 1391.823619149070055, 306.2181660491010007 ) ) ;
#90157=CARTESIAN_POINT ( 'NONE',  ( -85.62862489637198848, 1384.979837283239931, 306.9945860826840658 ) ) ;
#90159=CARTESIAN_POINT ( 'NONE',  ( -10.02009237210000059, 1387.031860423330045, 200.7242823892290176 ) ) ;
#90170=CARTESIAN_POINT ( 'NONE',  ( -109.0592861043541575, 1387.830987840716716, 297.5922214923872389 ) ) ;
#90201=CARTESIAN_POINT ( 'NONE',  ( -12.98673877210000072, 1379.902522067299969, 210.6698428602090019 ) ) ;
#90202=CARTESIAN_POINT ( 'NONE',  ( -99.14101470300249730, 1384.602434930499840, 310.7191070241219677 ) ) ;
#90203=CARTESIAN_POINT ( 'NONE',  ( -54.62703117506750061, 1385.036901425090036, 233.1472692318469910 ) ) ;
#90209=EDGE_CURVE ( 'NONE', #73303, #7907, #75330, .T. ) ;
#90212=CARTESIAN_POINT ( 'NONE',  ( -109.9849726249999975, 1384.916895159399928, 311.4561123682589709 ) ) ;
#90238=CARTESIAN_POINT ( 'NONE',  ( -68.37927156717290700, 1379.746995951000144, 279.9669834283100158 ) ) ;
#90251=CARTESIAN_POINT ( 'NONE',  ( -107.6068470358870002, 1378.913060387289988, 307.9810573902719852 ) ) ;
#90257=ORIENTED_EDGE ( 'NONE', *, *, #9115, .T. ) ;
#90267=CARTESIAN_POINT ( 'NONE',  ( -63.86841275767449133, 1379.736337741658417, 269.9166081863446607 ) ) ;
#90272=CARTESIAN_POINT ( 'NONE',  ( -86.45468328506269984, 1384.824127158329929, 290.0207638261140346 ) ) ;
#90280=ORIENTED_EDGE ( 'NONE', *, *, #32300, .F. ) ;
#90302=CARTESIAN_POINT ( 'NONE',  ( -109.9987472800000035, 1386.462030370639923, 311.2689672492589921 ) ) ;
#90304=CARTESIAN_POINT ( 'NONE',  ( -7.965810472619998528, 1384.899971912439923, 199.4892297391889997 ) ) ;
#90333=CARTESIAN_POINT ( 'NONE',  ( -12.31045119098629925, 1378.376187953739873, 209.7947064970520046 ) ) ;
#90339=CARTESIAN_POINT ( 'NONE',  ( -32.57912550924620376, 1384.818706616959844, 230.9894701418880061 ) ) ;
#90342=CARTESIAN_POINT ( 'NONE',  ( -105.6288279289999963, 1378.913059789030058, 304.0441755682590497 ) ) ;
#90364=CARTESIAN_POINT ( 'NONE',  ( -52.99573173910000179, 1376.645807390780192, 254.2473206627590230 ) ) ;
#90375=CARTESIAN_POINT ( 'NONE',  ( -7.906113842649999057, 1383.697730676289893, 218.7671565430789826 ) ) ;
#90392=CARTESIAN_POINT ( 'NONE',  ( -108.8765025263714250, 1387.919848751604832, 310.7253640878452075 ) ) ;
#90395=CARTESIAN_POINT ( 'NONE',  ( -12.31717236926220060, 1378.347777968080209, 209.6423893116530337 ) ) ;
#90399=CARTESIAN_POINT ( 'NONE',  ( -43.72451106999999837, 1377.617442312380035, 225.9983715054590050 ) ) ;
#90414=CARTESIAN_POINT ( 'NONE',  ( -49.74528571340000838, 1383.812288545099818, 260.8378110853589646 ) ) ;
#90418=CARTESIAN_POINT ( 'NONE',  ( -60.14896982169999973, 1379.725317057869916, 261.7476106778590292 ) ) ;
#90431=CARTESIAN_POINT ( 'NONE',  ( -43.53222241470000142, 1389.577826452589989, 221.0279022753590255 ) ) ;
#90433=CARTESIAN_POINT ( 'NONE',  ( -34.27198354733999963, 1385.212855379749953, 233.1604131954400145 ) ) ;
#90462=CARTESIAN_POINT ( 'NONE',  ( -105.5834716709999981, 1391.919560845880142, 303.0663598160589913 ) ) ;
#90471=DIRECTION ( 'NONE',  ( 1.836970198721029688E-16, 1.000000000000000000, 0.000000000000000000 ) ) ;
#90551=CARTESIAN_POINT ( 'NONE',  ( -9.123736379228210680, 1384.508619151900120, 199.9712811155520171 ) ) ;
#90555=CARTESIAN_POINT ( 'NONE',  ( -68.74502848580000602, 1379.747981523659973, 280.1360247429590231 ) ) ;
#90570=CARTESIAN_POINT ( 'NONE',  ( -9.093469788365199591, 1384.772129490919951, 199.9460114921000127 ) ) ;
#90592=CARTESIAN_POINT ( 'NONE',  ( -105.0581303879369983, 1379.236400313860031, 304.0328620142400382 ) ) ;
#90608=CARTESIAN_POINT ( 'NONE',  ( -42.86424717262820394, 1383.823646364319757, 247.0049435532770019 ) ) ;
#90616=CARTESIAN_POINT ( 'NONE',  ( -20.42369457250000053, 1378.928569551019791, 210.5700358550290048 ) ) ;
#90622=CARTESIAN_POINT ( 'NONE',  ( -12.02121513377869988, 1389.043580930620010, 215.7482713796579787 ) ) ;
#90626=CARTESIAN_POINT ( 'NONE',  ( -104.5162234509999877, 1380.028246613130023, 301.8403285842589412 ) ) ;
#90644=CARTESIAN_POINT ( 'NONE',  ( -109.0249265700000052, 1386.996120149900207, 310.9016331512590341 ) ) ;
#90705=CARTESIAN_POINT ( 'NONE',  ( -105.7715901379339982, 1391.141931180460006, 306.3730337667240065 ) ) ;
#90716=CARTESIAN_POINT ( 'NONE',  ( -77.89391513553759694, 1384.999643260920038, 302.3909578806699869 ) ) ;
#90718=CARTESIAN_POINT ( 'NONE',  ( -8.508434771949998421, 1386.782168888490105, 200.0040007541689988 ) ) ;
#90757=CARTESIAN_POINT ( 'NONE',  ( -104.0156867654433057, 1380.207460468658610, 306.5247186736235108 ) ) ;
#90761=AXIS2_PLACEMENT_3D ( 'NONE', #89923, #90471, #12116 ) ;
#90766=CARTESIAN_POINT ( 'NONE',  ( -52.24432420902090257, 1385.027339147369958, 228.9037425557689858 ) ) ;
#90776=CARTESIAN_POINT ( 'NONE',  ( -109.3084789200000131, 1384.717857449120174, 311.2599033892590228 ) ) ;
#90790=CARTESIAN_POINT ( 'NONE',  ( -5.243603173628749836, 1374.986671669950056, 203.4237121730149909 ) ) ;
#90797=CARTESIAN_POINT ( 'NONE',  ( -68.07780588669999133, 1379.747638516110101, 279.5234925687589680 ) ) ;
#90801=ORIENTED_EDGE ( 'NONE', *, *, #17302, .F. ) ;
#90809=CARTESIAN_POINT ( 'NONE',  ( -14.29934916198160089, 1379.719590493410124, 208.2697206714749996 ) ) ;
#90811=SHAPE_DEFINITION_REPRESENTATION ( #73286, #105979 ) ;
#90830=CARTESIAN_POINT ( 'NONE',  ( -80.12204894687070578, 1384.794894040560166, 283.2630655434839468 ) ) ;
#90840=CARTESIAN_POINT ( 'NONE',  ( -109.1111611177930030, 1384.583257041720117, 311.2497810013429671 ) ) ;
#90880=FACE_OUTER_BOUND ( 'NONE', #95782, .T. ) ;
#90885=B_SPLINE_CURVE_WITH_KNOTS ( 'NONE', 3,
 ( #17338, #91870, #7320, #42029, #23558, #24635, #93512, #8966, #94069, #24095, #51532, #8404, #33600, #7862, #40, #41483, #34171, #75644, #92969, #16241, #31964, #50987, #15144, #59953, #109243, #110327, #100807, #50446, #84570, #25197, #58284, #92409, #109783, #76178, #49886, #67795, #101905, #85116, #42576, #20125, #95187, #36927, #104686, #1146, #593, #86226 ),
 .UNSPECIFIED., .F., .F.,
 ( 4, 3, 3, 3, 3, 3, 3, 3, 3, 3, 3, 3, 3, 3, 3, 4 ),
 ( -11.22311477689549974, -10.99415920655549961, -10.18995056570000024, -9.361206530017639693, -8.517487667444680000, -7.615611964294410008, -6.760125105125089462, -5.916206473942639654, -5.089590486009999637, -4.554350324856789811, -3.682921093262059742, -2.834315530205490319, -1.999665612459999409, -1.587483130849479451, -0.7852278221460000651, 0.000000000000000000 ),
 .UNSPECIFIED. ) ;
#90902=CARTESIAN_POINT ( 'NONE',  ( -43.62562285640520088, 1384.770753572229978, 248.8406183467260178 ) ) ;
#90903=CARTESIAN_POINT ( 'NONE',  ( -106.7351624162349992, 1391.913060387289988, 302.3468487761870165 ) ) ;
#90926=CARTESIAN_POINT ( 'NONE',  ( 8.985389986235038126E-14, 1377.122490972250034, 211.4935542023889923 ) ) ;
#90928=CARTESIAN_POINT ( 'NONE',  ( -19.20715834270519906, 1379.591600376749966, 212.8172136241779810 ) ) ;
#90930=ORIENTED_EDGE ( 'NONE', *, *, #4296, .F. ) ;
#90957=CARTESIAN_POINT ( 'NONE',  ( -12.63123455407130002, 1379.447564691009802, 208.9815245622429813 ) ) ;
#90959=FACE_OUTER_BOUND ( 'NONE', #72950, .T. ) ;
#90961=CARTESIAN_POINT ( 'NONE',  ( -55.86512535760000020, 1379.936376805820146, 252.9328197421589834 ) ) ;
#90971=CARTESIAN_POINT ( 'NONE',  ( -5.932239102140000497, 1391.413060387289988, 209.1218459572589836 ) ) ;
#90973=CARTESIAN_POINT ( 'NONE',  ( -59.29940820010000380, 1384.093480151519998, 279.8903676332589612 ) ) ;
#90986=CARTESIAN_POINT ( 'NONE',  ( -39.01488008110000294, 1388.283545533540064, 213.2677783093589881 ) ) ;
#90988=CARTESIAN_POINT ( 'NONE',  ( -51.04972207953789365, 1385.115692561849983, 263.8849342485610237 ) ) ;
#91014=CARTESIAN_POINT ( 'NONE',  ( -105.5401914130000023, 1388.839035077719927, 299.4423369547589573 ) ) ;
#91020=CARTESIAN_POINT ( 'NONE',  ( -105.0271776439999911, 1379.361271506249977, 303.6846696449590013 ) ) ;
#91037=CARTESIAN_POINT ( 'NONE',  ( -113.4000000000000057, 1383.459135650929966, 297.2218459572590064 ) ) ;
#91070=EDGE_CURVE ( 'NONE', #74400, #49086, #84677, .T. ) ;
#91071=CARTESIAN_POINT ( 'NONE',  ( -8.849931646880000002, 1384.677929302499933, 199.9332806424890236 ) ) ;
#91098=CARTESIAN_POINT ( 'NONE',  ( -18.05215045752869685, 1384.529053208030064, 201.2145023365150109 ) ) ;
#91166=CARTESIAN_POINT ( 'NONE',  ( -41.53790650758289615, 1383.825758773150028, 244.5308847209749956 ) ) ;
#91170=CARTESIAN_POINT ( 'NONE',  ( -113.4000000000000057, 1390.913060387289988, 304.2218459572590064 ) ) ;
#91175=CARTESIAN_POINT ( 'NONE',  ( -16.32897964160000370, 1384.525298249519892, 200.5993092285889929 ) ) ;
#91177=ORIENTED_EDGE ( 'NONE', *, *, #42524, .T. ) ;
#91178=ORIENTED_EDGE ( 'NONE', *, *, #26821, .T. ) ;
#91180=CARTESIAN_POINT ( 'NONE',  ( -7.567236696338139446, 1385.515642188830270, 219.0512315761490072 ) ) ;
#91185=CARTESIAN_POINT ( 'NONE',  ( -106.5438666130000058, 1380.603607321050049, 299.5701110033589316 ) ) ;
#91191=CARTESIAN_POINT ( 'NONE',  ( -66.90724276829999440, 1379.748944712210005, 276.4281807783590352 ) ) ;
#91203=CARTESIAN_POINT ( 'NONE',  ( -109.5704612849999933, 1384.938891529579905, 311.3082982532590108 ) ) ;
#91236=CARTESIAN_POINT ( 'NONE',  ( -62.44985522310000192, 1384.688102815929824, 249.3037632142590212 ) ) ;
#91263=CARTESIAN_POINT ( 'NONE',  ( -108.4300409128252767, 1381.105006665046176, 298.0805022167543257 ) ) ;
#91275=CARTESIAN_POINT ( 'NONE',  ( -90.01380978207909322, 1384.969498126610006, 308.7154665456239968 ) ) ;
#91276=CARTESIAN_POINT ( 'NONE',  ( -9.221393643380000782, 1387.134211727530101, 200.5164217425590039 ) ) ;
#91288=CARTESIAN_POINT ( 'NONE',  ( -109.7434571511378323, 1386.572387547986409, 297.1542559680822819 ) ) ;
#91314=CARTESIAN_POINT ( 'NONE',  ( -105.1388918222897502, 1380.999031973004776, 308.5443376699517444 ) ) ;
#91323=CARTESIAN_POINT ( 'NONE',  ( -61.39718882775409980, 1385.068252780349894, 247.0266603675090096 ) ) ;
#91334=CARTESIAN_POINT ( 'NONE',  ( -109.4795670820000026, 1384.638871926420052, 311.2744876122590085 ) ) ;
#91357=CARTESIAN_POINT ( 'NONE',  ( -109.1253053317170014, 1384.665560649159943, 311.2565095416410372 ) ) ;
#91359=CARTESIAN_POINT ( 'NONE',  ( -68.71179394108339977, 1379.747778244289975, 280.3126260626940507 ) ) ;
#91363=CARTESIAN_POINT ( 'NONE',  ( -8.640836516204634776, 1381.414239460393446, 218.0276686012663845 ) ) ;
#91371=CARTESIAN_POINT ( 'NONE',  ( -106.8945970612549985, 1378.913060387289988, 307.0349506131610156 ) ) ;
#91381=EDGE_LOOP ( 'NONE', ( #13803, #89457, #42, #103018 ) ) ;
#91390=CARTESIAN_POINT ( 'NONE',  ( -14.47191441250000032, 1379.648773486759865, 208.1784591346629725 ) ) ;
#91396=CARTESIAN_POINT ( 'NONE',  ( -77.91920755176590774, 1384.783552880790239, 280.1696958822980150 ) ) ;
#91463=CARTESIAN_POINT ( 'NONE',  ( -51.76569597015449631, 1384.731644114589926, 265.3596788363910264 ) ) ;
#91478=CARTESIAN_POINT ( 'NONE',  ( -12.26117242810740038, 1377.986604079799918, 210.3392675169330346 ) ) ;
#91487=CARTESIAN_POINT ( 'NONE',  ( -18.12558133263030058, 1378.944431349770184, 212.8996372240309825 ) ) ;
#91490=CARTESIAN_POINT ( 'NONE',  ( -52.42853552719999755, 1379.742143313350198, 249.9106425961589935 ) ) ;
#91517=CARTESIAN_POINT ( 'NONE',  ( -109.0049894526701024, 1387.725350813251225, 310.8181635293149725 ) ) ;
#91524=CARTESIAN_POINT ( 'NONE',  ( -51.56180980459999574, 1375.317619266380007, 241.8087128081590151 ) ) ;
#91537=CARTESIAN_POINT ( 'NONE',  ( -43.14264924749999608, 1384.135846318449921, 247.4751904553590123 ) ) ;
#91550=CARTESIAN_POINT ( 'NONE',  ( -72.88336126909999280, 1389.495380267770088, 278.2578877944589522 ) ) ;
#91552=CARTESIAN_POINT ( 'NONE',  ( -41.62168732680330407, 1385.172644076110146, 245.0246584883539924 ) ) ;
#91562=CARTESIAN_POINT ( 'NONE',  ( -8.861701196289999416, 1384.879576664679917, 218.6850102892290124 ) ) ;
#91580=CARTESIAN_POINT ( 'NONE',  ( -105.3239982070000025, 1388.772974685380177, 299.3169349243589750 ) ) ;
#91582=CARTESIAN_POINT ( 'NONE',  ( -106.1567761860000019, 1391.062835315139864, 301.1121260340589743 ) ) ;
#91684=CARTESIAN_POINT ( 'NONE',  ( -8.888009947380730580, 1385.310821826299843, 218.6609850379070110 ) ) ;
#91715=CARTESIAN_POINT ( 'NONE',  ( -52.16017755504229569, 1383.808392896499981, 265.7696805365019941 ) ) ;
#91723=CARTESIAN_POINT ( 'NONE',  ( -49.74528571340000838, 1383.812288545099818, 260.8378110853589646 ) ) ;
#91726=VERTEX_POINT ( 'NONE', #57873 ) ;
#91728=CARTESIAN_POINT ( 'NONE',  ( -7.614648265717109510, 1386.000035739249824, 218.9991509990680072 ) ) ;
#91733=CARTESIAN_POINT ( 'NONE',  ( -106.9986950340000078, 1380.006134006080174, 299.5043260916589816 ) ) ;
#91778=CARTESIAN_POINT ( 'NONE',  ( -73.11457663749999369, 1384.756954744069844, 272.3426209276589702 ) ) ;
#91783=CARTESIAN_POINT ( 'NONE',  ( -105.2826783650000095, 1379.306804825290101, 305.8448452370589621 ) ) ;
#91811=CARTESIAN_POINT ( 'NONE',  ( -10.69978296939999929, 1378.845154982549957, 215.3071352179290159 ) ) ;
#91817=CARTESIAN_POINT ( 'NONE',  ( -109.1309839890330124, 1384.924126711810004, 311.2646841801559958 ) ) ;
#91820=CARTESIAN_POINT ( 'NONE',  ( -8.672397137009999923, 1387.672506191870070, 200.2132856537890007 ) ) ;
#91852=DIRECTION ( 'NONE',  ( 1.836970198721029688E-16, 1.000000000000000000, -7.703719777548939991E-34 ) ) ;
#91855=CARTESIAN_POINT ( 'NONE',  ( -109.5357277100000033, 1384.884655545610030, 297.1232340666590517 ) ) ;
#91860=CARTESIAN_POINT ( 'NONE',  ( -103.5791577002006392, 1379.885278930973300, 304.2740119158704601 ) ) ;
#91867=CARTESIAN_POINT ( 'NONE',  ( -12.27511545770000012, 1378.749906411379925, 210.4255720796790285 ) ) ;
#91869=CARTESIAN_POINT ( 'NONE',  ( -65.40580218510729082, 1385.088756549790105, 255.9493206941889696 ) ) ;
#91870=CARTESIAN_POINT ( 'NONE',  ( -11.66480462916690009, 1391.913060387289988, 209.7483395150459842 ) ) ;
#91893=ORIENTED_EDGE ( 'NONE', *, *, #10293, .F. ) ;
#91894=CARTESIAN_POINT ( 'NONE',  ( -109.1178393244110083, 1384.617941813639845, 311.2528399063589859 ) ) ;
#91896=CARTESIAN_POINT ( 'NONE',  ( -68.69558181574110733, 1379.747740281419965, 280.2958428208029886 ) ) ;
#91932=CARTESIAN_POINT ( 'NONE',  ( -11.15533026760000013, 1391.364751240080068, 214.3594460478390147 ) ) ;
#91933=CARTESIAN_POINT ( 'NONE',  ( -79.74970074852699042, 1384.793032888219841, 282.7736550586030262 ) ) ;
#91966=CARTESIAN_POINT ( 'NONE',  ( -9.094256809820000953, 1384.874748782070128, 199.9429996847190125 ) ) ;
#91979=ORIENTED_EDGE ( 'NONE', *, *, #68499, .F. ) ;
#91984=ADVANCED_FACE ( 'NONE', ( #39820 ), #29586, .T. ) ;
#92006=CARTESIAN_POINT ( 'NONE',  ( -55.97596842464690070, 1384.712463620669951, 273.6909236772529539 ) ) ;
#92035=CARTESIAN_POINT ( 'NONE',  ( -34.44898256530730407, 1379.727502236150031, 221.8237690217300155 ) ) ;
#92037=CARTESIAN_POINT ( 'NONE',  ( -36.56818187949999555, 1379.727990716889963, 223.6839165909590008 ) ) ;
#92064=CARTESIAN_POINT ( 'NONE',  ( -109.8609801027910322, 1385.943261636451552, 311.3663857728728885 ) ) ;
#92070=CARTESIAN_POINT ( 'NONE',  ( -11.47183536569999873, 1375.342188321910044, 208.5259290606699949 ) ) ;
#92083=CARTESIAN_POINT ( 'NONE',  ( -36.16775626039999736, 1384.153367539769988, 235.4370147729590030 ) ) ;
#92095=CARTESIAN_POINT ( 'NONE',  ( -62.45667138380000694, 1385.073369564110180, 249.3006260568589880 ) ) ;
#92097=CARTESIAN_POINT ( 'NONE',  ( -39.07382109423490135, 1385.187229302069909, 240.5099285539480150 ) ) ;
#92099=B_SPLINE_SURFACE_WITH_KNOTS ( 'NONE', 5, 5, ( 
 ( #4285, #88829, #99410, #107276, #21599, #56889, #55804, #63120, #48498 ),
 ( #30571, #12671, #82065, #29460, #91020, #20492, #38413, #64761, #80435 ),
 ( #54702, #98872, #82638, #5370, #3749, #39529, #73704, #37881, #72065 ),
 ( #24511, #56497, #74413, #48658, #32922, #6078, #76045, #40230, #15007 ),
 ( #58701, #14465, #82784, #65461, #108538, #99019, #90626, #82233, #99568 ),
 ( #92833, #49753, #107980, #31828, #22853, #73853, #66015, #67112, #41343 ),
 ( #40783, #13906, #74960, #48093, #100137, #109109, #57617, #49205, #22295 ),
 ( #15553, #23423, #91733, #7188, #91185, #83333, #32388, #66571, #58153 ),
 ( #5532, #6629, #100676, #23958, #92283, #83883, #75512, #39685, #101214 ),
 ( #16109, #109646, #50313, #84442, #7726, #41887, #31277, #57058, #110189 ),
 ( #33462, #35690, #68772, #76591, #69321, #69880, #9390, #78809, #25616 ),
 ( #59808, #101770, #61474, #43553, #18869, #93927, #77702, #53066, #110742 ),
 ( #60924, #103428, #78245, #17194, #84974, #463, #8268, #27293, #1013 ),
 ( #87204, #60357, #25061, #44667, #67663, #35139, #51391, #52512, #85524 ),
 ( #16648, #8818, #77160, #42433, #59263, #93381, #43003, #95601, #26736 ),
 ( #34586, #86642, #102873, #10495, #50844, #26170, #94479, #34034, #68224 ),
 ( #17752, #2122, #95053, #18321, #9937, #44110, #102330, #1557, #103995 ),
 ( #51955, #86096, #104555, #11603, #96718, #81006, #54182, #13225, #88310 ) ),
 .UNSPECIFIED., .F., .F., .F.,
 ( 6, 3, 3, 3, 3, 6 ),
 ( 6, 3, 6 ),
 ( 26.14460235269999799, 29.70143520729999764, 36.87935098730000050, 40.57606074569999777, 43.18675127440000239, 48.00176651980000031 ),
 ( 0.000000000000000000, 1.000000000000000000, 2.000000000000000000 ),
 .UNSPECIFIED. ) ;
#92108=CARTESIAN_POINT ( 'NONE',  ( -7.769184196640000373, 1384.903524103370046, 218.9178905665889943 ) ) ;
#92126=CARTESIAN_POINT ( 'NONE',  ( -104.6872550750000102, 1390.001717484610026, 301.9815041924589991 ) ) ;
#92128=CARTESIAN_POINT ( 'NONE',  ( -106.7924537439999995, 1391.913060387289988, 301.4346793793589541 ) ) ;
#92159=CARTESIAN_POINT ( 'NONE',  ( -7.567241880450000124, 1385.515695150829970, 219.0512258816089854 ) ) ;
#92170=EDGE_LOOP ( 'NONE', ( #30632, #23878, #30768, #20426 ) ) ;
#92180=CARTESIAN_POINT ( 'NONE',  ( -7.965810903780000451, 1384.899971913130003, 199.4892300885790064 ) ) ;
#92201=CARTESIAN_POINT ( 'NONE',  ( -29.53767091413150325, 1384.555073608529938, 205.3427205205709924 ) ) ;
#92220=ORIENTED_EDGE ( 'NONE', *, *, #102340, .F. ) ;
#92221=CARTESIAN_POINT ( 'NONE',  ( -7.966081143649218710, 1384.918389534460175, 199.4892681243580057 ) ) ;
#92223=CARTESIAN_POINT ( 'NONE',  ( -5.959028607229999608, 1385.182909178320187, 218.5168903876589752 ) ) ;
#92246=CARTESIAN_POINT ( 'NONE',  ( -7.545064063707340729, 1384.907232462019920, 219.0876311385090105 ) ) ;
#92258=EDGE_LOOP ( 'NONE', ( #21027, #41509, #21367, #88194 ) ) ;
#92267=CARTESIAN_POINT ( 'NONE',  ( -46.21053394692320637, 1383.818180755360117, 253.5808621639829994 ) ) ;
#92275=CARTESIAN_POINT ( 'NONE',  ( -62.44985522310000192, 1384.688102815929824, 249.3037632142590212 ) ) ;
#92283=CARTESIAN_POINT ( 'NONE',  ( -107.1973146609999930, 1381.194866720909886, 298.8585007089590135 ) ) ;
#92286=DIRECTION ( 'NONE',  ( 0.000000000000000000, 0.000000000000000000, -1.000000000000000000 ) ) ;
#92300=CARTESIAN_POINT ( 'NONE',  ( -105.2357120539999897, 1390.250932512190047, 306.4420972570590038 ) ) ;
#92315=CARTESIAN_POINT ( 'NONE',  ( -1.658081806242819971E-15, 1375.886883438980021, 209.1218459572589836 ) ) ;
#92327=CARTESIAN_POINT ( 'NONE',  ( -39.76976369060000138, 1384.853131567590026, 212.4474779504389801 ) ) ;
#92337=CARTESIAN_POINT ( 'NONE',  ( -10.86466539000899978, 1391.913060387130145, 205.6479294918659946 ) ) ;
#92340=ORIENTED_EDGE ( 'NONE', *, *, #59839, .F. ) ;
#92357=CARTESIAN_POINT ( 'NONE',  ( -13.12553963729999928, 1379.406087309789882, 211.7521819623089812 ) ) ;
#92363=CARTESIAN_POINT ( 'NONE',  ( -12.91306700440000022, 1390.089741809970064, 205.6071646888290161 ) ) ;
#92374=CARTESIAN_POINT ( 'NONE',  ( -107.7676061301826280, 1389.569596624323367, 298.7085081970911915 ) ) ;
#92399=DIRECTION ( 'NONE',  ( -0.3170185151553819858, -0.9051242360756870386, -0.2832832122048195012 ) ) ;
#92403=CARTESIAN_POINT ( 'NONE',  ( -107.3835680070587983, 1379.994974221857547, 309.2994170105861258 ) ) ;
#92404=CARTESIAN_POINT ( 'NONE',  ( -14.01398736212220086, 1379.590348564800024, 211.9184487047760115 ) ) ;
#92406=CARTESIAN_POINT ( 'NONE',  ( -14.18177803620000077, 1380.146094623469935, 210.8656358578390098 ) ) ;
#92408=CARTESIAN_POINT ( 'NONE',  ( -57.68740113826780203, 1385.050377599670128, 239.1317386132739955 ) ) ;
#92409=CARTESIAN_POINT ( 'NONE',  ( -10.64049728136139983, 1391.913060387289988, 213.3044660420850107 ) ) ;
#92434=CARTESIAN_POINT ( 'NONE',  ( -68.48768668117180880, 1379.747307472329794, 280.1013031988870239 ) ) ;
#92466=CARTESIAN_POINT ( 'NONE',  ( -12.33854995039999913, 1378.601075279359975, 208.9290456525660034 ) ) ;
#92470=CARTESIAN_POINT ( 'NONE',  ( -11.02757116259999925, 1391.621866938430003, 214.2885041620889979 ) ) ;
#92472=CARTESIAN_POINT ( 'NONE',  ( -68.65280262021799729, 1384.728655164589782, 263.0730744108470276 ) ) ;
#92490=CARTESIAN_POINT ( 'NONE',  ( -47.82285893009999711, 1379.680498130210026, 235.2466082674589813 ) ) ;
#92511=CARTESIAN_POINT ( 'NONE',  ( -109.9610541615100061, 1384.376359339889859, 311.4294103760240091 ) ) ;
#92525=EDGE_CURVE ( 'NONE', #48273, #109170, #36078, .T. ) ;
#92544=CARTESIAN_POINT ( 'NONE',  ( -45.47709076214669466, 1384.761897948679916, 252.4926689112959650 ) ) ;
#92545=CARTESIAN_POINT ( 'NONE',  ( -106.4032899763519993, 1391.913060387289988, 304.0478018970730432 ) ) ;
#92547=CARTESIAN_POINT ( 'NONE',  ( -107.2249090579999802, 1378.913060387289988, 300.8612202483589613 ) ) ;
#92550=DIRECTION ( 'NONE',  ( -1.000000000000000000, 0.000000000000000000, 0.000000000000000000 ) ) ;
#92573=CARTESIAN_POINT ( 'NONE',  ( -43.51401419724399489, 1380.083813360000022, 232.6619762463070060 ) ) ;
#92575=CARTESIAN_POINT ( 'NONE',  ( -36.30886271766330253, 1379.645996577580036, 223.9080834309320096 ) ) ;
#92581=CARTESIAN_POINT ( 'NONE',  ( -107.7196721970000084, 1378.913060387289988, 308.1225810710590167 ) ) ;
#92604=CARTESIAN_POINT ( 'NONE',  ( -108.0117080513960985, 1389.072098649294503, 309.9875421113430320 ) ) ;
#92608=ORIENTED_EDGE ( 'NONE', *, *, #54852, .T. ) ;
#92611=CARTESIAN_POINT ( 'NONE',  ( -3.771520291289999882, 1380.082072813469949, 207.5503167614189977 ) ) ;
#92625=CARTESIAN_POINT ( 'NONE',  ( -102.7375125960000020, 1384.595838641269893, 311.2202755702589911 ) ) ;
#92641=CARTESIAN_POINT ( 'NONE',  ( -59.61585404930000465, 1389.535794964619981, 250.6150333764589675 ) ) ;
#92643=CARTESIAN_POINT ( 'NONE',  ( -39.87565794312929768, 1385.182708064410235, 241.8885196562599731 ) ) ;
#92668=CARTESIAN_POINT ( 'NONE',  ( -109.7257039389999989, 1386.446923186560070, 297.1549502653589911 ) ) ;
#92693=CARTESIAN_POINT ( 'NONE',  ( -12.60774529335560779, 1379.062498616119001, 211.6870459221253498 ) ) ;
#92701=CARTESIAN_POINT ( 'NONE',  ( -12.29992035190429966, 1378.341876957339991, 209.9524196890029941 ) ) ;
#92718=CARTESIAN_POINT ( 'NONE',  ( -110.0630222465480017, 1384.919003957790210, 296.9512650941160246 ) ) ;
#92722=CARTESIAN_POINT ( 'NONE',  ( -8.154761128900000600, 1384.841831967909911, 199.6474426925889816 ) ) ;
#92741=EDGE_CURVE ( 'NONE', #7780, #32175, #37832, .T. ) ;
#92747=CARTESIAN_POINT ( 'NONE',  ( -35.55223107086649748, 1384.570145142690080, 209.1373044713860168 ) ) ;
#92755=CARTESIAN_POINT ( 'NONE',  ( -9.263518881979999620, 1384.040644720069849, 200.0636813112390087 ) ) ;
#92760=CARTESIAN_POINT ( 'NONE',  ( -68.68265996670000106, 1379.747811297680300, 279.9579939446590515 ) ) ;
#92776=FACE_OUTER_BOUND ( 'NONE', #38005, .T. ) ;
#92784=CARTESIAN_POINT ( 'NONE',  ( -8.875811585187578956, 1385.236883567939913, 218.6688581284889779 ) ) ;
#92796=CARTESIAN_POINT ( 'NONE',  ( -7.545023643077629849, 1384.923116630999857, 219.0875805831419996 ) ) ;
#92813=CARTESIAN_POINT ( 'NONE',  ( -13.82431552801049968, 1379.697172790399918, 208.1616873013680049 ) ) ;
#92817=CARTESIAN_POINT ( 'NONE',  ( -74.68581025115760497, 1383.781068242549964, 299.5368704359049730 ) ) ;
#92824=CARTESIAN_POINT ( 'NONE',  ( -49.82325338690000649, 1381.578505732160011, 226.8201688485589784 ) ) ;
#92828=CARTESIAN_POINT ( 'NONE',  ( -7.846308076728210068, 1385.913410601039914, 218.8401308622059958 ) ) ;
#92833=CARTESIAN_POINT ( 'NONE',  ( -106.2922410430000042, 1378.604080016899843, 300.8096223931590316 ) ) ;
#92854=CARTESIAN_POINT ( 'NONE',  ( -105.5819434490000077, 1390.739035477769903, 306.4716207183589631 ) ) ;
#92861=CARTESIAN_POINT ( 'NONE',  ( -9.123030677640000974, 1385.451960981700040, 199.9749920654289781 ) ) ;
#92886=CARTESIAN_POINT ( 'NONE',  ( -109.9857364230449974, 1384.899971927750130, 311.4562996732899478 ) ) ;
#92917=CARTESIAN_POINT ( 'NONE',  ( -10.49741166160000105, 1379.367595482069873, 215.6674695879490002 ) ) ;
#92924=CARTESIAN_POINT ( 'NONE',  ( -14.14948096550000045, 1390.186770710789915, 206.8378643784789972 ) ) ;
#92932=B_SPLINE_SURFACE_WITH_KNOTS ( 'NONE', 5, 5, ( 
 ( #54279, #80004, #4410, #43244, #37452, #97889 ),
 ( #38539, #89502, #34824, #62128, #29055, #11163 ),
 ( #106839, #2773, #36893, #63241, #97347, #72185 ),
 ( #51639, #20618, #29588, #54821, #88945, #12238 ),
 ( #46427, #80560, #3875, #38003, #55369, #74381 ),
 ( #32356, #98987, #40748, #64880, #83303, #55920 ) ),
 .UNSPECIFIED., .F., .F., .F.,
 ( 6, 6 ),
 ( 6, 6 ),
 ( 9.225465320329998775, 10.07010781710000025 ),
 ( 0.000000000000000000, 2.000000000000000000 ),
 .UNSPECIFIED. ) ;
#92945=CARTESIAN_POINT ( 'NONE',  ( -14.86200884888219953, 1383.858700832289969, 219.2304258842500246 ) ) ;
#92956=CARTESIAN_POINT ( 'NONE',  ( -109.3499934019999955, 1384.883594448820077, 297.1386964685590328 ) ) ;
#92957=ORIENTED_EDGE ( 'NONE', *, *, #62066, .T. ) ;
#92960=CARTESIAN_POINT ( 'NONE',  ( -105.2453956327515954, 1381.073543364039097, 308.6760955912837971 ) ) ;
#92963=CARTESIAN_POINT ( 'NONE',  ( -107.8212372937749421, 1380.513613017200441, 309.7939830466359581 ) ) ;
#92968=CARTESIAN_POINT ( 'NONE',  ( -75.71336797908890048, 1385.139485295300119, 276.6772571808519956 ) ) ;
#92969=CARTESIAN_POINT ( 'NONE',  ( -11.27004030100790111, 1391.913060387289988, 211.7974019302799888 ) ) ;
#92989=EDGE_LOOP ( 'NONE', ( #17445, #68996, #71995, #64882, #26407 ) ) ;
#92990=CARTESIAN_POINT ( 'NONE',  ( -109.1111611177930030, 1384.583257041720117, 311.2497810013429671 ) ) ;
#92992=CARTESIAN_POINT ( 'NONE',  ( -68.58042545469770346, 1379.747469642939905, 280.1935340281700633 ) ) ;
#92994=CARTESIAN_POINT ( 'NONE',  ( -8.233476245617373124, 1382.138012879694315, 218.4303649234365423 ) ) ;
#93019=CARTESIAN_POINT ( 'NONE',  ( -14.17425181905940157, 1380.106801343270035, 210.9147591587110071 ) ) ;
#93029=CARTESIAN_POINT ( 'NONE',  ( -103.4471835965699995, 1384.884903909179911, 296.7663910193570587 ) ) ;
#93046=CARTESIAN_POINT ( 'NONE',  ( -54.25698729759999850, 1379.746222734200046, 249.0120014888590276 ) ) ;
#93061=CARTESIAN_POINT ( 'NONE',  ( -8.604576478229999381, 1384.925130841180135, 199.8686410051190023 ) ) ;
#93097=CARTESIAN_POINT ( 'NONE',  ( -12.27558643317981790, 1391.355947415424453, 211.6931146922721894 ) ) ;
#93099=CARTESIAN_POINT ( 'NONE',  ( -56.29574522006849691, 1384.711066908519797, 274.2995360668660396 ) ) ;
#93108=CARTESIAN_POINT ( 'NONE',  ( -10.46358859826853838, 1379.681001781858413, 202.5371937123522912 ) ) ;
#93131=CARTESIAN_POINT ( 'NONE',  ( 7.886150497493308481E-14, 1379.061224848670008, 211.6703178456000103 ) ) ;
#93133=CARTESIAN_POINT ( 'NONE',  ( -48.10662876290690093, 1379.692216664059970, 241.4897638297360061 ) ) ;
#93139=CARTESIAN_POINT ( 'NONE',  ( -107.3950653609999932, 1379.272371631200031, 309.0941593425589531 ) ) ;
#93140=CARTESIAN_POINT ( 'NONE',  ( -109.6575144470000112, 1384.919424601119999, 311.3230338722590318 ) ) ;
#93167=ORIENTED_EDGE ( 'NONE', *, *, #20027, .F. ) ;
#93168=CARTESIAN_POINT ( 'NONE',  ( -104.4846036076890101, 1379.706327206979950, 304.5108243419020368 ) ) ;
#93176=CARTESIAN_POINT ( 'NONE',  ( -113.4000000000000057, 1383.754957750760013, 311.0314894602589675 ) ) ;
#93191=CARTESIAN_POINT ( 'NONE',  ( -53.47023167649999920, 1385.031515079650262, 230.7490043923590122 ) ) ;
#93193=CARTESIAN_POINT ( 'NONE',  ( -63.30007382191959664, 1385.050657975149988, 286.2646782049000080 ) ) ;
#93204=CARTESIAN_POINT ( 'NONE',  ( -107.4633657559999875, 1380.084902923649906, 309.4123343822590186 ) ) ;
#93221=CARTESIAN_POINT ( 'NONE',  ( -109.9909981520000031, 1385.946039747419945, 297.0141037326589526 ) ) ;
#93267=ORIENTED_EDGE ( 'NONE', *, *, #42522, .T. ) ;
#93293=CARTESIAN_POINT ( 'NONE',  ( -113.4000000000000057, 1379.413060387289988, 303.4364477938589744 ) ) ;
#93298=CARTESIAN_POINT ( 'NONE',  ( -32.52026698425390094, 1384.562322830350013, 207.0570309995399896 ) ) ;
#93300=CARTESIAN_POINT ( 'NONE',  ( -105.5485668489999966, 1388.544618357170066, 309.1779867852590655 ) ) ;
#93305=CARTESIAN_POINT ( 'NONE',  ( -49.40611499322205447, 1379.690198512848838, 244.6122530584670187 ) ) ;
#93311=CARTESIAN_POINT ( 'NONE',  ( -68.59203063350000207, 1379.747524784999996, 279.7276289599590200 ) ) ;
#93349=DIRECTION ( 'NONE',  ( 0.000000000000000000, -1.000000000000000000, 0.000000000000000000 ) ) ;
#93351=VERTEX_POINT ( 'NONE', #26326 ) ;
#93363=CARTESIAN_POINT ( 'NONE',  ( -64.14920489430819828, 1383.791463424650146, 287.2113058269809471 ) ) ;
#93370=CARTESIAN_POINT ( 'NONE',  ( -44.90575339929999643, 1380.945526020650050, 246.6134158280590043 ) ) ;
#93375=CARTESIAN_POINT ( 'NONE',  ( -9.252619606462529234, 1386.194650040039960, 218.4639876966940051 ) ) ;
#93381=CARTESIAN_POINT ( 'NONE',  ( -109.0917520289999914, 1383.655254917920047, 297.2994177358589809 ) ) ;
#93405=CARTESIAN_POINT ( 'NONE',  ( -107.0970161019999978, 1387.848630225089892, 309.9720921612589564 ) ) ;
#93438=CARTESIAN_POINT ( 'NONE',  ( -11.00165343754819958, 1391.913060387039877, 206.0010710664089970 ) ) ;
#93449=CARTESIAN_POINT ( 'NONE',  ( -9.853078183510000088, 1384.932634673870098, 199.8720430995890069 ) ) ;
#93457=CARTESIAN_POINT ( 'NONE',  ( -11.62355165729999840, 1378.295668984849954, 213.2764633795689804 ) ) ;
#93463=CARTESIAN_POINT ( 'NONE',  ( -11.91005457920000055, 1391.448248967449899, 205.5251632796090178 ) ) ;
#93464=CARTESIAN_POINT ( 'NONE',  ( -113.4589914632272212, 1390.913060387289988, 306.7211498618009387 ) ) ;
#93479=APPLICATION_CONTEXT ( 'automotive_design' ) ;
#93484=EDGE_CURVE ( 'NONE', #60257, #105885, #3718, .T. ) ;
#93487=CARTESIAN_POINT ( 'NONE',  ( -10.24703385824910029, 1383.862840724990065, 218.6056771012169975 ) ) ;
#93499=CARTESIAN_POINT ( 'NONE',  ( -110.0634901189999937, 1384.899971912280080, 296.9512051102590249 ) ) ;
#93506=CARTESIAN_POINT ( 'NONE',  ( -107.4791259594196617, 1380.106263187048626, 309.4148095461648609 ) ) ;
#93509=CARTESIAN_POINT ( 'NONE',  ( -11.42604309490000070, 1391.913060387289988, 207.1941759383389865 ) ) ;
#93510=CARTESIAN_POINT ( 'NONE',  ( -84.10063176446999478, 1385.173004153059992, 287.8709662445750155 ) ) ;
#93512=CARTESIAN_POINT ( 'NONE',  ( -11.62628111383389928, 1391.913060387289988, 210.2022570141400024 ) ) ;
#93530=DIRECTION ( 'NONE',  ( 0.000000000000000000, -1.000000000000000000, 0.000000000000000000 ) ) ;
#93537=CARTESIAN_POINT ( 'NONE',  ( -68.43502141645350889, 1379.747127445309843, 280.0327720878970013 ) ) ;
#93540=ORIENTED_EDGE ( 'NONE', *, *, #29533, .T. ) ;
#93548=( NAMED_UNIT ( * ) SI_UNIT ( $, .STERADIAN. ) SOLID_ANGLE_UNIT ( ) );
#93549=CARTESIAN_POINT ( 'NONE',  ( -12.32917350377740107, 1378.362683362840016, 209.4170945134390251 ) ) ;
#93562=CARTESIAN_POINT ( 'NONE',  ( -14.27857828532780182, 1380.308034680090032, 210.1943914574769963 ) ) ;
#93570=CARTESIAN_POINT ( 'NONE',  ( -103.8531838164470003, 1384.886124027839969, 296.8068726812870182 ) ) ;
#93586=CARTESIAN_POINT ( 'NONE',  ( -58.13411997410000254, 1379.718485381059963, 257.1571189129589925 ) ) ;
#93631=CARTESIAN_POINT ( 'NONE',  ( -12.02612939183720009, 1377.659857216290220, 211.7505375168460091 ) ) ;
#93636=CARTESIAN_POINT ( 'NONE',  ( -67.43312117150000518, 1384.669984925169956, 291.9984064737109861 ) ) ;
#93637=CARTESIAN_POINT ( 'NONE',  ( -24.94794202207559763, 1384.959512558119968, 203.2447943497110145 ) ) ;
#93643=CARTESIAN_POINT ( 'NONE',  ( -10.84436532123444508, 1379.243588034859386, 203.2049456427220946 ) ) ;
#93652=CARTESIAN_POINT ( 'NONE',  ( -12.47607414476330057, 1379.154200148260088, 210.8826634821560049 ) ) ;
#93666=CARTESIAN_POINT ( 'NONE',  ( -56.90245408136139815, 1379.713870185199994, 259.4980311760010068 ) ) ;
#93673=CARTESIAN_POINT ( 'NONE',  ( -109.3075263750000090, 1384.927480430210153, 311.2646524412589315 ) ) ;
#93700=CARTESIAN_POINT ( 'NONE',  ( -11.54050778900000118, 1375.649725832029844, 207.7392432702390295 ) ) ;
#93705=DIRECTION ( 'NONE',  ( -1.000000000000000000, 0.000000000000000000, 0.000000000000000000 ) ) ;
#93725=CARTESIAN_POINT ( 'NONE',  ( -67.09670646059998944, 1386.610685867510028, 292.1437283079590088 ) ) ;
#93727=CARTESIAN_POINT ( 'NONE',  ( -60.62638870901079713, 1385.063061064700150, 282.0167569604489586 ) ) ;
#93738=CARTESIAN_POINT ( 'NONE',  ( -109.0056894283609950, 1382.294289550630083, 310.8401910643229940 ) ) ;
#93752=CARTESIAN_POINT ( 'NONE',  ( -109.1450416020000063, 1385.242479493820156, 297.1468691531589457 ) ) ;
#93764=DIRECTION ( 'NONE',  ( 1.836970198721029688E-16, 1.000000000000000000, 0.000000000000000000 ) ) ;
#93788=CARTESIAN_POINT ( 'NONE',  ( -25.65041448810000091, 1380.250345454750004, 213.2122020707489867 ) ) ;
#93814=CARTESIAN_POINT ( 'NONE',  ( -12.50888813809999967, 1391.368279522899911, 208.1679514191799854 ) ) ;
#93819=ORIENTED_EDGE ( 'NONE', *, *, #74658, .F. ) ;
#93820=CARTESIAN_POINT ( 'NONE',  ( -5.013435694540000043, 1375.426148861440197, 203.5256706139790310 ) ) ;
#93827=ORIENTED_EDGE ( 'NONE', *, *, #101266, .F. ) ;
#93828=CARTESIAN_POINT ( 'NONE',  ( -109.5441724430000079, 1379.437034645699896, 303.4364478832590066 ) ) ;
#93839=CARTESIAN_POINT ( 'NONE',  ( -38.89130781446370122, 1384.579501196720003, 211.8816752983790082 ) ) ;
#93843=ORIENTED_EDGE ( 'NONE', *, *, #99050, .T. ) ;
#93846=CARTESIAN_POINT ( 'NONE',  ( -47.29346754776256034, 1379.682659667603048, 240.6734148706816825 ) ) ;
#93851=CARTESIAN_POINT ( 'NONE',  ( -68.70392287810000198, 1379.747767561100090, 279.9836365250589552 ) ) ;
#93857=CARTESIAN_POINT ( 'NONE',  ( -7.965680540240001051, 1384.926148861439970, 199.4891222871690104 ) ) ;
#93861=CARTESIAN_POINT ( 'NONE',  ( -2.142567804705589641E-15, 1385.055606633620073, 218.6218459572590120 ) ) ;
#93863=CARTESIAN_POINT ( 'NONE',  ( -105.2660175659031125, 1379.052920223518413, 304.0369892317328890 ) ) ;
#93887=UNCERTAINTY_MEASURE_WITH_UNIT (LENGTH_MEASURE( 1.000000000000000082E-05 ), #41656, 'distance_accuracy_value', 'NONE');
#93888=CARTESIAN_POINT ( 'NONE',  ( -7.545176580024880231, 1384.913154240279937, 219.0875923063640016 ) ) ;
#93889=DIRECTION ( 'NONE',  ( 1.000000000000000000, 0.000000000000000000, 0.000000000000000000 ) ) ;
#93909=CARTESIAN_POINT ( 'NONE',  ( -58.10467463043680425, 1383.799326198670087, 277.2797696228070095 ) ) ;
#93917=CARTESIAN_POINT ( 'NONE',  ( -58.29236204880000116, 1384.661700128139955, 240.0739325125589971 ) ) ;
#93927=CARTESIAN_POINT ( 'NONE',  ( -107.9739803319999965, 1382.432766417899984, 297.9312510628590189 ) ) ;
#93952=CARTESIAN_POINT ( 'NONE',  ( -107.7913657269999987, 1387.087163723699859, 310.5801087772589995 ) ) ;
#94003=CARTESIAN_POINT ( 'NONE',  ( -109.1324239101479918, 1384.847617670179943, 313.2643838898119952 ) ) ;
#94017=CARTESIAN_POINT ( 'NONE',  ( -12.02613236540000052, 1377.659859441090020, 211.7505269062990010 ) ) ;
#94025=CARTESIAN_POINT ( 'NONE',  ( -12.43556348120000088, 1391.700544350710061, 208.3488348747239911 ) ) ;
#94059=CARTESIAN_POINT ( 'NONE',  ( -13.33377604244770076, 1390.546217195540066, 210.7350625626099827 ) ) ;
#94065=B_SPLINE_CURVE_WITH_KNOTS ( 'NONE', 5,
 ( #43766, #1224, #35359, #61693, #44329, #61155, #95271, #78472, #1784, #35922, #104218, #19082, #42114, #54933, #20738, #89062, #11813, #80672, #12347, #44892, #79042, #29163, #63351, #2343, #55484, #96371, #28055, #36456, #98004, #105321, #2889, #28614, #72288, #45441, #106420, #37565, #81204, #88528, #38110, #72830, #45983, #10721, #79584, #54396, #70654, #19650, #12901, #97469 ),
 .UNSPECIFIED., .F., .F.,
 ( 6, 3, 3, 3, 3, 3, 3, 3, 3, 3, 3, 3, 3, 3, 3, 6 ),
 ( 0.000000000000000000, 0.001696444935363111695, 0.002566884068491868606, 0.004136085766892796077, 0.005705287465293942123, 0.008843690869748293756, 0.01637566666253125955, 0.02390764245531465729, 0.03884334483964269058, 0.08207802453382453955, 0.1535160673748799665, 0.2249756095436203363, 0.4745335301881646317, 0.7379578698543362014, 0.8518335909529411998, 1.000000000000000000 ),
 .UNSPECIFIED. ) ;
#94066=CARTESIAN_POINT ( 'NONE',  ( -13.50145109259999998, 1379.789977162729883, 211.3496610090389822 ) ) ;
#94067=CARTESIAN_POINT ( 'NONE',  ( -11.66658561999999932, 1391.913060387289988, 209.7120187064359982 ) ) ;
#94068=CARTESIAN_POINT ( 'NONE',  ( -85.93020247385199184, 1385.179414779810031, 289.5851895153920168 ) ) ;
#94069=CARTESIAN_POINT ( 'NONE',  ( -11.59266921033580111, 1391.913060387289988, 210.4631112540610047 ) ) ;
#94087=B_SPLINE_CURVE_WITH_KNOTS ( 'NONE', 5,
 ( #66400, #16486, #58539, #25446, #109486, #100519 ),
 .UNSPECIFIED., .F., .F.,
 ( 6, 6 ),
 ( 0.000000000000000000, 1.000000000000000000 ),
 .UNSPECIFIED. ) ;
#94106=CARTESIAN_POINT ( 'NONE',  ( -13.65428303350900130, 1379.630667800430047, 208.3402418708319885 ) ) ;
#94130=CARTESIAN_POINT ( 'NONE',  ( -105.1378806791870062, 1384.889948924000009, 296.9208209011409849 ) ) ;
#94146=CARTESIAN_POINT ( 'NONE',  ( -21.21955013839999893, 1379.607182551329970, 209.4272815681599980 ) ) ;
#94155=PRODUCT_DEFINITION_FORMATION_WITH_SPECIFIED_SOURCE ( 'ANY', '', #31272, .NOT_KNOWN. ) ;
#94167=CARTESIAN_POINT ( 'NONE',  ( -12.98386957539999997, 1379.322232868390074, 207.9132533945689829 ) ) ;
#94177=CARTESIAN_POINT ( 'NONE',  ( -113.4000000000000057, 1379.913060387289988, 304.2218459572590064 ) ) ;
#94199=CARTESIAN_POINT ( 'NONE',  ( -81.63561843131769535, 1384.635211739379884, 304.8817802514000164 ) ) ;
#94200=CARTESIAN_POINT ( 'NONE',  ( -14.30187964350709962, 1384.940608584799975, 200.5040086548420106 ) ) ;
#94215=CARTESIAN_POINT ( 'NONE',  ( -9.007783669269999294, 1383.959994898070136, 200.0643063390290024 ) ) ;
#94230=CARTESIAN_POINT ( 'NONE',  ( -63.22294501475990103, 1379.735052518850125, 271.8309557046729878 ) ) ;
#94238=CARTESIAN_POINT ( 'NONE',  ( -8.888756782119999755, 1385.314821197049923, 218.6605176087589939 ) ) ;
#94262=CARTESIAN_POINT ( 'NONE',  ( -58.97309372111901382, 1379.721245612332950, 259.0595248300897993 ) ) ;
#94263=CARTESIAN_POINT ( 'NONE',  ( -7.592224575779999540, 1380.058622747559866, 207.5503173039890044 ) ) ;
#94267=CARTESIAN_POINT ( 'NONE',  ( -105.4978708633500162, 1378.553056725880197, 304.5324165031829580 ) ) ;
#94289=CARTESIAN_POINT ( 'NONE',  ( -103.5315408879999950, 1389.439030332400080, 299.8536342697589703 ) ) ;
#94291=CARTESIAN_POINT ( 'NONE',  ( -68.14386999458439220, 1385.030899397170060, 292.8874234360349647 ) ) ;
#94301=CARTESIAN_POINT ( 'NONE',  ( -107.9316645854389947, 1381.454286385220257, 310.0668126409769911 ) ) ;
#94329=CARTESIAN_POINT ( 'NONE',  ( -13.52759590285629976, 1384.881001315799949, 219.1662475987569962 ) ) ;
#94383=CARTESIAN_POINT ( 'NONE',  ( -105.7140364779999970, 1379.461008902830145, 303.4364470169589936 ) ) ;
#94389=CARTESIAN_POINT ( 'NONE',  ( -68.70547844060000386, 1384.729371863979850, 263.4329467144589785 ) ) ;
#94390=CARTESIAN_POINT ( 'NONE',  ( -43.64178920747140467, 1384.594654343729871, 216.7300204284549920 ) ) ;
#94392=CARTESIAN_POINT ( 'NONE',  ( -104.4869036590000064, 1389.270867165570053, 307.8650956148590012 ) ) ;
#94402=CARTESIAN_POINT ( 'NONE',  ( -68.62999220760001151, 1379.747924320049833, 279.8460896497590511 ) ) ;
#94409=CARTESIAN_POINT ( 'NONE',  ( -59.22805538469999931, 1384.945537078079951, 279.9292060866590077 ) ) ;
#94411=CARTESIAN_POINT ( 'NONE',  ( -15.37547630988030001, 1385.293449114180021, 219.4910068333289814 ) ) ;
#94424=CARTESIAN_POINT ( 'NONE',  ( -8.864690188119949354, 1385.133112985140087, 218.6772544400749894 ) ) ;
#94429=ORIENTED_EDGE ( 'NONE', *, *, #62348, .F. ) ;
#94456=CARTESIAN_POINT ( 'NONE',  ( -66.89731259161800381, 1383.788378096659926, 291.0260303366639505 ) ) ;
#94468=CARTESIAN_POINT ( 'NONE',  ( -94.50912602849999189, 1384.855827234549906, 294.8620370673590401 ) ) ;
#94479=CARTESIAN_POINT ( 'NONE',  ( -109.2455494860000016, 1384.077694082239987, 297.1940690992589680 ) ) ;
#94502=CARTESIAN_POINT ( 'NONE',  ( -108.7149811449999959, 1387.932087793509936, 310.6222449872589664 ) ) ;
#94509=EDGE_CURVE ( 'NONE', #105177, #55324, #66381, .T. ) ;
#94554=CARTESIAN_POINT ( 'NONE',  ( -6.331822530929999360, 1388.284444344999883, 200.8293682005390224 ) ) ;
#94572=CARTESIAN_POINT ( 'NONE',  ( -12.43426257129999968, 1391.244016237139931, 206.9658053057590053 ) ) ;
#94608=ORIENTED_EDGE ( 'NONE', *, *, #27920, .T. ) ;
#94611=CARTESIAN_POINT ( 'NONE',  ( -14.43963703662210030, 1380.159948612549897, 209.0189137943660000 ) ) ;
#94615=EDGE_CURVE ( 'NONE', #29914, #99683, #1508, .T. ) ;
#94616=CARTESIAN_POINT ( 'NONE',  ( -108.6923101465634716, 1381.634892108574377, 310.5848204547120304 ) ) ;
#94620=CARTESIAN_POINT ( 'NONE',  ( -12.54019733330000008, 1391.397793261360221, 209.7548870936209937 ) ) ;
#94622=CARTESIAN_POINT ( 'NONE',  ( -71.90449437803688681, 1385.121734512539888, 269.7491603056169538 ) ) ;
#94656=ORIENTED_EDGE ( 'NONE', *, *, #34393, .T. ) ;
#94666=CARTESIAN_POINT ( 'NONE',  ( -12.84384240866459947, 1379.221145577220113, 208.6845722232019966 ) ) ;
#94688=CARTESIAN_POINT ( 'NONE',  ( -92.29727215281390329, 1384.847535221339967, 293.8106274702879546 ) ) ;
#94705=CARTESIAN_POINT ( 'NONE',  ( -16.50765472400000178, 1379.592255418909872, 208.3681221328770050 ) ) ;
#94731=CARTESIAN_POINT ( 'NONE',  ( 1.285879139104720042E-15, 1391.913060387289988, 209.1218459572589836 ) ) ;
#94755=B_SPLINE_SURFACE_WITH_KNOTS ( 'NONE', 5, 5, ( 
 ( #32029, #34230, #83523, #17400, #76240, #110387 ),
 ( #6277, #66218, #23625, #100337, #85179, #6817 ),
 ( #57808, #91932, #92470, #109303, #15206, #7922 ),
 ( #100865, #16299, #49396, #68416, #40976, #109846 ),
 ( #75156, #32589, #66765, #24156, #15741, #84080 ),
 ( #51046, #7378, #76791, #67310, #101407, #24698 ),
 ( #50503, #84625, #42092, #69524, #26942, #68970 ),
 ( #18508, #87967, #2321, #104745, #36431, #61131 ),
 ( #95245, #43198, #96905, #28033, #87403, #60567 ) ),
 .UNSPECIFIED., .F., .F., .F.,
 ( 6, 3, 6 ),
 ( 6, 6 ),
 ( 0.000000000000000000, 5.089590486009999637, 11.22315645349999969 ),
 ( 0.000000000000000000, 1.000000000000000000 ),
 .UNSPECIFIED. ) ;
#94757=EDGE_CURVE ( 'NONE', #43960, #73303, #199, .T. ) ;
#94763=CARTESIAN_POINT ( 'NONE',  ( -60.62730084387049345, 1384.693337083439928, 282.0175979611260004 ) ) ;
#94764=CARTESIAN_POINT ( 'NONE',  ( -5.511153256349440532, 1374.913063729909936, 214.9361186106310129 ) ) ;
#94769=CARTESIAN_POINT ( 'NONE',  ( -9.094910833689999308, 1384.931037369060050, 199.9427862008689942 ) ) ;
#94781=CARTESIAN_POINT ( 'NONE',  ( -7.989567385690000023, 1384.306347471770096, 199.5291465469090042 ) ) ;
#94798=CARTESIAN_POINT ( 'NONE',  ( -62.68882714082580065, 1379.739779185960060, 270.6182910835300390 ) ) ;
#94804=CARTESIAN_POINT ( 'NONE',  ( -107.3880028199999970, 1378.913060387289988, 307.7170154214589388 ) ) ;
#94819=CARTESIAN_POINT ( 'NONE',  ( -5.013337946330830519, 1375.421898367659878, 203.5257142815540305 ) ) ;
#94820=EDGE_LOOP ( 'NONE', ( #6428, #13419, #47705, #91979 ) ) ;
#94821=VERTEX_POINT ( 'NONE', #42270 ) ;
#94836=CARTESIAN_POINT ( 'NONE',  ( -103.8798399685330054, 1379.885066417289863, 304.5265232271229934 ) ) ;
#94837=CIRCLE ( 'NONE', #23276, 1.999997796872630351 ) ;
#94844=EDGE_LOOP ( 'NONE', ( #75936, #93843, #85061, #82306 ) ) ;
#94857=DIRECTION ( 'NONE',  ( -1.836970198721029688E-16, -1.000000000000000000, 0.000000000000000000 ) ) ;
#94860=CARTESIAN_POINT ( 'NONE',  ( -92.78054746879999470, 1385.201317530089909, 294.1545524748589742 ) ) ;
#94862=CIRCLE ( 'NONE', #85980, 11.26398391340000060 ) ;
#94872=CARTESIAN_POINT ( 'NONE',  ( -108.4852562064530161, 1383.359514468059842, 310.9366048184130022 ) ) ;
#94886=CARTESIAN_POINT ( 'NONE',  ( -109.0712831559999927, 1385.610640481809924, 297.1783689030590381 ) ) ;
#94926=CARTESIAN_POINT ( 'NONE',  ( -109.5441724319999963, 1376.146465230639933, 306.5935542917590055 ) ) ;
#94939=CARTESIAN_POINT ( 'NONE',  ( -7.989567273059999586, 1384.306348609750103, 199.5291464143689950 ) ) ;
#94959=EDGE_LOOP ( 'NONE', ( #43205, #28148, #53371, #3403 ) ) ;
#94960=CARTESIAN_POINT ( 'NONE',  ( -101.7780519309999931, 1379.485289779790037, 304.0160546798589962 ) ) ;
#94962=CARTESIAN_POINT ( 'NONE',  ( -107.1199205305639879, 1378.913060387299993, 301.0091205714350053 ) ) ;
#94966=CARTESIAN_POINT ( 'NONE',  ( -84.13119167140000343, 1384.814165098149942, 288.0554183306589948 ) ) ;
#94967=CARTESIAN_POINT ( 'NONE',  ( -59.87499638670439595, 1384.672222060019976, 243.7406793530619780 ) ) ;
#94979=CARTESIAN_POINT ( 'NONE',  ( -68.29164953469999944, 1379.747125763249869, 279.1059754382590086 ) ) ;
#94987=CARTESIAN_POINT ( 'NONE',  ( -38.49145949329999894, 1384.794605546870116, 239.3122526757589981 ) ) ;
#94990=CARTESIAN_POINT ( 'NONE',  ( -17.16993831374970014, 1385.286989672689742, 219.9424929166420100 ) ) ;
#95016=CARTESIAN_POINT ( 'NONE',  ( -4.145978979534980458E-15, 1375.413060387289988, 209.1218459572589836 ) ) ;
#95033=CARTESIAN_POINT ( 'NONE',  ( -95.12345330600079762, 1383.767095643290077, 309.8833154982480096 ) ) ;
#95042=CARTESIAN_POINT ( 'NONE',  ( -76.52635743460000128, 1382.336017472330013, 300.7162654001589885 ) ) ;
#95053=CARTESIAN_POINT ( 'NONE',  ( -109.9099220809999906, 1384.374201251870090, 297.0307877050590264 ) ) ;
#95082=ORIENTED_EDGE ( 'NONE', *, *, #3895, .T. ) ;
#95113=CARTESIAN_POINT ( 'NONE',  ( -11.66989614716730017, 1391.913060387289988, 209.6445408818580063 ) ) ;
#95126=CARTESIAN_POINT ( 'NONE',  ( -17.47467951480000181, 1385.286067972039973, 219.9356668727590147 ) ) ;
#95127=CARTESIAN_POINT ( 'NONE',  ( -4.145978979534980458E-15, 1375.413060387289988, 209.1218459572589836 ) ) ;
#95136=CARTESIAN_POINT ( 'NONE',  ( -9.700195692639999479, 1379.919833190730060, 216.8653063374690078 ) ) ;
#95143=CARTESIAN_POINT ( 'NONE',  ( -113.4000000000000057, 1391.913060387289988, 304.2218459572590064 ) ) ;
#95173=CARTESIAN_POINT ( 'NONE',  ( -6.280588687330000752, 1380.190335656839807, 203.2358530807489956 ) ) ;
#95180=CARTESIAN_POINT ( 'NONE',  ( -14.36267855726159937, 1380.304917481549865, 209.5901700444179880 ) ) ;
#95186=CARTESIAN_POINT ( 'NONE',  ( -82.75382724187160477, 1385.168106391910214, 286.4548433143800139 ) ) ;
#95187=CARTESIAN_POINT ( 'NONE',  ( -10.14901568273809929, 1391.913060387289988, 214.2247289053989903 ) ) ;
#95188=CARTESIAN_POINT ( 'NONE',  ( -59.96754922390000075, 1379.749011644449865, 261.8279529299589967 ) ) ;
#95225=CARTESIAN_POINT ( 'NONE',  ( -13.58429793331039903, 1379.610516642590028, 208.3569126637650015 ) ) ;
#95245=CARTESIAN_POINT ( 'NONE',  ( -12.54019908070000078, 1391.397792955739988, 209.7548876603800068 ) ) ;
#95246=CARTESIAN_POINT ( 'NONE',  ( -94.75128443427969671, 1384.856503445179897, 294.8510205860830524 ) ) ;
#95271=CARTESIAN_POINT ( 'NONE',  ( -68.62231159911313227, 1379.747791814526636, 280.2140134007494794 ) ) ;
#95285=CARTESIAN_POINT ( 'NONE',  ( -12.31752010984839885, 1377.944433743309901, 209.1218459601290078 ) ) ;
#95293=EDGE_CURVE ( 'NONE', #69449, #42195, #28270, .T. ) ;
#95303=CARTESIAN_POINT ( 'NONE',  ( -13.63528866819950025, 1379.581412608760047, 207.9504834338530088 ) ) ;
#95321=CARTESIAN_POINT ( 'NONE',  ( -65.68697704670019277, 1384.675462607609916, 289.6970332893050113 ) ) ;
#95322=CARTESIAN_POINT ( 'NONE',  ( -21.16387757469560071, 1384.952792652959943, 201.9777141633980193 ) ) ;
#95354=CARTESIAN_POINT ( 'NONE',  ( -66.34684761518089147, 1379.742662962009945, 277.0805805419040553 ) ) ;
#95362=CARTESIAN_POINT ( 'NONE',  ( -8.876070945589999539, 1385.242442397379818, 218.6685569028989846 ) ) ;
#95387=CARTESIAN_POINT ( 'NONE',  ( -55.54181829044275531, 1379.709133944529640, 251.3019363274339071 ) ) ;
#95410=EDGE_CURVE ( 'NONE', #29176, #77278, #47734, .T. ) ;
#95418=CARTESIAN_POINT ( 'NONE',  ( -89.15245910350000713, 1385.190331364289932, 292.2648985219589690 ) ) ;
#95456=CARTESIAN_POINT ( 'NONE',  ( -13.26473696127539981, 1384.881707513919991, 219.1240188487190039 ) ) ;
#95478=CARTESIAN_POINT ( 'NONE',  ( -101.5461033995489828, 1378.133454241549998, 306.5661732367119612 ) ) ;
#95506=CARTESIAN_POINT ( 'NONE',  ( -73.44525058019999619, 1378.783439397329857, 283.9849196026589766 ) ) ;
#95508=CARTESIAN_POINT ( 'NONE',  ( -106.2230645729750051, 1378.913060387289988, 302.3817510371559933 ) ) ;
#95514=CARTESIAN_POINT ( 'NONE',  ( -103.7369032989999909, 1385.230281736809957, 296.9336279125589613 ) ) ;
#95515=CARTESIAN_POINT ( 'NONE',  ( -59.63489001104600362, 1384.670753463339906, 243.2267383120320119 ) ) ;
#95526=CARTESIAN_POINT ( 'NONE',  ( -66.92355912140000385, 1379.746314988699851, 276.4200488462589647 ) ) ;
#95533=CARTESIAN_POINT ( 'NONE',  ( -109.2296128992090019, 1384.847618016620117, 295.1340898668969999 ) ) ;
#95535=CARTESIAN_POINT ( 'NONE',  ( -36.11164246829999769, 1384.804902789069956, 235.4725595070590032 ) ) ;
#95556=B_SPLINE_CURVE_WITH_KNOTS ( 'NONE', 3,
 ( #11952, #80264, #20884, #1352, #2484, #1924 ),
 .UNSPECIFIED., .F., .F.,
 ( 4, 2, 4 ),
 ( 0.000000000000000000, 0.5000000000000000000, 1.000000000000000000 ),
 .UNSPECIFIED. ) ;
#95583=CARTESIAN_POINT ( 'NONE',  ( -86.51864351971761380, 1383.772549446489847, 307.1887348928860320 ) ) ;
#95584=CARTESIAN_POINT ( 'NONE',  ( -109.0938415789800047, 1384.498162415240131, 311.2419644568369677 ) ) ;
#95590=CARTESIAN_POINT ( 'NONE',  ( -62.22036486049999837, 1383.793512663130059, 284.6761640327590044 ) ) ;
#95601=CARTESIAN_POINT ( 'NONE',  ( -108.8873841550000066, 1383.761288468090015, 297.2879149401589984 ) ) ;
#95654=ORIENTED_EDGE ( 'NONE', *, *, #50275, .F. ) ;
#95676=CARTESIAN_POINT ( 'NONE',  ( -1.130432680880949984E-15, 1385.340268378329938, 218.5931445290690078 ) ) ;
#95679=B_SPLINE_SURFACE_WITH_KNOTS ( 'NONE', 5, 5, ( 
 ( #95676, #10012, #8895, #77234, #43626, #44182, #43074, #535, #27363 ),
 ( #35212, #8341, #35771, #102946, #76118, #77774, #78320, #59339, #86168 ),
 ( #34659, #52586, #68843, #26248, #53139, #60436, #94554, #110814, #33534 ),
 ( #17827, #52032, #42505, #69954, #61545, #110258, #76665, #25136, #93449 ),
 ( #41964, #1086, #16719, #69398, #103509, #26812, #61000, #104068, #34107 ),
 ( #95126, #86719, #68298, #102406, #1634, #99931, #27922, #97323, #88380 ),
 ( #62104, #23225, #11136, #105184, #56300, #2199, #96228, #65266, #2748 ),
 ( #13709, #73667, #36868, #62669, #19505, #28476, #36313, #79979, #47895 ),
 ( #22101, #99376, #5335, #11670, #87277, #53709, #70510, #45296, #104625 ),
 ( #31632, #87848, #108351, #63216, #45846, #82603, #90986, #79436, #71062 ),
 ( #107798, #82031, #96790, #20060, #14274, #90431, #39495, #31083, #54254 ),
 ( #22651, #56855, #3298, #48465, #37429, #10571, #5893, #40039, #71626 ),
 ( #105747, #29031, #74222, #65813, #44743, #78893, #59068, #68573, #93191 ),
 ( #42804, #32741, #58511, #76399, #108901, #66921, #102676, #57425, #16460 ),
 ( #32191, #50654, #101030, #66376, #24328, #92641, #49563, #17003, #92095 ),
 ( #110553, #67472, #84243, #40591, #6987, #84785, #34400, #6445, #8629 ),
 ( #75320, #33839, #25417, #7541, #15915, #109462, #50114, #101577, #102139 ),
 ( #41696, #24865, #75855, #74762, #76964, #57962, #83692, #8083, #15374 ),
 ( #41141, #59612, #274, #110005, #33282, #91550, #23775, #42252, #68029 ),
 ( #100494, #93725, #51203, #14827, #85332, #49014, #83150, #17567, #18135 ),
 ( #1361, #817, #1933, #3042, #43368, #43912, #103815, #28208, #26545 ),
 ( #103233, #45592, #36070, #27115, #19799, #62397, #60738, #51767, #61299 ),
 ( #19226, #77516, #52332, #96522, #70255, #104362, #27659, #9746, #95418 ),
 ( #61846, #95965, #18681, #53433, #78056, #37168, #54003, #87580, #94860 ),
 ( #86455, #35503, #52879, #69696, #36609, #10868, #87007, #71364, #85901 ),
 ( #25972, #10296, #9208, #44472, #78617, #45041, #79186, #88135, #60171 ),
 ( #2492, #70810, #34945, #69130, #104923, #94289, #11423, #79733, #106569 ),
 ( #46146, #5772, #29307, #12512, #72977, #20345, #80276, #81904, #20892 ),
 ( #30403, #90302, #55090, #80822, #37714, #46691, #54549, #98158, #64594 ),
 ( #38802, #5209, #21973, #29855, #105476, #71916, #88683, #63506, #11960 ) ),
 .UNSPECIFIED., .F., .F., .F.,
 ( 6, 3, 3, 3, 3, 3, 3, 3, 3, 6 ),
 ( 6, 3, 6 ),
 ( 0.000000000000000000, 15.39383910899999997, 27.58084801740000103, 41.39509552349999666, 65.53909258059999843, 90.91108773649999364, 117.6367619669999982, 132.4493970709999928, 144.8160795070000120, 161.8240513320000105 ),
 ( 34.48604544350000367, 51.30231389200000081, 68.11858234059999972 ),
 .UNSPECIFIED. ) ;
#95683=CARTESIAN_POINT ( 'NONE',  ( -9.094129269030000629, 1384.954944735329946, 199.9429221374590213 ) ) ;
#95704=CARTESIAN_POINT ( 'NONE',  ( -106.0556725455072211, 1391.049867165201249, 307.0681147628054646 ) ) ;
#95712=CARTESIAN_POINT ( 'NONE',  ( -32.73835355732309438, 1383.838552529339950, 230.9115847139019877 ) ) ;
#95721=CARTESIAN_POINT ( 'NONE',  ( -5.504892848440839376E-16, 1382.319254473250112, 217.9325275017089893 ) ) ;
#95726=ORIENTED_EDGE ( 'NONE', *, *, #97295, .T. ) ;
#95728=CARTESIAN_POINT ( 'NONE',  ( -14.51787070936009805, 1379.822861006080075, 208.4144866268740088 ) ) ;
#95733=CARTESIAN_POINT ( 'NONE',  ( -12.31752010984839885, 1377.944433743309901, 209.1218459601290078 ) ) ;
#95735=CARTESIAN_POINT ( 'NONE',  ( -11.76014441919999953, 1391.665771868209958, 205.8582101077390121 ) ) ;
#95736=CARTESIAN_POINT ( 'NONE',  ( -96.75293248057811013, 1385.212375750189949, 295.5163800457769980 ) ) ;
#95773=CARTESIAN_POINT ( 'NONE',  ( -13.79573821373410070, 1379.664681114740006, 208.3123142327969788 ) ) ;
#95782=EDGE_LOOP ( 'NONE', ( #66408, #85574, #41081, #46505, #43887, #109713 ) ) ;
#95809=CARTESIAN_POINT ( 'NONE',  ( -109.8548145285198387, 1383.584493755403855, 297.0890030339772352 ) ) ;
#95811=CARTESIAN_POINT ( 'NONE',  ( -32.61735071319999690, 1379.648822273989936, 216.0058851815090009 ) ) ;
#95847=CARTESIAN_POINT ( 'NONE',  ( -14.43005995440260136, 1379.618177126189948, 208.1145997592700212 ) ) ;
#95855=CARTESIAN_POINT ( 'NONE',  ( -7.596271589240429556, 1384.058932579810062, 219.0207375155539751 ) ) ;
#95867=CARTESIAN_POINT ( 'NONE',  ( -69.80456196563160631, 1384.663061549279973, 294.8462645368060180 ) ) ;
#95868=CARTESIAN_POINT ( 'NONE',  ( -34.80461611804459920, 1384.978283401549788, 208.5676735308819900 ) ) ;
#95875=CARTESIAN_POINT ( 'NONE',  ( -7.966081152810000177, 1384.918389262350047, 199.4892680610689979 ) ) ;
#95902=CARTESIAN_POINT ( 'NONE',  ( -66.97548518297490716, 1379.744360727889898, 277.9508606322140167 ) ) ;
#95915=CARTESIAN_POINT ( 'NONE',  ( -105.8906218209530010, 1378.913060388219719, 304.9510362749820160 ) ) ;
#95932=CARTESIAN_POINT ( 'NONE',  ( -8.581228205849999568, 1384.934619283940037, 218.6696012310689810 ) ) ;
#95937=CARTESIAN_POINT ( 'NONE',  ( -38.67752440520889934, 1379.650603488850038, 221.7945647579082333 ) ) ;
#95948=CARTESIAN_POINT ( 'NONE',  ( -54.27566527714611766, 1379.707491775901872, 254.2935361429743466 ) ) ;
#95965=CARTESIAN_POINT ( 'NONE',  ( -86.94526474789999781, 1386.534739258749823, 307.6971543075589466 ) ) ;
#95977=CARTESIAN_POINT ( 'NONE',  ( -104.5971662677009988, 1379.798410771470117, 305.4970342620409838 ) ) ;
#96001=CARTESIAN_POINT ( 'NONE',  ( -20.42440048154189824, 1384.860985728550077, 221.1297803709319965 ) ) ;
#96022=CIRCLE ( 'NONE', #1329, 6.868727599660006788 ) ;
#96052=VERTEX_POINT ( 'NONE', #81941 ) ;
#96061=CARTESIAN_POINT ( 'NONE',  ( -78.35932141380000360, 1374.964007173050049, 291.3894706323590071 ) ) ;
#96076=CARTESIAN_POINT ( 'NONE',  ( -67.33401983280000991, 1379.744965387350021, 277.0816680017589988 ) ) ;
#96084=CARTESIAN_POINT ( 'NONE',  ( -62.06522312460000279, 1384.809685994470101, 284.7693067110590164 ) ) ;
#96085=VERTEX_POINT ( 'NONE', #5810 ) ;
#96096=CARTESIAN_POINT ( 'NONE',  ( -5.932239102140000497, 1391.913060387289988, 215.1144410137189880 ) ) ;
#96108=CARTESIAN_POINT ( 'NONE',  ( -109.1309839890330124, 1384.924126711810004, 311.2646841801559958 ) ) ;
#96133=CARTESIAN_POINT ( 'NONE',  ( -92.50840546082399385, 1383.768738235890169, 309.2665542712870206 ) ) ;
#96134=CARTESIAN_POINT ( 'NONE',  ( -109.5946542274029980, 1383.641284564509988, 311.2236547677540557 ) ) ;
#96140=CARTESIAN_POINT ( 'NONE',  ( -91.82171654609999223, 1380.714193802210048, 296.3822057022590002 ) ) ;
#96150=EDGE_CURVE ( 'NONE', #110163, #103208, #106702, .T. ) ;
#96168=COLOUR_RGB ( '', 0.66274510, 0.83137255, 0.94901961) ;
#96213=AXIS2_PLACEMENT_3D ( 'NONE', #53057, #87764, #51944 ) ;
#96218=CARTESIAN_POINT ( 'NONE',  ( -11.53051474154809952, 1391.913060387269979, 207.8395204436380084 ) ) ;
#96224=EDGE_LOOP ( 'NONE', ( #107475, #101007, #90930, #69762 ) ) ;
#96228=CARTESIAN_POINT ( 'NONE',  ( -25.50709298239999967, 1388.283930419619992, 204.4842806613090147 ) ) ;
#96237=CARTESIAN_POINT ( 'NONE',  ( -9.129868668039998525, 1382.253540356249914, 217.9228041959689790 ) ) ;
#96238=AXIS2_PLACEMENT_3D ( 'NONE', #100797, #92399, #35828 ) ;
#96245=AXIS2_PLACEMENT_3D ( 'NONE', #77804, #103542, #26846 ) ;
#96267=CARTESIAN_POINT ( 'NONE',  ( -36.25285754200669430, 1383.833716293010184, 235.7112261900410033 ) ) ;
#96275=CARTESIAN_POINT ( 'NONE',  ( -3.078458354199999913, 1382.920902153249926, 199.9060629954589956 ) ) ;
#96282=CARTESIAN_POINT ( 'NONE',  ( -14.41810545100110019, 1380.214461174779899, 209.1805091506649887 ) ) ;
#96290=CARTESIAN_POINT ( 'NONE',  ( -99.64099788066441477, 1385.219955568270052, 296.2123915739539939 ) ) ;
#96292=CARTESIAN_POINT ( 'NONE',  ( -44.12060424749999754, 1379.737242085850085, 229.5711980135589840 ) ) ;
#96295=EDGE_CURVE ( 'NONE', #55409, #69449, #82787, .T. ) ;
#96318=ORIENTED_EDGE ( 'NONE', *, *, #72188, .F. ) ;
#96364=CARTESIAN_POINT ( 'NONE',  ( -106.9747615859999996, 1387.585777271070128, 298.0968282848589865 ) ) ;
#96367=CARTESIAN_POINT ( 'NONE',  ( -16.46152824260000003, 1379.712491941360213, 208.5854493838049848 ) ) ;
#96371=CARTESIAN_POINT ( 'NONE',  ( -66.42203761248978822, 1379.747445253714659, 277.0326445464845619 ) ) ;
#96378=CARTESIAN_POINT ( 'NONE',  ( -71.67062476821969597, 1385.018456839120063, 296.8795409282479909 ) ) ;
#96408=CARTESIAN_POINT ( 'NONE',  ( -13.02155667789130078, 1379.339783279080166, 208.0032768703970021 ) ) ;
#96428=CARTESIAN_POINT ( 'NONE',  ( -97.79596852057099454, 1384.604925093459997, 310.5386097793889917 ) ) ;
#96429=CARTESIAN_POINT ( 'NONE',  ( -47.40790290358329884, 1385.010400382010175, 221.4590170555140105 ) ) ;
#96435=CARTESIAN_POINT ( 'NONE',  ( -5.013435694540000043, 1375.426148861440197, 214.7180213005390215 ) ) ;
#96436=CARTESIAN_POINT ( 'NONE',  ( -9.094817557369999861, 1384.935820800019883, 199.9428001500290293 ) ) ;
#96447=CARTESIAN_POINT ( 'NONE',  ( -11.38166339569999863, 1381.807649517150139, 201.7589817661390157 ) ) ;
#96459=CARTESIAN_POINT ( 'NONE',  ( -67.00076415430000054, 1379.747503662089912, 277.9341329109589651 ) ) ;
#96464=CARTESIAN_POINT ( 'NONE',  ( -8.861333410889999485, 1384.870662623839962, 218.6848950059789729 ) ) ;
#96471=CARTESIAN_POINT ( 'NONE',  ( -106.0957693905839960, 1378.913060388589884, 305.6009486211909802 ) ) ;
#96490=CARTESIAN_POINT ( 'NONE',  ( -49.24152454686350922, 1379.685811767087898, 238.1174555105647528 ) ) ;
#96502=CARTESIAN_POINT ( 'NONE',  ( -60.50191481579621922, 1379.727517218082312, 266.7693724609832202 ) ) ;
#96522=CARTESIAN_POINT ( 'NONE',  ( -82.65821105559999182, 1389.340475723369991, 302.6007231854590032 ) ) ;
#96525=AXIS2_PLACEMENT_3D ( 'NONE', #36233, #22012, #44650 ) ;
#96536=CARTESIAN_POINT ( 'NONE',  ( -105.9035083438030114, 1380.145576709830038, 307.7816103815599718 ) ) ;
#96537=ORIENTED_EDGE ( 'NONE', *, *, #4136, .T. ) ;
#96554=B_SPLINE_CURVE_WITH_KNOTS ( 'NONE', 3,
 ( #43760, #77912, #70647, #78466, #104212, #61686, #95809, #28049, #53280, #104764, #62239, #20733, #82313, #97999, #57136, #5049, #48175, #22371, #99092, #56020, #56571, #73924, #5611, #13427, #108053, #39194, #31349, #91263, #21269, #47617, #3981, #65533, #98552, #14542, #97464 ),
 .UNSPECIFIED., .F., .F.,
 ( 4, 2, 2, 1, 1, 1, 2, 2, 2, 2, 1, 1, 1, 2, 2, 2, 2, 1, 2, 2, 4 ),
 ( 0.000000000000000000, 0.1249999999977491338, 0.1874999999966215636, 0.2187499999960577646, 0.2343749999957791263, 0.2421874999956387942, 0.2460937499956126484, 0.2499999999955865304, 0.3749999999950853757, 0.4374999999947900009, 0.4687499999946407869, 0.4843749999946093676, 0.4921874999945921592, 0.4960937499945835549, 0.4999999999945750062, 0.6249999999958929520, 0.6874999999965575315, 0.7187499999968445241, 0.7343749999969880760, 0.7499999999971316278, 1.000000000000000000 ),
 .UNSPECIFIED. ) ;
#96564=CARTESIAN_POINT ( 'NONE',  ( -22.64763560905369744, 1384.853897193610010, 222.2275427940429893 ) ) ;
#96581=CARTESIAN_POINT ( 'NONE',  ( -12.58289157959999827, 1379.610106932609824, 209.8104170840169900 ) ) ;
#96588=CARTESIAN_POINT ( 'NONE',  ( -82.87519116838579691, 1378.248460717899889, 300.2215825002689940 ) ) ;
#96593=VERTEX_POINT ( 'NONE', #92404 ) ;
#96596=DIRECTION ( 'NONE',  ( 0.01668530547205149608, 0.7071067811868640973, -0.7069098956591685079 ) ) ;
#96598=CARTESIAN_POINT ( 'NONE',  ( -8.537909486209999343, 1383.668034227369844, 218.4909987399589966 ) ) ;
#96614=EDGE_CURVE ( 'NONE', #34413, #60257, #24442, .T. ) ;
#96622=CARTESIAN_POINT ( 'NONE',  ( -84.75344743939999148, 1374.600296256490083, 297.4377104198590018 ) ) ;
#96623=CARTESIAN_POINT ( 'NONE',  ( -106.3928623033740024, 1378.913060387289988, 302.0630715194479876 ) ) ;
#96628=CARTESIAN_POINT ( 'NONE',  ( -113.4000000000000057, 1385.251674955540238, 297.2379167808589955 ) ) ;
#96636=CARTESIAN_POINT ( 'NONE',  ( -17.46768317430000295, 1384.870099884450156, 219.9576826991589940 ) ) ;
#96642=CARTESIAN_POINT ( 'NONE',  ( -67.92939999230000581, 1379.746255314009886, 278.2862461588590008 ) ) ;
#96651=CARTESIAN_POINT ( 'NONE',  ( -54.13172275060000516, 1384.971233722779971, 270.3676613534589706 ) ) ;
#96654=CARTESIAN_POINT ( 'NONE',  ( -22.28602175699319687, 1385.267146508269889, 222.0073600989599925 ) ) ;
#96676=DIRECTION ( 'NONE',  ( -1.836970198721029688E-16, -1.000000000000000000, -8.835242138475329394E-33 ) ) ;
#96701=CARTESIAN_POINT ( 'NONE',  ( -80.60779555424529974, 1383.776547664450163, 304.0453241665860560 ) ) ;
#96702=CARTESIAN_POINT ( 'NONE',  ( -108.9251951694480027, 1383.742096774909896, 311.0727769249569974 ) ) ;
#96708=CARTESIAN_POINT ( 'NONE',  ( -92.45138929590000032, 1381.911264019279770, 294.9202873905589968 ) ) ;
#96713=CARTESIAN_POINT ( 'NONE',  ( -109.3493624629999914, 1384.903260851859841, 297.1385571428590424 ) ) ;
#96718=CARTESIAN_POINT ( 'NONE',  ( -109.6260819770000126, 1384.887353564230125, 297.0994507507589901 ) ) ;
#96759=EDGE_CURVE ( 'NONE', #78937, #46370, #101398, .T. ) ;
#96790=CARTESIAN_POINT ( 'NONE',  ( -33.19360111489999809, 1388.470894590589978, 229.1017553306589889 ) ) ;
#96795=CARTESIAN_POINT ( 'NONE',  ( -14.04885618097836897, 1379.586891663671850, 211.8295121144176676 ) ) ;
#96798=CARTESIAN_POINT ( 'NONE',  ( -11.39126005979999867, 1381.496251003520001, 216.9356158229890070 ) ) ;
#96812=CARTESIAN_POINT ( 'NONE',  ( -12.31211413366879981, 1378.375898250180171, 209.7639663314890015 ) ) ;
#96830=CARTESIAN_POINT ( 'NONE',  ( -21.32959704448400018, 1383.852165897360010, 221.3536186575369982 ) ) ;
#96837=ORIENTED_EDGE ( 'NONE', *, *, #61205, .T. ) ;
#96840=CARTESIAN_POINT ( 'NONE',  ( -6.349985216170000335, 1382.931437671549929, 199.9495528202790240 ) ) ;
#96847=CARTESIAN_POINT ( 'NONE',  ( -8.974550634399999893, 1388.636165673550295, 217.7040576462889874 ) ) ;
#96854=CARTESIAN_POINT ( 'NONE',  ( -7.966093458541450012, 1384.918002514549926, 199.4892729902699955 ) ) ;
#96855=CARTESIAN_POINT ( 'NONE',  ( -95.36803178986139073, 1385.208579419249872, 295.0786609535289813 ) ) ;
#96857=CARTESIAN_POINT ( 'NONE',  ( -41.85969401239999854, 1379.735023715520128, 226.1594769080589913 ) ) ;
#96876=CARTESIAN_POINT ( 'NONE',  ( -107.0843635519999992, 1382.329134876569924, 298.0462323021590691 ) ) ;
#96905=CARTESIAN_POINT ( 'NONE',  ( -12.28448271699999950, 1391.742831493179892, 209.7423336216829739 ) ) ;
#96907=ORIENTED_EDGE ( 'NONE', *, *, #101266, .T. ) ;
#96917=EDGE_CURVE ( 'NONE', #105177, #60257, #13811, .T. ) ;
#96937=CARTESIAN_POINT ( 'NONE',  ( -61.62696079022420292, 1385.058290879319884, 283.6552644066600237 ) ) ;
#96948=CARTESIAN_POINT ( 'NONE',  ( -12.35978978633600001, 1391.723785652940933, 209.7460346078842974 ) ) ;
#96964=FACE_OUTER_BOUND ( 'NONE', #28837, .T. ) ;
#96972=CARTESIAN_POINT ( 'NONE',  ( -7.548201923578629291, 1384.559186287549892, 219.0738854171599996 ) ) ;
#96980=CARTESIAN_POINT ( 'NONE',  ( -1.836970198721029983E-15, 1374.913060387289988, 209.1218459572589836 ) ) ;
#96987=CARTESIAN_POINT ( 'NONE',  ( -105.8373447700190013, 1384.589731091189833, 311.2092883949439965 ) ) ;
#96988=CARTESIAN_POINT ( 'NONE',  ( -49.08829210262739906, 1385.015916341950060, 223.8650612806140145 ) ) ;
#96989=CARTESIAN_POINT ( 'NONE',  ( -5.101748558636990616, 1375.122757580649932, 214.7573637342229915 ) ) ;
#96995=ORIENTED_EDGE ( 'NONE', *, *, #56962, .T. ) ;
#97006=CARTESIAN_POINT ( 'NONE',  ( -11.99335295539999890, 1380.187651171090010, 204.2174947147890123 ) ) ;
#97019=CARTESIAN_POINT ( 'NONE',  ( -68.31098214269999858, 1379.747686652819993, 279.8373429270589554 ) ) ;
#97025=CARTESIAN_POINT ( 'NONE',  ( -109.4842782119999924, 1384.933317133270066, 311.2840723172590174 ) ) ;
#97047=CARTESIAN_POINT ( 'NONE',  ( -7.545183853529999318, 1384.918586394910108, 219.0875716720989885 ) ) ;
#97049=CARTESIAN_POINT ( 'NONE',  ( -14.52404855940000061, 1379.696583046410069, 208.2610545982349777 ) ) ;
#97050=CARTESIAN_POINT ( 'NONE',  ( -67.62931585915434596, 1379.745611060300917, 277.6776758072804228 ) ) ;
#97061=CARTESIAN_POINT ( 'NONE',  ( -46.83417551517494104, 1379.681032646411495, 239.8460456441436293 ) ) ;
#97063=FACE_OUTER_BOUND ( 'NONE', #108044, .T. ) ;
#97091=CARTESIAN_POINT ( 'NONE',  ( -106.9481960069999928, 1379.492203629369897, 308.7579988892589995 ) ) ;
#97101=CARTESIAN_POINT ( 'NONE',  ( -106.3976693117229928, 1390.939243848519936, 307.7527733253859878 ) ) ;
#97113=CARTESIAN_POINT ( 'NONE',  ( -38.50602658467759909, 1384.794211068249979, 239.5861974842979976 ) ) ;
#97129=CARTESIAN_POINT ( 'NONE',  ( -109.9838524239499975, 1384.633113356680042, 311.4476818303249388 ) ) ;
#97134=CARTESIAN_POINT ( 'NONE',  ( -49.29737642897650574, 1380.010108409559962, 242.9177998910799658 ) ) ;
#97144=CARTESIAN_POINT ( 'NONE',  ( -8.296394296239999022, 1384.634392827019838, 218.6956713340389911 ) ) ;
#97164=CARTESIAN_POINT ( 'NONE',  ( -94.75917113079999865, 1374.839168173989947, 301.3391293692590125 ) ) ;
#97174=CARTESIAN_POINT ( 'NONE',  ( -5.962417602059999489, 1383.866448007470126, 218.3533362890090075 ) ) ;
#97178=CARTESIAN_POINT ( 'NONE',  ( -67.98666868309999245, 1379.746563024860052, 278.4884602742590118 ) ) ;
#97186=CARTESIAN_POINT ( 'NONE',  ( -113.4000000000000057, 1384.800102265719943, 311.2218459572590064 ) ) ;
#97188=CARTESIAN_POINT ( 'NONE',  ( -37.35614046057779802, 1385.196686404090087, 237.6971322074060140 ) ) ;
#97197=CARTESIAN_POINT ( 'NONE',  ( -5.444242866291760130, 1391.534755755089918, 214.9072828329470042 ) ) ;
#97224=EDGE_CURVE ( 'NONE', #51642, #88625, #108626, .T. ) ;
#97234=CARTESIAN_POINT ( 'NONE',  ( -89.28949325252699509, 1383.770769996720219, 308.2764280168249797 ) ) ;
#97235=CARTESIAN_POINT ( 'NONE',  ( -108.8493753602240020, 1383.998071234949975, 311.1481355889490032 ) ) ;
#97239=CARTESIAN_POINT ( 'NONE',  ( -113.4000000000000057, 1383.754957750760013, 311.0314894602589675 ) ) ;
#97244=CARTESIAN_POINT ( 'NONE',  ( -109.5348967119999912, 1384.904918197099732, 297.1231116118590307 ) ) ;
#97295=EDGE_CURVE ( 'NONE', #50191, #19741, #49581, .T. ) ;
#97319=ORIENTED_EDGE ( 'NONE', *, *, #24086, .F. ) ;
#97323=CARTESIAN_POINT ( 'NONE',  ( -22.99718798410000176, 1386.621894033409944, 202.4024127538190214 ) ) ;
#97347=CARTESIAN_POINT ( 'NONE',  ( -109.3493290679999888, 1385.139709706009853, 297.1446333424589739 ) ) ;
#97349=ORIENTED_EDGE ( 'NONE', *, *, #20045, .T. ) ;
#97360=CARTESIAN_POINT ( 'NONE',  ( -18.70316107891150281, 1383.854929796499846, 220.2675684361349795 ) ) ;
#97369=CARTESIAN_POINT ( 'NONE',  ( -5.962417602059999489, 1383.866448007470126, 218.3533362890090075 ) ) ;
#97376=CARTESIAN_POINT ( 'NONE',  ( -10.45628814230000181, 1390.721297460369897, 215.7199839781590072 ) ) ;
#97385=CARTESIAN_POINT ( 'NONE',  ( -106.7907400783429921, 1385.237181466299944, 297.0459356838589997 ) ) ;
#97392=EDGE_CURVE ( 'NONE', #101083, #96593, #59915, .T. ) ;
#97407=DIRECTION ( 'NONE',  ( 0.003563285688556391394, -0.9999913849417920719, 0.002129093069402243805 ) ) ;
#97464=CARTESIAN_POINT ( 'NONE',  ( -107.4477384240240099, 1379.886883745280102, 299.0757736425410371 ) ) ;
#97468=CARTESIAN_POINT ( 'NONE',  ( -106.4065864580110059, 1391.913060387289988, 304.8084661972009712 ) ) ;
#97469=CARTESIAN_POINT ( 'NONE',  ( -14.08142637225379978, 1379.709117121690042, 211.5303641152310092 ) ) ;
#97475=CARTESIAN_POINT ( 'NONE',  ( -105.2149124839869927, 1384.933864520869975, 311.2011526427629633 ) ) ;
#97478=FACE_OUTER_BOUND ( 'NONE', #3995, .T. ) ;
#97525=CARTESIAN_POINT ( 'NONE',  ( -33.29420051208550291, 1384.975192605860002, 207.5272639334069993 ) ) ;
#97545=CARTESIAN_POINT ( 'NONE',  ( -11.58399188110000111, 1381.166830487859897, 202.6872540392290318 ) ) ;
#97546=CARTESIAN_POINT ( 'NONE',  ( -9.129808743239919977, 1383.863787745319996, 218.5279288296370055 ) ) ;
#97557=CARTESIAN_POINT ( 'NONE',  ( -68.19307365539999921, 1379.747659725539961, 279.6816280294590342 ) ) ;
#97565=CARTESIAN_POINT ( 'NONE',  ( -109.6576905139999951, 1384.926051320400120, 311.3230246392589606 ) ) ;
#97586=CARTESIAN_POINT ( 'NONE',  ( -7.769235937790000435, 1384.905328562600062, 218.9178834932589837 ) ) ;
#97590=CARTESIAN_POINT ( 'NONE',  ( -66.35921308805916397, 1379.742723719715968, 275.1101220287822002 ) ) ;
#97595=CARTESIAN_POINT ( 'NONE',  ( -49.72680530535440369, 1384.618443061529888, 224.8565442374369923 ) ) ;
#97635=CARTESIAN_POINT ( 'NONE',  ( -106.6524542679999854, 1380.137974075159946, 308.5605864792590296 ) ) ;
#97648=CARTESIAN_POINT ( 'NONE',  ( -105.6997850770000014, 1391.688872221259999, 304.2060384943581539 ) ) ;
#97658=CARTESIAN_POINT ( 'NONE',  ( -30.50452582731020001, 1384.826580460149898, 228.5933960381599945 ) ) ;
#97659=CARTESIAN_POINT ( 'NONE',  ( -105.0581544420000029, 1379.236406965169863, 304.0328518213589746 ) ) ;
#97679=CARTESIAN_POINT ( 'NONE',  ( -42.14410030795320239, 1378.731951168329942, 233.4973399294630099 ) ) ;
#97681=CARTESIAN_POINT ( 'NONE',  ( -16.62685139801940082, 1379.596349548939997, 212.3140244300689972 ) ) ;
#97689=CARTESIAN_POINT ( 'NONE',  ( -8.576277482710001010, 1384.765141178520025, 218.6682590137189948 ) ) ;
#97709=CARTESIAN_POINT ( 'NONE',  ( -12.31045031087770170, 1378.376187938819839, 209.7947225889870140 ) ) ;
#97711=EDGE_LOOP ( 'NONE', ( #51966, #61398, #78866, #89596, #1797 ) ) ;
#97713=CARTESIAN_POINT ( 'NONE',  ( -71.10329879200000391, 1377.246858117049896, 279.1099741719589815 ) ) ;
#97719=CARTESIAN_POINT ( 'NONE',  ( -89.15684587290000707, 1384.835666735910081, 292.2581851215589950 ) ) ;
#97726=CARTESIAN_POINT ( 'NONE',  ( -1.332267629549999902E-15, 1384.913060387289988, 218.6218459572590120 ) ) ;
#97730=CARTESIAN_POINT ( 'NONE',  ( -67.27445496530000923, 1379.746684743910009, 277.1113995282589713 ) ) ;
#97740=CARTESIAN_POINT ( 'NONE',  ( -81.18324780579999356, 1384.635789063720040, 304.9525423562590163 ) ) ;
#97742=CARTESIAN_POINT ( 'NONE',  ( -29.66846558571840120, 1385.235115920719863, 227.6884932317539949 ) ) ;
#97765=CARTESIAN_POINT ( 'NONE',  ( -105.3795303980000000, 1390.980575111779899, 304.2016934099590344 ) ) ;
#97781=CARTESIAN_POINT ( 'NONE',  ( -109.3135390088490055, 1383.527569083439857, 311.1030218576129869 ) ) ;
#97786=CARTESIAN_POINT ( 'NONE',  ( -102.8679838510000053, 1381.036522549190067, 309.3638378892590026 ) ) ;
#97791=CARTESIAN_POINT ( 'NONE',  ( -109.1645137389999860, 1384.901512809399946, 297.1326343689589748 ) ) ;
#97835=CARTESIAN_POINT ( 'NONE',  ( -26.91388312470140320, 1384.548951572099895, 204.0772839077369838 ) ) ;
#97885=CARTESIAN_POINT ( 'NONE',  ( -12.31445988513510059, 1378.367058764619969, 209.7118765406739840 ) ) ;
#97889=CARTESIAN_POINT ( 'NONE',  ( -109.1450418849999835, 1385.242479476409926, 297.1468690488589459 ) ) ;
#97900=CARTESIAN_POINT ( 'NONE',  ( -30.66717156608859796, 1383.841235968630144, 228.5150949522549979 ) ) ;
#97908=CARTESIAN_POINT ( 'NONE',  ( -18.79955029639999964, 1379.850043559990127, 215.7272756679390113 ) ) ;
#97917=CARTESIAN_POINT ( 'NONE',  ( -11.82541222281230020, 1389.477605041999823, 215.1362464586540000 ) ) ;
#97918=CARTESIAN_POINT ( 'NONE',  ( -10.67458942334280003, 1390.939239166159950, 215.3172498179779666 ) ) ;
#97927=CARTESIAN_POINT ( 'NONE',  ( -97.82861174526568959, 1385.215246727240128, 295.8056424823309953 ) ) ;
#97929=CARTESIAN_POINT ( 'NONE',  ( -68.11985932390000187, 1379.748509173530010, 278.8066904925590279 ) ) ;
#97948=CARTESIAN_POINT ( 'NONE',  ( -8.297448664060000922, 1384.938007622469968, 218.7034657859290121 ) ) ;
#97969=AXIS2_PLACEMENT_3D ( 'NONE', #28099, #27005, #62289 ) ;
#97999=CARTESIAN_POINT ( 'NONE',  ( -109.5833881897985265, 1382.919105250094844, 297.2490322646984851 ) ) ;
#98003=CARTESIAN_POINT ( 'NONE',  ( -105.6997970149250108, 1391.688863015299830, 304.2060425153250094 ) ) ;
#98004=CARTESIAN_POINT ( 'NONE',  ( -64.37783753527037334, 1379.747207013340358, 273.6112401814819464 ) ) ;
#98011=CARTESIAN_POINT ( 'NONE',  ( -87.22070388642269734, 1384.976040036309996, 307.6860165158650489 ) ) ;
#98017=EDGE_CURVE ( 'NONE', #50916, #96052, #1301, .T. ) ;
#98025=DIRECTION ( 'NONE',  ( 6.332794898383918850E-17, 1.000000000000000000, -8.716344404180429969E-17 ) ) ;
#98061=CARTESIAN_POINT ( 'NONE',  ( -95.07784190500939303, 1384.609914070380000, 310.0516348293959936 ) ) ;
#98063=CARTESIAN_POINT ( 'NONE',  ( -38.54599120904159548, 1384.986460508979917, 211.5487390164689998 ) ) ;
#98071=CARTESIAN_POINT ( 'NONE',  ( -109.1308573929999852, 1384.902467940340102, 311.2647317742590189 ) ) ;
#98072=AXIS2_PLACEMENT_3D ( 'NONE', #94003, #530, #59334 ) ;
#98082=CARTESIAN_POINT ( 'NONE',  ( -10.57226022420000078, 1380.120851655610068, 202.6664852126289986 ) ) ;
#98089=AXIS2_PLACEMENT_3D ( 'NONE', #12595, #55725, #20420 ) ;
#98092=CARTESIAN_POINT ( 'NONE',  ( -67.32292340012330101, 1379.744822991889805, 278.5476412461240443 ) ) ;
#98104=CARTESIAN_POINT ( 'NONE',  ( -105.8385759250460012, 1378.913060387480073, 304.6883937350420410 ) ) ;
#98120=CARTESIAN_POINT ( 'NONE',  ( -8.862056491009999704, 1384.892951007250076, 218.6851137842390074 ) ) ;
#98122=CARTESIAN_POINT ( 'NONE',  ( -66.20869285293976247, 1379.742364948664090, 274.8035288233667188 ) ) ;
#98126=CARTESIAN_POINT ( 'NONE',  ( -54.61776087596129514, 1384.642101012380181, 233.1560539664220073 ) ) ;
#98137=CARTESIAN_POINT ( 'NONE',  ( -108.7912805756727721, 1383.917190576337134, 311.1259201896712057 ) ) ;
#98158=CARTESIAN_POINT ( 'NONE',  ( -109.9987473170000101, 1386.781127266330031, 297.3270903142590100 ) ) ;
#98160=CARTESIAN_POINT ( 'NONE',  ( -8.156690520060001504, 1384.906090458550125, 199.6468865885190098 ) ) ;
#98198=CARTESIAN_POINT ( 'NONE',  ( -29.65001300571809750, 1384.829734561930081, 227.6949194770519966 ) ) ;
#98202=CARTESIAN_POINT ( 'NONE',  ( -105.8429516820000060, 1379.429574992919925, 301.1876983431590133 ) ) ;
#98223=CARTESIAN_POINT ( 'NONE',  ( -75.18978754212498927, 1377.263627487500116, 294.2967627425929891 ) ) ;
#98230=CARTESIAN_POINT ( 'NONE',  ( -113.4000000000000057, 1379.013060387289897, 304.2218459572590064 ) ) ;
#98235=CARTESIAN_POINT ( 'NONE',  ( -8.913847076610000641, 1384.359708517599984, 218.6448320083890167 ) ) ;
#98257=CARTESIAN_POINT ( 'NONE',  ( -14.36827873795669852, 1380.307879667200041, 209.5510879081830069 ) ) ;
#98261=CARTESIAN_POINT ( 'NONE',  ( -44.99452937619999915, 1380.083786706710043, 231.7591686846589880 ) ) ;
#98273=CARTESIAN_POINT ( 'NONE',  ( -25.93734973360000140, 1384.843007074499837, 224.2459728783589981 ) ) ;
#98277=CARTESIAN_POINT ( 'NONE',  ( -62.13174705850000379, 1379.729651049759923, 266.3263280308589742 ) ) ;
#98283=CARTESIAN_POINT ( 'NONE',  ( -106.5645047596862156, 1391.196592043153487, 300.3916496599600237 ) ) ;
#98285=CARTESIAN_POINT ( 'NONE',  ( -81.17851594969998530, 1384.753895121710002, 304.9599978423589732 ) ) ;
#98287=CARTESIAN_POINT ( 'NONE',  ( -26.70710024954369999, 1385.248442757040038, 224.9715981382639995 ) ) ;
#98292=CARTESIAN_POINT ( 'NONE',  ( -9.094755087212869071, 1384.939018560090062, 199.9428094726760037 ) ) ;
#98314=CARTESIAN_POINT ( 'NONE',  ( -105.5650123339999880, 1390.851006877979898, 302.0524783112590512 ) ) ;
#98316=CARTESIAN_POINT ( 'NONE',  ( -106.2614451870000067, 1391.913060386500092, 302.8078771165589842 ) ) ;
#98341=CARTESIAN_POINT ( 'NONE',  ( -102.7498137299999996, 1383.762281939259992, 311.0461218402589907 ) ) ;
#98346=CARTESIAN_POINT ( 'NONE',  ( -109.1643701970000109, 1384.923480540200217, 297.1325780693589991 ) ) ;
#98347=CARTESIAN_POINT ( 'NONE',  ( -9.013032691016070075, 1381.609887807723226, 200.5860147506873545 ) ) ;
#98359=DIRECTION ( 'NONE',  ( -6.162707975952100561E-15, -1.000000000000000000, -1.094450614310000083E-14 ) ) ;
#98363=EDGE_LOOP ( 'NONE', ( #51032, #98797, #80638, #99774, #3000 ) ) ;
#98394=CARTESIAN_POINT ( 'NONE',  ( -13.08406847753679969, 1384.517833128000120, 200.3646909337909960 ) ) ;
#98400=ORIENTED_EDGE ( 'NONE', *, *, #17950, .F. ) ;
#98458=CARTESIAN_POINT ( 'NONE',  ( -40.29337211549999864, 1383.827701909899815, 242.2979617791790190 ) ) ;
#98466=CARTESIAN_POINT ( 'NONE',  ( -18.10779123049999839, 1380.896120499720155, 217.9240877703190051 ) ) ;
#98473=CARTESIAN_POINT ( 'NONE',  ( -10.52351523589999971, 1390.477550767929870, 215.6246750091789863 ) ) ;
#98481=CARTESIAN_POINT ( 'NONE',  ( -7.966157931650249324, 1384.915561067150065, 199.4892992289589984 ) ) ;
#98496=CARTESIAN_POINT ( 'NONE',  ( -109.0318845759999959, 1385.766567570789903, 311.1758076612590003 ) ) ;
#98505=CARTESIAN_POINT ( 'NONE',  ( -8.582794586710001283, 1385.145244622950031, 218.6615206947490151 ) ) ;
#98528=CARTESIAN_POINT ( 'NONE',  ( -9.853100102660000914, 1384.791813251800022, 199.8713787141489888 ) ) ;
#98535=VERTEX_POINT ( 'NONE', #27578 ) ;
#98540=TOROIDAL_SURFACE ( 'NONE', #80653, 11.34254167809999991, 1.000000000000000000 ) ;
#98552=CARTESIAN_POINT ( 'NONE',  ( -107.9782425448296266, 1380.517964044677910, 298.4850064908227409 ) ) ;
#98556=CARTESIAN_POINT ( 'NONE',  ( -105.8303611032980029, 1391.403921100310072, 306.3485471784230185 ) ) ;
#98564=CARTESIAN_POINT ( 'NONE',  ( -85.22981105258379841, 1384.980801281210006, 306.8062713692789885 ) ) ;
#98565=CARTESIAN_POINT ( 'NONE',  ( -8.840249975039998986, 1385.811718649069917, 199.9964793815190092 ) ) ;
#98580=CARTESIAN_POINT ( 'NONE',  ( -106.5585968837300044, 1390.939245634569943, 300.3884029622149683 ) ) ;
#98593=B_SPLINE_CURVE_WITH_KNOTS ( 'NONE', 5,
 ( #995, #52496, #17735, #51937, #33446, #102857 ),
 .UNSPECIFIED., .F., .F.,
 ( 6, 6 ),
 ( 0.000000000000000000, 1.000000000000000000 ),
 .UNSPECIFIED. ) ;
#98612=CARTESIAN_POINT ( 'NONE',  ( -12.29932871299999952, 1378.340749811539808, 209.9617947631720085 ) ) ;
#98613=CARTESIAN_POINT ( 'NONE',  ( -88.01709926131411521, 1384.622882125699789, 307.9926968129980196 ) ) ;
#98614=CARTESIAN_POINT ( 'NONE',  ( -62.52713540591220465, 1385.073953399070206, 249.5246976450929992 ) ) ;
#98621=CARTESIAN_POINT ( 'NONE',  ( -109.9848792289999864, 1384.913535650479844, 311.4560967522589863 ) ) ;
#98631=CARTESIAN_POINT ( 'NONE',  ( -11.34339085279999892, 1379.280816169740092, 204.1266110777590086 ) ) ;
#98640=ORIENTED_EDGE ( 'NONE', *, *, #5552, .F. ) ;
#98643=CARTESIAN_POINT ( 'NONE',  ( -68.04155215168790960, 1379.746364830730045, 279.5506397144160360 ) ) ;
#98677=CARTESIAN_POINT ( 'NONE',  ( -13.83705309760000191, 1379.709095927359840, 208.1765788499700136 ) ) ;
#98678=CARTESIAN_POINT ( 'NONE',  ( -68.77278092737650184, 1379.747928288920093, 280.3133413970129482 ) ) ;
#98683=CARTESIAN_POINT ( 'NONE',  ( -61.94336356843140123, 1384.685152223810064, 248.2490218926199930 ) ) ;
#98688=ORIENTED_EDGE ( 'NONE', *, *, #25438, .F. ) ;
#98750=CARTESIAN_POINT ( 'NONE',  ( -42.07899341319999564, 1384.778030063439928, 245.8949318473310086 ) ) ;
#98775=CARTESIAN_POINT ( 'NONE',  ( -82.80618832229581017, 1377.207454081310289, 300.3238556022119496 ) ) ;
#98778=ORIENTED_EDGE ( 'NONE', *, *, #27920, .F. ) ;
#98784=ADVANCED_FACE ( 'NONE', ( #5554 ), #56460, .F. ) ;
#98787=CARTESIAN_POINT ( 'NONE',  ( -8.251661180240001059, 1383.545955608860140, 218.5607180263089901 ) ) ;
#98790=ADVANCED_FACE ( 'NONE', ( #64669 ), #39474, .T. ) ;
#98797=ORIENTED_EDGE ( 'NONE', *, *, #62066, .F. ) ;
#98805=CARTESIAN_POINT ( 'NONE',  ( -109.9823850403438712, 1385.269780471392323, 311.4448117272161198 ) ) ;
#98808=CARTESIAN_POINT ( 'NONE',  ( -12.31216202546280059, 1378.376212517099930, 209.7634181235169706 ) ) ;
#98813=CARTESIAN_POINT ( 'NONE',  ( -42.05438492420000074, 1375.117442312619914, 227.1521432528590196 ) ) ;
#98827=CARTESIAN_POINT ( 'NONE',  ( -49.65271057950000255, 1384.118016094159884, 260.8803987871590380 ) ) ;
#98832=CARTESIAN_POINT ( 'NONE',  ( -62.83880642449999954, 1379.741026228560031, 268.0244666111590277 ) ) ;
#98840=CARTESIAN_POINT ( 'NONE',  ( -106.4193208100000021, 1384.931129459059775, 311.3263713972589812 ) ) ;
#98842=CARTESIAN_POINT ( 'NONE',  ( -33.46600142563520563, 1385.216900170149984, 232.0947013295109969 ) ) ;
#98866=CARTESIAN_POINT ( 'NONE',  ( -106.5486053249999969, 1387.898087395329867, 298.3709353731589999 ) ) ;
#98868=CARTESIAN_POINT ( 'NONE',  ( -105.6997850770000014, 1391.688872221259999, 304.2060384943590066 ) ) ;
#98872=CARTESIAN_POINT ( 'NONE',  ( -105.6135012430000018, 1378.264671279439881, 303.3196108302589664 ) ) ;
#98883=CARTESIAN_POINT ( 'NONE',  ( -104.5883840766809953, 1383.761025698020148, 310.9908609358749914 ) ) ;
#98888=CARTESIAN_POINT ( 'NONE',  ( -109.9987472910000008, 1380.124979902150017, 307.5701647321589576 ) ) ;
#98894=CARTESIAN_POINT ( 'NONE',  ( -8.164798220873796808, 1383.354011203070968, 199.7069691412050076 ) ) ;
#98910=EDGE_LOOP ( 'NONE', ( #103073, #92220, #101806, #33582, #89, #11424, #44174, #90280 ) ) ;
#98987=CARTESIAN_POINT ( 'NONE',  ( -109.8956297860000006, 1384.931289663850066, 297.0283806398589945 ) ) ;
#98998=CARTESIAN_POINT ( 'NONE',  ( -50.19710983959630113, 1383.811588252980073, 261.7494256533389603 ) ) ;
#99007=CARTESIAN_POINT ( 'NONE',  ( -38.90243383290000168, 1381.518824974109975, 213.3883314898789934 ) ) ;
#99013=CARTESIAN_POINT ( 'NONE',  ( -9.214005947760000481, 1389.265557518159994, 217.4246417548390014 ) ) ;
#99019=CARTESIAN_POINT ( 'NONE',  ( -104.7943799579999933, 1379.906422268759798, 301.8989113051590039 ) ) ;
#99026=CARTESIAN_POINT ( 'NONE',  ( -68.62428177750000202, 1379.748209670530059, 279.8484656398590005 ) ) ;
#99028=DIRECTION ( 'NONE',  ( 0.2420316379589268763, -4.446049060781863124E-17, 0.9702683578407156340 ) ) ;
#99031=CARTESIAN_POINT ( 'NONE',  ( -109.1642343328397260, 1384.919851393370436, 297.1325477198193425 ) ) ;
#99037=CARTESIAN_POINT ( 'NONE',  ( -109.2142229400000133, 1387.165659784040145, 310.9727364242590397 ) ) ;
#99046=CARTESIAN_POINT ( 'NONE',  ( -8.589998329009999267, 1385.225457215250117, 218.6546645165990128 ) ) ;
#99050=EDGE_CURVE ( 'NONE', #23316, #82812, #85427, .T. ) ;
#99062=CARTESIAN_POINT ( 'NONE',  ( -108.1236415588580115, 1378.913060387289988, 299.8223284637080610 ) ) ;
#99081=ORIENTED_EDGE ( 'NONE', *, *, #7673, .F. ) ;
#99092=CARTESIAN_POINT ( 'NONE',  ( -109.1299347229319210, 1382.116777868800455, 297.5434349749086778 ) ) ;
#99097=CARTESIAN_POINT ( 'NONE',  ( -106.5186017514349999, 1391.553736368970021, 307.6918517192190166 ) ) ;
#99105=CARTESIAN_POINT ( 'NONE',  ( -79.55893548068129917, 1384.995123410919859, 303.5731928006850353 ) ) ;
#99107=CARTESIAN_POINT ( 'NONE',  ( -8.998777790820000178, 1385.475401132710203, 199.9682204879490257 ) ) ;
#99112=CARTESIAN_POINT ( 'NONE',  ( -7.544733521240000407, 1384.899971913130003, 219.0877090842990071 ) ) ;
#99142=CARTESIAN_POINT ( 'NONE',  ( -103.7837470130642856, 1380.040681755203195, 305.7727476933569051 ) ) ;
#99150=CARTESIAN_POINT ( 'NONE',  ( -57.51883745420190053, 1385.049604656559950, 238.7888358578429973 ) ) ;
#99157=CARTESIAN_POINT ( 'NONE',  ( -109.3073322039999908, 1384.904126850409966, 311.2647055142589920 ) ) ;
#99160=CARTESIAN_POINT ( 'NONE',  ( -109.9871902949999907, 1384.855229205870046, 311.4556902802589775 ) ) ;
#99174=CARTESIAN_POINT ( 'NONE',  ( -5.099447121353800405, 1375.125474032349985, 203.4873467743369986 ) ) ;
#99182=CARTESIAN_POINT ( 'NONE',  ( -68.44821854895280921, 1379.747450488880077, 280.0214965132619795 ) ) ;
#99185=CARTESIAN_POINT ( 'NONE',  ( -11.01457153678066980, 1378.540399413372143, 214.6712006714588199 ) ) ;
#99210=CARTESIAN_POINT ( 'NONE',  ( -67.63660556605692875, 1379.745626871633021, 277.6924153040722558 ) ) ;
#99215=CARTESIAN_POINT ( 'NONE',  ( -75.71374782820129212, 1384.771513434549888, 276.6754848879950259 ) ) ;
#99225=CARTESIAN_POINT ( 'NONE',  ( -14.01398736212220086, 1379.590348564800024, 211.9184487047760115 ) ) ;
#99284=CARTESIAN_POINT ( 'NONE',  ( -31.70262514495150086, 1384.822076339110254, 229.9359219034049886 ) ) ;
#99285=CARTESIAN_POINT ( 'NONE',  ( -106.4316804820100089, 1391.913060387289988, 303.6209942796789960 ) ) ;
#99287=CARTESIAN_POINT ( 'NONE',  ( -105.6089689389999933, 1379.039522535980041, 302.3092273913590020 ) ) ;
#99290=VECTOR ( 'NONE', #109077, 1000.000000000000000 ) ;
#99301=CARTESIAN_POINT ( 'NONE',  ( -12.86192383983290100, 1379.355455732259998, 211.5054726329910011 ) ) ;
#99310=CARTESIAN_POINT ( 'NONE',  ( 6.490272193332720122E-14, 1378.020218211860083, 211.7927966155920103 ) ) ;
#99339=CARTESIAN_POINT ( 'NONE',  ( -109.6623370671470781, 1386.518664481797941, 311.2475360254030079 ) ) ;
#99342=CARTESIAN_POINT ( 'NONE',  ( -12.64090277919120098, 1379.240988027499952, 208.6656503568100050 ) ) ;
#99346=CARTESIAN_POINT ( 'NONE',  ( -44.99452937809999753, 1375.083786706710043, 231.7591686826590092 ) ) ;
#99360=CARTESIAN_POINT ( 'NONE',  ( -54.20202940400000102, 1384.105748123020021, 270.3343205631590536 ) ) ;
#99366=CARTESIAN_POINT ( 'NONE',  ( -51.85551458690000004, 1379.702026082089787, 243.6795232500590203 ) ) ;
#99376=CARTESIAN_POINT ( 'NONE',  ( -26.06393844649999991, 1386.902048729640001, 224.0886486646589901 ) ) ;
#99378=CARTESIAN_POINT ( 'NONE',  ( -41.85805827384730549, 1385.171263413119959, 245.4604812281340287 ) ) ;
#99382=AXIS2_PLACEMENT_3D ( 'NONE', #4520, #40308, #56575 ) ;
#99406=CARTESIAN_POINT ( 'NONE',  ( -107.1300166679999961, 1387.670188495179900, 298.1786851041590012 ) ) ;
#99409=VERTEX_POINT ( 'NONE', #62637 ) ;
#99410=CARTESIAN_POINT ( 'NONE',  ( -105.5086717259999887, 1378.552684895010088, 304.0447740192590231 ) ) ;
#99427=ORIENTED_EDGE ( 'NONE', *, *, #20132, .T. ) ;
#99428=CARTESIAN_POINT ( 'NONE',  ( -96.27487712110000473, 1383.766385264410019, 310.4021576922589816 ) ) ;
#99449=AXIS2_PLACEMENT_3D ( 'NONE', #54946, #29175, #63365 ) ;
#99460=CARTESIAN_POINT ( 'NONE',  ( -8.857648614099998596, 1384.596810254769935, 199.9412065693690010 ) ) ;
#99479=CARTESIAN_POINT ( 'NONE',  ( -19.40145187611040001, 1384.532064108600025, 201.5288265737380016 ) ) ;
#99493=CARTESIAN_POINT ( 'NONE',  ( -68.77190080519999071, 1379.747925807450201, 280.3125203366930123 ) ) ;
#99500=ORIENTED_EDGE ( 'NONE', *, *, #45337, .F. ) ;
#99504=EDGE_LOOP ( 'NONE', ( #81216, #65343, #49547, #28059 ) ) ;
#99512=CARTESIAN_POINT ( 'NONE',  ( -14.07887498544812743, 1379.617235141234687, 211.6859004506403323 ) ) ;
#99550=CARTESIAN_POINT ( 'NONE',  ( -39.50122532003389608, 1383.828917900590113, 240.9233743668259820 ) ) ;
#99559=CARTESIAN_POINT ( 'NONE',  ( -27.25467149600000027, 1380.910011778850276, 222.6012197218589677 ) ) ;
#99568=CARTESIAN_POINT ( 'NONE',  ( -103.9362963259999901, 1380.106856784760112, 301.6745611782590117 ) ) ;
#99587=CARTESIAN_POINT ( 'NONE',  ( -109.6649067579999866, 1386.049555229090174, 311.2750003182590035 ) ) ;
#99597=CARTESIAN_POINT ( 'NONE',  ( -14.47191459792289869, 1379.648775954749908, 208.1784578746709826 ) ) ;
#99616=CARTESIAN_POINT ( 'NONE',  ( -53.47023167649999920, 1385.031515079650262, 230.7490043923590122 ) ) ;
#99635=DIRECTION ( 'NONE',  ( -1.836970198721029688E-16, -1.000000000000000000, -8.835242138475329394E-33 ) ) ;
#99644=CARTESIAN_POINT ( 'NONE',  ( -105.6427474625459979, 1391.452704347849931, 305.6364936059279671 ) ) ;
#99654=CARTESIAN_POINT ( 'NONE',  ( -94.85908788526670321, 1384.958307967540122, 310.0174651394229386 ) ) ;
#99655=CARTESIAN_POINT ( 'NONE',  ( -8.851511101499999867, 1386.548753862859940, 200.1620584707990247 ) ) ;
#99668=CARTESIAN_POINT ( 'NONE',  ( -109.3076880190397020, 1387.423153082153476, 297.4241389203062909 ) ) ;
#99683=VERTEX_POINT ( 'NONE', #56761 ) ;
#99695=CARTESIAN_POINT ( 'NONE',  ( -5.013264356492538099, 1375.413060387289761, 214.7179447576738482 ) ) ;
#99700=CARTESIAN_POINT ( 'NONE',  ( -12.28572795910000082, 1378.826156777889992, 210.3262432577790264 ) ) ;
#99702=CARTESIAN_POINT ( 'NONE',  ( -66.59252740955220418, 1385.094901321110001, 258.5833803216879687 ) ) ;
#99710=CARTESIAN_POINT ( 'NONE',  ( -109.1310914430000167, 1384.891515483489911, 311.2646936322590250 ) ) ;
#99714=CARTESIAN_POINT ( 'NONE',  ( -109.1321484620000035, 1384.869787276959869, 311.2644936502589985 ) ) ;
#99732=CARTESIAN_POINT ( 'NONE',  ( -109.1655177890000061, 1384.872414444939977, 297.1329087538589420 ) ) ;
#99735=CARTESIAN_POINT ( 'NONE',  ( -68.71636368279999374, 1379.747847531599973, 280.3054625287589943 ) ) ;
#99738=CARTESIAN_POINT ( 'NONE',  ( -11.05880225982243381, 1378.497832814331559, 214.5800325812288918 ) ) ;
#99748=CARTESIAN_POINT ( 'NONE',  ( -106.9640595847560007, 1378.913060387289988, 307.1352131009099935 ) ) ;
#99764=CARTESIAN_POINT ( 'NONE',  ( -13.17512049819999831, 1379.550058867589996, 208.3055830647739697 ) ) ;
#99770=CARTESIAN_POINT ( 'NONE',  ( -72.30335119138749178, 1384.751552219569930, 270.5210238762560380 ) ) ;
#99774=ORIENTED_EDGE ( 'NONE', *, *, #30123, .T. ) ;
#99778=CARTESIAN_POINT ( 'NONE',  ( -113.4235965852909089, 1389.413060387289988, 305.2215675190763591 ) ) ;
#99801=ORIENTED_EDGE ( 'NONE', *, *, #89858, .F. ) ;
#99841=CARTESIAN_POINT ( 'NONE',  ( -42.50846000140169423, 1384.776023261829778, 246.7016633287670118 ) ) ;
#99844=CARTESIAN_POINT ( 'NONE',  ( -105.4748898929999967, 1378.947219630530071, 303.4796662018589473 ) ) ;
#99855=DIRECTION ( 'NONE',  ( 1.836970198721029688E-16, 1.000000000000000000, 0.000000000000000000 ) ) ;
#99864=CARTESIAN_POINT ( 'NONE',  ( -18.09482676940919887, 1377.903424712840206, 213.0196949892159921 ) ) ;
#99866=CARTESIAN_POINT ( 'NONE',  ( -36.41835043334280186, 1379.641566369280099, 223.8136772429340056 ) ) ;
#99875=CARTESIAN_POINT ( 'NONE',  ( -8.861333410889999485, 1384.870662623869976, 218.6848950059889773 ) ) ;
#99889=ORIENTED_EDGE ( 'NONE', *, *, #499, .T. ) ;
#99894=CARTESIAN_POINT ( 'NONE',  ( -108.2218672464631197, 1388.808672301278648, 310.1868769870816323 ) ) ;
#99896=CARTESIAN_POINT ( 'NONE',  ( -13.74255644588489922, 1380.321565345840099, 209.5209940965139879 ) ) ;
#99901=CARTESIAN_POINT ( 'NONE',  ( -57.85314987360000316, 1374.895658628189949, 259.2190729278590311 ) ) ;
#99917=CARTESIAN_POINT ( 'NONE',  ( -67.04611378480001349, 1384.669946114650202, 292.1828053715589704 ) ) ;
#99931=CARTESIAN_POINT ( 'NONE',  ( -22.00954832700000097, 1389.608130893230054, 205.5395550013790285 ) ) ;
#99933=CARTESIAN_POINT ( 'NONE',  ( -42.90628611040540363, 1385.165074035010093, 247.4351966983790021 ) ) ;
#99943=CARTESIAN_POINT ( 'NONE',  ( -7.769040032840000443, 1384.899909079960025, 218.9179066534690037 ) ) ;
#99956=AXIS2_PLACEMENT_3D ( 'NONE', #98230, #89833, #9409 ) ;
#99961=CARTESIAN_POINT ( 'NONE',  ( -108.1807521070000035, 1387.239101882400064, 297.7772244688590035 ) ) ;
#99962=ADVANCED_FACE ( 'NONE', ( #8507, #49983 ), #33710, .F. ) ;
#100015=CARTESIAN_POINT ( 'NONE',  ( -5.013435694540000043, 1375.426148861440197, 214.7180213005390215 ) ) ;
#100031=EDGE_CURVE ( 'NONE', #53370, #110657, #55187, .T. ) ;
#100046=CARTESIAN_POINT ( 'NONE',  ( -22.03947762662830101, 1384.537944471270066, 202.2607269266779895 ) ) ;
#100063=FACE_OUTER_BOUND ( 'NONE', #99504, .T. ) ;
#100065=CARTESIAN_POINT ( 'NONE',  ( -109.1322461037039915, 1384.978503018139918, 313.2642998889880346 ) ) ;
#100074=CARTESIAN_POINT ( 'NONE',  ( -8.744990863649999113, 1385.315572773260101, 218.5566709142290165 ) ) ;
#100103=CARTESIAN_POINT ( 'NONE',  ( -109.1637285801670032, 1385.118900514759844, 297.1380744252289787 ) ) ;
#100118=CARTESIAN_POINT ( 'NONE',  ( -51.20695252170450118, 1383.809936270029993, 263.8239077099820520 ) ) ;
#100128=CARTESIAN_POINT ( 'NONE',  ( -22.99522306489999579, 1384.540050732020063, 202.4077213122689898 ) ) ;
#100132=CARTESIAN_POINT ( 'NONE',  ( -8.517264636099429964, 1385.713703502809949, 218.6243582954489852 ) ) ;
#100137=CARTESIAN_POINT ( 'NONE',  ( -105.9813432219999925, 1380.125633722419934, 300.4093128206589540 ) ) ;
#100156=CARTESIAN_POINT ( 'NONE',  ( -108.7028354350000114, 1386.982920307299764, 310.7828582002589428 ) ) ;
#100161=ADVANCED_FACE ( 'NONE', ( #2777 ), #5028, .F. ) ;
#100189=CARTESIAN_POINT ( 'NONE',  ( -75.49308973149999247, 1385.139059930169878, 276.6890413075590232 ) ) ;
#100194=CARTESIAN_POINT ( 'NONE',  ( -105.1200804420000026, 1379.260731124600170, 305.2465900763589843 ) ) ;
#100224=CARTESIAN_POINT ( 'NONE',  ( -11.59204932530000143, 1378.005205810240113, 213.3426278446090123 ) ) ;
#100232=CARTESIAN_POINT ( 'NONE',  ( -9.105351999590000744, 1386.405645367540046, 200.2123243072389869 ) ) ;
#100244=CARTESIAN_POINT ( 'NONE',  ( -108.6316274086125020, 1388.459345456638630, 297.9094210424456151 ) ) ;
#100247=CIRCLE ( 'NONE', #1967, 3.500000000000003109 ) ;
#100270=CARTESIAN_POINT ( 'NONE',  ( -107.4425579992611830, 1382.651356145541286, 310.5015941399482244 ) ) ;
#100275=CARTESIAN_POINT ( 'NONE',  ( -12.54840892090000004, 1379.545626517140136, 210.2256536815890229 ) ) ;
#100277=CARTESIAN_POINT ( 'NONE',  ( -60.62137868135909713, 1385.064398150979741, 245.3311423290439848 ) ) ;
#100288=CARTESIAN_POINT ( 'NONE',  ( -109.6584366050000057, 1384.889060011860010, 311.3230549062590171 ) ) ;
#100303=CARTESIAN_POINT ( 'NONE',  ( -68.62161786750179715, 1379.747591873680221, 280.2379983867550095 ) ) ;
#100306=CARTESIAN_POINT ( 'NONE',  ( -8.779627249246892973, 1381.198063572799583, 217.8823406631832142 ) ) ;
#100314=CARTESIAN_POINT ( 'NONE',  ( -107.4534871969369902, 1378.913060387289988, 307.7877216430330236 ) ) ;
#100315=CARTESIAN_POINT ( 'NONE',  ( -14.48037769471150149, 1379.715043008649900, 208.2752642513599994 ) ) ;
#100333=CARTESIAN_POINT ( 'NONE',  ( -12.31888632829999963, 1377.996605653940151, 209.2056224726200071 ) ) ;
#100337=CARTESIAN_POINT ( 'NONE',  ( -10.58542156100000042, 1391.805874643410107, 214.6478040594989807 ) ) ;
#100338=CARTESIAN_POINT ( 'NONE',  ( -77.54941825186959647, 1384.781592401509897, 279.6170682065900337 ) ) ;
#100378=DIRECTION ( 'NONE',  ( 1.000000000000000000, 0.000000000000000000, 0.000000000000000000 ) ) ;
#100389=CARTESIAN_POINT ( 'NONE',  ( -10.53528427685149005, 1390.796569291690957, 215.5647122002405638 ) ) ;
#100401=AXIS2_PLACEMENT_3D ( 'NONE', #63021, #80330, #38853 ) ;
#100406=CARTESIAN_POINT ( 'NONE',  ( -45.18590935617369553, 1384.763297676119919, 251.9116518250590389 ) ) ;
#100407=CARTESIAN_POINT ( 'NONE',  ( -106.9011555262299993, 1391.913060387289988, 301.9300221985360508 ) ) ;
#100435=CARTESIAN_POINT ( 'NONE',  ( -59.67093331630000108, 1379.746016655649782, 264.7494437565589465 ) ) ;
#100467=CARTESIAN_POINT ( 'NONE',  ( -19.31603552230000176, 1376.225470561590100, 208.2524156231209815 ) ) ;
#100469=ORIENTED_EDGE ( 'NONE', *, *, #58439, .T. ) ;
#100481=CARTESIAN_POINT ( 'NONE',  ( -59.38610754540000158, 1383.797318715759957, 279.8430129459590034 ) ) ;
#100494=CARTESIAN_POINT ( 'NONE',  ( -67.04318418450000649, 1385.033547286170005, 292.1847026260589928 ) ) ;
#100496=CARTESIAN_POINT ( 'NONE',  ( -48.92494107440639795, 1385.128557567969892, 259.5107056320019865 ) ) ;
#100506=CARTESIAN_POINT ( 'NONE',  ( -8.297843675610002023, 1384.899870833489786, 218.7036046430589806 ) ) ;
#100519=CARTESIAN_POINT ( 'NONE',  ( -106.5585968837300044, 1390.939245634569943, 300.3884029622149683 ) ) ;
#100522=CARTESIAN_POINT ( 'NONE',  ( -106.7184954779999941, 1387.980454484629945, 298.4661214286589939 ) ) ;
#100524=CARTESIAN_POINT ( 'NONE',  ( -105.8054920000000010, 1391.680210928180031, 302.6861668426589631 ) ) ;
#100543=CARTESIAN_POINT ( 'NONE',  ( -13.41288733981332015, 1379.525778898297631, 211.7978688460160015 ) ) ;
#100561=ORIENTED_EDGE ( 'NONE', *, *, #39389, .F. ) ;
#100576=CARTESIAN_POINT ( 'NONE',  ( -12.32169104970000006, 1391.303891397440111, 206.9552536725390155 ) ) ;
#100592=CARTESIAN_POINT ( 'NONE',  ( -42.79837815356560071, 1384.591774741229983, 215.7805842356740129 ) ) ;
#100601=CARTESIAN_POINT ( 'NONE',  ( -9.813982587879999997, 1383.225161719749849, 200.4195862986289853 ) ) ;
#100605=CARTESIAN_POINT ( 'NONE',  ( -68.75987617920000616, 1379.748052094799959, 280.1906344666589916 ) ) ;
#100622=CARTESIAN_POINT ( 'NONE',  ( 12.49965726624219187, 1384.899971913130003, 209.1218459572589836 ) ) ;
#100632=CARTESIAN_POINT ( 'NONE',  ( -7.545178029317930246, 1384.916914618600003, 219.0875785980250043 ) ) ;
#100653=CARTESIAN_POINT ( 'NONE',  ( -37.80963358037920585, 1383.831454921230034, 238.1220177388399861 ) ) ;
#100664=CARTESIAN_POINT ( 'NONE',  ( -46.83374554580000648, 1379.942045336279762, 245.6713053846590071 ) ) ;
#100676=CARTESIAN_POINT ( 'NONE',  ( -107.6180288740000037, 1380.687228087200083, 298.7908680479590089 ) ) ;
#100693=CARTESIAN_POINT ( 'NONE',  ( -107.4345822860000084, 1387.580258537220061, 310.2252759172590117 ) ) ;
#100703=CARTESIAN_POINT ( 'NONE',  ( -14.17772861730700207, 1379.591530685439920, 207.8208986668599891 ) ) ;
#100716=ORIENTED_EDGE ( 'NONE', *, *, #29533, .F. ) ;
#100721=CARTESIAN_POINT ( 'NONE',  ( -62.45870848130000041, 1384.816439370750004, 249.2996736312589974 ) ) ;
#100729=CARTESIAN_POINT ( 'NONE',  ( -10.44070837812300034, 1391.913060387289988, 204.6731945046309704 ) ) ;
#100750=CARTESIAN_POINT ( 'NONE',  ( -11.32418084390000068, 1378.916280331980033, 214.2342780821290091 ) ) ;
#100756=CARTESIAN_POINT ( 'NONE',  ( -10.29442817569999846, 1389.680258987810021, 202.2226486107689993 ) ) ;
#100763=CARTESIAN_POINT ( 'NONE',  ( -8.864146540411450559, 1384.685144641450051, 218.6774944319709846 ) ) ;
#100767=EDGE_CURVE ( 'NONE', #43749, #49944, #88827, .T. ) ;
#100777=CARTESIAN_POINT ( 'NONE',  ( -5.513264357029999729, 1374.913060387289988, 203.3066656689789795 ) ) ;
#100792=CARTESIAN_POINT ( 'NONE',  ( -109.3493610729999972, 1384.903287640260032, 297.1385568369590260 ) ) ;
#100797=CARTESIAN_POINT ( 'NONE',  ( -9.016783256541959446, 1383.231411182179954, 220.4219636834260143 ) ) ;
#100806=CARTESIAN_POINT ( 'NONE',  ( -54.91437447499630053, 1385.038116820099958, 233.6872214610490062 ) ) ;
#100807=CARTESIAN_POINT ( 'NONE',  ( -10.91810810328910009, 1391.913060387289988, 212.7120084556750044 ) ) ;
#100817=CARTESIAN_POINT ( 'NONE',  ( -109.1218945300000058, 1384.640297123439950, 311.2547333012590229 ) ) ;
#100831=CARTESIAN_POINT ( 'NONE',  ( -11.13055623967079555, 1375.886883438980021, 214.2704005330025723 ) ) ;
#100833=CARTESIAN_POINT ( 'NONE',  ( -68.66495634729999153, 1379.747814253419847, 280.2580260664590242 ) ) ;
#100843=CARTESIAN_POINT ( 'NONE',  ( -106.6934947193090011, 1378.913060387289988, 306.7339471936149948 ) ) ;
#100865=CARTESIAN_POINT ( 'NONE',  ( -11.44054090840000093, 1391.153937292269802, 213.9067485665989921 ) ) ;
#100866=CARTESIAN_POINT ( 'NONE',  ( -83.03334324507059705, 1384.808909933130053, 286.7532168304919651 ) ) ;
#100886=ADVANCED_FACE ( 'NONE', ( #15128 ), #58680, .T. ) ;
#100913=CARTESIAN_POINT ( 'NONE',  ( -5.513264357029999729, 1375.413060387289988, 209.1218459572589836 ) ) ;
#100938=CARTESIAN_POINT ( 'NONE',  ( -45.76759480931980306, 1384.760497626650022, 253.0762944135069858 ) ) ;
#100939=CARTESIAN_POINT ( 'NONE',  ( -106.5202740518050035, 1391.913060387289988, 303.0849643599170236 ) ) ;
#100943=B_SPLINE_SURFACE_WITH_KNOTS ( 'NONE', 5, 5, ( 
 ( #61595, #53190, #44795, #45352, #103569, #78948, #26870, #61060, #17887 ),
 ( #51521, #36368, #2255, #27971, #77286, #94059, #52086, #584, #85655 ),
 ( #18436, #34711, #68902, #79492, #103003, #52636, #70560, #9509, #104677 ),
 ( #34162, #43676, #25741, #68348, #102454, #77828, #1136, #63265, #22291 ),
 ( #12263, #4438, #47540, #73288, #62725, #4965, #13347, #20114, #46453 ),
 ( #80586, #21742, #3901, #81659, #36919, #97917, #29616, #38030, #2801 ),
 ( #97376, #98473, #63801, #56493, #88973, #38564, #54849, #90622, #64905 ),
 ( #72209, #30720, #55395, #72742, #29081, #39110, #64351, #107424, #3353 ),
 ( #99013, #80032, #71113, #106332, #20647, #13902, #48089, #105801, #89527 ),
 ( #45896, #96847, #21186, #37478, #105237, #28526, #54306, #12817, #88435 ),
 ( #46997, #81120, #106869, #71681, #30160, #55944, #90065, #11726, #101209 ),
 ( #107976, #108533, #49200, #59258, #24505, #109103, #40778, #50307, #93375 ),
 ( #57054, #74954, #82779, #58696, #66011, #58148, #14460, #16642, #31823 ),
 ( #91728, #6072, #92828, #110185, #5528, #100132, #84437, #82227, #39682 ),
 ( #91180, #23952, #73849, #40225, #65457, #66566, #67107, #7721, #75507 ) ),
 .UNSPECIFIED., .F., .F., .F.,
 ( 6, 3, 3, 3, 6 ),
 ( 6, 3, 6 ),
 ( 31.54023800929859789, 39.18581663660000203, 44.09091811200000421, 49.81951809560000299, 53.72098354768269957 ),
 ( 0.000000000000000000, 1.000000000000000000, 2.000085314782729995 ),
 .UNSPECIFIED. ) ;
#100944=CARTESIAN_POINT ( 'NONE',  ( -107.3285983110000075, 1378.913060287569806, 300.3204975590590493 ) ) ;
#100948=CARTESIAN_POINT ( 'NONE',  ( -9.994751287005144036, 1380.244992563594224, 201.8194665170140070 ) ) ;
#100968=CARTESIAN_POINT ( 'NONE',  ( -11.19604652080000129, 1377.051618906870090, 211.6852637316389973 ) ) ;
#100971=CARTESIAN_POINT ( 'NONE',  ( -54.35795438361589760, 1379.711943094660000, 254.1192448666850225 ) ) ;
#100977=CARTESIAN_POINT ( 'NONE',  ( -105.3882398639999991, 1379.160164679609807, 305.8019944446589875 ) ) ;
#100998=CARTESIAN_POINT ( 'NONE',  ( -109.5436877675987688, 1386.781868541095491, 311.1752058669367216 ) ) ;
#101007=ORIENTED_EDGE ( 'NONE', *, *, #55721, .F. ) ;
#101017=CARTESIAN_POINT ( 'NONE',  ( -62.22036486049999837, 1383.793512663130059, 284.6761640327590044 ) ) ;
#101030=CARTESIAN_POINT ( 'NONE',  ( -48.48855173430000320, 1388.337145087740055, 255.7627372621590212 ) ) ;
#101032=CARTESIAN_POINT ( 'NONE',  ( -39.61210671423299345, 1385.184201439789831, 241.4309191739689879 ) ) ;
#101041=CARTESIAN_POINT ( 'NONE',  ( -8.023097652669999746, 1384.898239823859967, 218.7875342523390145 ) ) ;
#101058=CARTESIAN_POINT ( 'NONE',  ( -107.9217616539999938, 1387.054747972530095, 297.7113990731589865 ) ) ;
#101083=VERTEX_POINT ( 'NONE', #26294 ) ;
#101090=CARTESIAN_POINT ( 'NONE',  ( -17.05170201009999786, 1380.306507143900035, 210.4183098381890034 ) ) ;
#101109=CARTESIAN_POINT ( 'NONE',  ( -9.092690131330000369, 1384.838170029980120, 199.9433835858289967 ) ) ;
#101133=CARTESIAN_POINT ( 'NONE',  ( -49.07695366983040230, 1384.615622046050248, 223.8752598800379872 ) ) ;
#101138=ORIENTED_EDGE ( 'NONE', *, *, #60651, .T. ) ;
#101142=CARTESIAN_POINT ( 'NONE',  ( -12.00444414999999942, 1381.312822588570043, 202.5161199644090289 ) ) ;
#101167=CARTESIAN_POINT ( 'NONE',  ( -8.883094036332620291, 1385.283542038099995, 218.6640794153470040 ) ) ;
#101176=CARTESIAN_POINT ( 'NONE',  ( -104.3950658971828460, 1390.067543051406574, 304.1809742105791088 ) ) ;
#101187=ORIENTED_EDGE ( 'NONE', *, *, #33624, .T. ) ;
#101198=CARTESIAN_POINT ( 'NONE',  ( -61.45951696033579736, 1383.794773811220011, 283.0528198679410252 ) ) ;
#101205=CARTESIAN_POINT ( 'NONE',  ( -54.73637590230000427, 1382.331405336219859, 270.0802247036589847 ) ) ;
#101209=CARTESIAN_POINT ( 'NONE',  ( -9.775751096677179675, 1386.869787730469852, 218.1689280660520183 ) ) ;
#101214=CARTESIAN_POINT ( 'NONE',  ( -106.3258853770000059, 1381.775203003109937, 298.5533487220590132 ) ) ;
#101231=CARTESIAN_POINT ( 'NONE',  ( -108.3007714539999995, 1388.465142555530065, 310.2841513672590281 ) ) ;
#101239=CARTESIAN_POINT ( 'NONE',  ( -14.42421378022759981, 1379.620479347240007, 208.1098118855669838 ) ) ;
#101253=FACE_OUTER_BOUND ( 'NONE', #49114, .T. ) ;
#101258=CARTESIAN_POINT ( 'NONE',  ( -64.54217663740000432, 1384.956766891789812, 254.0305872787589863 ) ) ;
#101266=EDGE_CURVE ( 'NONE', #62022, #6492, #71627, .T. ) ;
#101268=ADVANCED_FACE ( 'NONE', ( #44789 ), #65953, .F. ) ;
#101269=CARTESIAN_POINT ( 'NONE',  ( -11.17502343409620025, 1391.913060387130145, 206.4900290431199892 ) ) ;
#101290=CARTESIAN_POINT ( 'NONE',  ( -12.22846866959999979, 1380.845870869829923, 215.9110647297389960 ) ) ;
#101296=CARTESIAN_POINT ( 'NONE',  ( -10.79874708580000053, 1388.923907300369819, 202.4036804765890167 ) ) ;
#101331=FACE_OUTER_BOUND ( 'NONE', #20476, .T. ) ;
#101335=CARTESIAN_POINT ( 'NONE',  ( -104.3428327140408385, 1380.439868052300881, 307.2882731461818366 ) ) ;
#101343=CARTESIAN_POINT ( 'NONE',  ( -69.86459936517930203, 1385.111636070419763, 265.6217149743549726 ) ) ;
#101354=CARTESIAN_POINT ( 'NONE',  ( -109.9857361549999979, 1384.899971913130003, 311.4562995532589866 ) ) ;
#101371=CARTESIAN_POINT ( 'NONE',  ( -68.69690608884340577, 1379.747745670520089, 280.2939418190039760 ) ) ;
#101398=B_SPLINE_CURVE_WITH_KNOTS ( 'NONE', 3,
 ( #95733, #26305, #36923, #78385, #71119, #103008, #1141, #27417 ),
 .UNSPECIFIED., .F., .F.,
 ( 4, 2, 2, 4 ),
 ( 0.000000000000000000, 0.2500000000000000000, 0.5000000000000000000, 1.000000000000000000 ),
 .UNSPECIFIED. ) ;
#101407=CARTESIAN_POINT ( 'NONE',  ( -11.62394760940000005, 1391.913060725860078, 211.5064627571190101 ) ) ;
#101408=CARTESIAN_POINT ( 'NONE',  ( -90.63163529889820325, 1384.841170975159912, 292.9371972892139411 ) ) ;
#101417=ORIENTED_EDGE ( 'NONE', *, *, #104128, .T. ) ;
#101426=CARTESIAN_POINT ( 'NONE',  ( -56.81483858269999843, 1379.709620124910089, 254.2646988397590064 ) ) ;
#101443=CARTESIAN_POINT ( 'NONE',  ( -8.371438357349999748, 1384.922515940929998, 199.7749755103790221 ) ) ;
#101460=B_SPLINE_CURVE_WITH_KNOTS ( 'NONE', 3,
 ( #31079, #65262, #13155, #28890, #98283, #106682 ),
 .UNSPECIFIED., .F., .F.,
 ( 4, 2, 4 ),
 ( 0.000000000000000000, 0.5000000000000000000, 1.000000000000000000 ),
 .UNSPECIFIED. ) ;
#101465=CARTESIAN_POINT ( 'NONE',  ( -8.064928480694979029, 1387.323551673170186, 218.5893119357714056 ) ) ;
#101482=CARTESIAN_POINT ( 'NONE',  ( -52.68643441635880720, 1384.727329538739923, 267.2268374729209768 ) ) ;
#101491=CARTESIAN_POINT ( 'NONE',  ( -8.993343321902724341, 1381.641526762418835, 200.5640689155782184 ) ) ;
#101505=EDGE_CURVE ( 'NONE', #22898, #94821, #103492, .T. ) ;
#101512=CARTESIAN_POINT ( 'NONE',  ( -35.85012805650530510, 1380.172836987449955, 220.5089525084339925 ) ) ;
#101514=CARTESIAN_POINT ( 'NONE',  ( -21.66469037441770240, 1379.608053137539855, 213.7100242930600018 ) ) ;
#101520=CARTESIAN_POINT ( 'NONE',  ( -106.0334448509999987, 1378.913060387289988, 305.5503496670590380 ) ) ;
#101547=CARTESIAN_POINT ( 'NONE',  ( 1.889251328982650109E-15, 1379.483856714079820, 206.9293834673690071 ) ) ;
#101548=ORIENTED_EDGE ( 'NONE', *, *, #11341, .T. ) ;
#101577=CARTESIAN_POINT ( 'NONE',  ( -68.63560918429999447, 1386.704837996910101, 263.4658735872590114 ) ) ;
#101579=CARTESIAN_POINT ( 'NONE',  ( -39.34650272300579843, 1385.185695465040226, 240.9764786771909826 ) ) ;
#101588=CARTESIAN_POINT ( 'NONE',  ( -7.544821718529999721, 1384.901423591120192, 219.0876899922290022 ) ) ;
#101590=CARTESIAN_POINT ( 'NONE',  ( -106.4551009342630010, 1381.717765542610096, 309.6367472382920027 ) ) ;
#101604=CARTESIAN_POINT ( 'NONE',  ( -8.862056518773441027, 1384.892951007370129, 218.6851137863439760 ) ) ;
#101605=CARTESIAN_POINT ( 'NONE',  ( -108.8566410550000114, 1386.492030720920184, 297.4136311286590058 ) ) ;
#101634=CARTESIAN_POINT ( 'NONE',  ( -12.31045119098629925, 1378.376187953739873, 209.7947064970520046 ) ) ;
#101651=CARTESIAN_POINT ( 'NONE',  ( -110.0628587348610097, 1384.913582352849971, 296.9513039175640188 ) ) ;
#101654=CARTESIAN_POINT ( 'NONE',  ( -8.168610837440001049, 1384.459582517680019, 199.6726098237590179 ) ) ;
#101672=B_SPLINE_CURVE_WITH_KNOTS ( 'NONE', 3,
 ( #35052, #16025, #67577, #42350, #58617, #110654, #9310 ),
 .UNSPECIFIED., .F., .F.,
 ( 4, 3, 4 ),
 ( 0.000000000000000000, 0.3299121248754509628, 0.5294136330519999545 ),
 .UNSPECIFIED. ) ;
#101675=CARTESIAN_POINT ( 'NONE',  ( -113.4000000000000057, 1379.413060387289988, 304.2218459572590064 ) ) ;
#101682=CARTESIAN_POINT ( 'NONE',  ( -34.42078214483079535, 1384.567160501399940, 208.3171832722069894 ) ) ;
#101689=CARTESIAN_POINT ( 'NONE',  ( -68.70880675088680789, 1379.747766871069871, 280.3821654378152175 ) ) ;
#101695=CARTESIAN_POINT ( 'NONE',  ( -68.69440785229998880, 1379.747830596759968, 279.9872465871590066 ) ) ;
#101704=CARTESIAN_POINT ( 'NONE',  ( -3.078458293700000237, 1385.332091261079995, 218.5458417419390003 ) ) ;
#101710=CARTESIAN_POINT ( 'NONE',  ( 0.000000000000000000, 1384.913060387289988, 209.1218459572589836 ) ) ;
#101719=CARTESIAN_POINT ( 'NONE',  ( -8.865470775637810164, 1385.143464112529955, 218.6765624161500057 ) ) ;
#101726=EDGE_LOOP ( 'NONE', ( #108531, #17652, #109407, #56822 ) ) ;
#101734=DIRECTION ( 'NONE',  ( 0.000000000000000000, -1.000000000000000000, 0.000000000000000000 ) ) ;
#101754=CARTESIAN_POINT ( 'NONE',  ( -63.46805869144479573, 1383.792271846660014, 286.2010029998429559 ) ) ;
#101761=CARTESIAN_POINT ( 'NONE',  ( -61.91320719539999828, 1380.491709420169855, 255.2400922398589955 ) ) ;
#101764=ORIENTED_EDGE ( 'NONE', *, *, #93484, .T. ) ;
#101770=CARTESIAN_POINT ( 'NONE',  ( -108.7044653689999905, 1381.736054483690168, 297.8421293474590357 ) ) ;
#101787=CARTESIAN_POINT ( 'NONE',  ( -8.861662123853877304, 1384.878099886156406, 218.6849989278500459 ) ) ;
#101794=CARTESIAN_POINT ( 'NONE',  ( -108.0120647289999880, 1388.816386314980036, 310.0183359962589975 ) ) ;
#101806=ORIENTED_EDGE ( 'NONE', *, *, #43355, .F. ) ;
#101824=CIRCLE ( 'NONE', #80368, 6.842541678089994583 ) ;
#101830=CARTESIAN_POINT ( 'NONE',  ( -10.98953490978640168, 1391.913060387049882, 205.9689414614919940 ) ) ;
#101851=CARTESIAN_POINT ( 'NONE',  ( -10.74491738439999899, 1379.840458593170069, 215.5533963907290058 ) ) ;
#101858=CARTESIAN_POINT ( 'NONE',  ( -11.54624697350000062, 1388.394384052139912, 202.2644599199190054 ) ) ;
#101899=CARTESIAN_POINT ( 'NONE',  ( -108.9164604828789180, 1381.958826580047571, 310.7542428962289023 ) ) ;
#101904=CARTESIAN_POINT ( 'NONE',  ( -74.59479506201390109, 1385.134432623380007, 274.7545841228630366 ) ) ;
#101905=CARTESIAN_POINT ( 'NONE',  ( -10.31564862673620020, 1391.913060387289988, 213.9236953778939778 ) ) ;
#101907=VERTEX_POINT ( 'NONE', #66986 ) ;
#101916=B_SPLINE_CURVE_WITH_KNOTS ( 'NONE', 5,
 ( #47179, #79693, #81308, #2999, #38759, #72395 ),
 .UNSPECIFIED., .F., .F.,
 ( 6, 6 ),
 ( 0.000000000000000000, 1.000000000000000000 ),
 .UNSPECIFIED. ) ;
#101927=CARTESIAN_POINT ( 'NONE',  ( -4.145978979534980458E-15, 1375.413060387289988, 209.1218459572589836 ) ) ;
#101934=CARTESIAN_POINT ( 'NONE',  ( -68.50318901198390620, 1379.747522081850093, 280.0875204781369803 ) ) ;
#101947=SURFACE_SIDE_STYLE ('',( #7357 ) ) ;
#101948=CARTESIAN_POINT ( 'NONE',  ( -12.89620243338210059, 1379.263018346050103, 208.6490890656160104 ) ) ;
#101971=CARTESIAN_POINT ( 'NONE',  ( -96.75625392299259886, 1384.863480572399794, 295.5060220262309940 ) ) ;
#101989=CARTESIAN_POINT ( 'NONE',  ( -51.80693370059999836, 1379.719625093879813, 243.7027045558589862 ) ) ;
#102011=CARTESIAN_POINT ( 'NONE',  ( -113.4000000000000057, 1379.913060387289988, 304.2218459572590064 ) ) ;
#102035=LINE ( 'NONE', #85801, #12628 ) ;
#102036=CARTESIAN_POINT ( 'NONE',  ( -12.28855869350000063, 1378.253616442990051, 210.0769077263690008 ) ) ;
#102039=CARTESIAN_POINT ( 'NONE',  ( -12.50784581141053842, 1391.398398864934734, 210.4070514657185242 ) ) ;
#102041=CARTESIAN_POINT ( 'NONE',  ( -54.74134739851029963, 1384.717926922609877, 271.3113735593159959 ) ) ;
#102042=CARTESIAN_POINT ( 'NONE',  ( -14.93124696056320033, 1384.941737462140054, 200.6042365411380217 ) ) ;
#102053=CARTESIAN_POINT ( 'NONE',  ( -12.23669307423070052, 1377.661331666050273, 207.7794331870949804 ) ) ;
#102064=CARTESIAN_POINT ( 'NONE',  ( -8.629930252190000317, 1384.437861086550129, 199.9043375559089952 ) ) ;
#102077=CARTESIAN_POINT ( 'NONE',  ( -57.01644491799999770, 1379.744987730500043, 259.4421383624589907 ) ) ;
#102083=CARTESIAN_POINT ( 'NONE',  ( -105.6866551539999932, 1378.955223242689954, 305.6848347894589892 ) ) ;
#102084=CARTESIAN_POINT ( 'NONE',  ( -109.4839831700000019, 1384.925032507449941, 311.2841082172590177 ) ) ;
#102103=ORIENTED_EDGE ( 'NONE', *, *, #55979, .F. ) ;
#102114=CARTESIAN_POINT ( 'NONE',  ( -3.771520288500000539, 1380.389610323579973, 208.3364477064349956 ) ) ;
#102126=CARTESIAN_POINT ( 'NONE',  ( -102.7498137299999996, 1383.762281939259992, 311.0461218402589907 ) ) ;
#102139=CARTESIAN_POINT ( 'NONE',  ( -68.70832551159999468, 1385.106080149109857, 263.4315270082590246 ) ) ;
#102141=CARTESIAN_POINT ( 'NONE',  ( -58.60909715759989780, 1385.073142730379914, 278.5419364966310241 ) ) ;
#102148=AXIS2_PLACEMENT_3D ( 'NONE', #31378, #40333, #65560 ) ;
#102152=CARTESIAN_POINT ( 'NONE',  ( -108.3776759915979966, 1383.424114602280042, 310.9628763870520061 ) ) ;
#102175=EDGE_CURVE ( 'NONE', #36205, #78937, #2837, .T. ) ;
#102205=CARTESIAN_POINT ( 'NONE',  ( -12.30675062099569850, 1378.370996218429809, 209.8570216548399969 ) ) ;
#102217=ORIENTED_EDGE ( 'NONE', *, *, #11205, .F. ) ;
#102250=CARTESIAN_POINT ( 'NONE',  ( -42.20971106035590026, 1384.589822447700044, 215.1439631396389984 ) ) ;
#102257=CARTESIAN_POINT ( 'NONE',  ( -46.82349676020197649, 1379.680994877702915, 239.8269233030615339 ) ) ;
#102261=CARTESIAN_POINT ( 'NONE',  ( -68.73855403010000487, 1379.747900905000051, 280.1049392198590340 ) ) ;
#102279=DIRECTION ( 'NONE',  ( 1.835183309750130004E-16, 1.000000000000000000, 1.599799320660000123E-19 ) ) ;
#102282=CARTESIAN_POINT ( 'NONE',  ( -8.861665967949491574, 1385.086004207679935, 218.6801736522280066 ) ) ;
#102311=CARTESIAN_POINT ( 'NONE',  ( -60.12749137407530498, 1383.796527668070212, 280.8331374614150491 ) ) ;
#102317=CIRCLE ( 'NONE', #7544, 12.49965726619999984 ) ;
#102318=CARTESIAN_POINT ( 'NONE',  ( -32.63285090699999813, 1382.325048536849863, 229.5366794896590079 ) ) ;
#102330=CARTESIAN_POINT ( 'NONE',  ( -109.3690719439999981, 1384.479823484100052, 297.1383975656590337 ) ) ;
#102340=EDGE_CURVE ( 'NONE', #61114, #85936, #1535, .T. ) ;
#102356=CARTESIAN_POINT ( 'NONE',  ( -107.9094517300000149, 1388.661150411839799, 309.9624615272590518 ) ) ;
#102379=CARTESIAN_POINT ( 'NONE',  ( -14.53473304376390018, 1379.710786975620067, 208.2794084638009906 ) ) ;
#102389=CARTESIAN_POINT ( 'NONE',  ( -109.9849253298559972, 1384.914539739569818, 311.4561054518049446 ) ) ;
#102394=CARTESIAN_POINT ( 'NONE',  ( -11.65263573226700089, 1391.913060387150153, 208.7517851132730016 ) ) ;
#102406=CARTESIAN_POINT ( 'NONE',  ( -18.61904574209999907, 1389.810251683270280, 216.3045377948590158 ) ) ;
#102414=CARTESIAN_POINT ( 'NONE',  ( -11.84288296679999952, 1378.858663654499878, 213.2050210349089809 ) ) ;
#102421=CARTESIAN_POINT ( 'NONE',  ( -14.33548952289999967, 1390.363893295419984, 208.3507362592630159 ) ) ;
#102426=CARTESIAN_POINT ( 'NONE',  ( -8.905790132374109547, 1384.416626165959769, 218.6501556148870122 ) ) ;
#102454=CARTESIAN_POINT ( 'NONE',  ( -12.46581701093480099, 1390.671825296710040, 212.4770441740029980 ) ) ;
#102460=CARTESIAN_POINT ( 'NONE',  ( -13.48561158899999946, 1379.693418477929981, 211.4566258570390005 ) ) ;
#102461=CARTESIAN_POINT ( 'NONE',  ( -11.90356457640000087, 1391.442765664790159, 205.8043614906389962 ) ) ;
#102462=CARTESIAN_POINT ( 'NONE',  ( -84.88875595641219718, 1385.175798546129954, 288.6381895591889588 ) ) ;
#102488=CARTESIAN_POINT ( 'NONE',  ( -68.75469704279311145, 1379.747881236529793, 280.3330792319889611 ) ) ;
#102500=CARTESIAN_POINT ( 'NONE',  ( -12.36522994357800087, 1378.525463850149890, 209.2776376259250242 ) ) ;
#102519=CARTESIAN_POINT ( 'NONE',  ( -104.2765687246049993, 1384.887396391249922, 296.8490877439370479 ) ) ;
#102535=CARTESIAN_POINT ( 'NONE',  ( -44.22148322110000151, 1379.678134692099775, 229.5078809691590038 ) ) ;
#102561=CARTESIAN_POINT ( 'NONE',  ( -121.3990240114689385, 1384.913060387289988, 304.3468054064544503 ) ) ;
#102568=CARTESIAN_POINT ( 'NONE',  ( -10.39150615120248489, 1390.644890799487484, 215.8008389675831893 ) ) ;
#102585=CARTESIAN_POINT ( 'NONE',  ( -79.98755288028320365, 1384.638602750850168, 303.8468171847529788 ) ) ;
#102588=CARTESIAN_POINT ( 'NONE',  ( -106.5446895480000080, 1379.366632456400112, 300.3036432984590078 ) ) ;
#102598=CARTESIAN_POINT ( 'NONE',  ( -7.544890056106759779, 1384.926148859619843, 219.0875905756669795 ) ) ;
#102614=CARTESIAN_POINT ( 'NONE',  ( -61.32702018127960031, 1379.729903114180161, 268.3509515309739868 ) ) ;
#102620=CARTESIAN_POINT ( 'NONE',  ( -107.2961829519999952, 1379.578066573650176, 309.1743912152589928 ) ) ;
#102638=EDGE_LOOP ( 'NONE', ( #94656, #7542, #23031, #42010 ) ) ;
#102647=CARTESIAN_POINT ( 'NONE',  ( -35.12950831648389993, 1379.640695976296456, 218.1006992214701086 ) ) ;
#102648=CARTESIAN_POINT ( 'NONE',  ( -11.59474938690000023, 1376.271391995119984, 207.1178716385390146 ) ) ;
#102652=CARTESIAN_POINT ( 'NONE',  ( -104.4921371840429885, 1379.706968095510092, 304.0176578806480165 ) ) ;
#102661=CARTESIAN_POINT ( 'NONE',  ( -113.4000000000000057, 1384.024049419740095, 311.1211866832589976 ) ) ;
#102676=CARTESIAN_POINT ( 'NONE',  ( -57.30562384310000112, 1388.282717979049949, 240.5566957094589782 ) ) ;
#102678=CARTESIAN_POINT ( 'NONE',  ( -64.31586160255349682, 1385.046231101620151, 287.7684490242009474 ) ) ;
#102689=CARTESIAN_POINT ( 'NONE',  ( -108.6994105457680035, 1383.219165405780132, 310.9122041113990349 ) ) ;
#102716=DIRECTION ( 'NONE',  ( 1.000000000000000000, 0.000000000000000000, 0.000000000000000000 ) ) ;
#102720=CARTESIAN_POINT ( 'NONE',  ( -10.33108858841420030, 1384.889309772979914, 218.7842458343939995 ) ) ;
#102755=CARTESIAN_POINT ( 'NONE',  ( -8.875403652970000223, 1384.475744644940050, 199.9572674755190178 ) ) ;
#102765=B_SPLINE_SURFACE_WITH_KNOTS ( 'NONE', 5, 5, ( 
 ( #65825, #15926, #110016, #100506, #42261, #22666 ),
 ( #24341, #92108, #83704, #40051, #50127, #56866 ),
 ( #57437, #33292, #101041, #67485, #84256, #108363 ),
 ( #15385, #99943, #41706, #23238, #75866, #91562 ),
 ( #101588, #40603, #74773, #108914, #50663, #23785 ),
 ( #6998, #16472, #41157, #109473, #8093, #27124 ) ),
 .UNSPECIFIED., .F., .F., .F.,
 ( 6, 6 ),
 ( 6, 6 ),
 ( 0.4226346287780000099, 0.4682762820520000036 ),
 ( 0.000000000000000000, 2.000000000000000000 ),
 .UNSPECIFIED. ) ;
#102786=CARTESIAN_POINT ( 'NONE',  ( -37.81300040260060058, 1384.576380814120057, 210.9400181599590098 ) ) ;
#102796=CARTESIAN_POINT ( 'NONE',  ( -68.73029257049999785, 1379.747872838770036, 280.0412483861589976 ) ) ;
#102805=CARTESIAN_POINT ( 'NONE',  ( -17.46729035290000098, 1385.008859354100196, 219.9589867226589774 ) ) ;
#102808=CARTESIAN_POINT ( 'NONE',  ( -11.30456612219839840, 1385.307194473369918, 218.8490163376000055 ) ) ;
#102823=ORIENTED_EDGE ( 'NONE', *, *, #30897, .T. ) ;
#102829=CARTESIAN_POINT ( 'NONE',  ( -121.2403273175383589, 1390.939237335599955, 304.3931724222538264 ) ) ;
#102855=CARTESIAN_POINT ( 'NONE',  ( -62.46055455354049712, 1383.793505938100225, 284.6514352238460219 ) ) ;
#102857=CARTESIAN_POINT ( 'NONE',  ( -107.4477384240240099, 1379.886883745280102, 299.0757736425410371 ) ) ;
#102863=CARTESIAN_POINT ( 'NONE',  ( -50.77724190669999871, 1380.391473192369858, 232.2877509419589899 ) ) ;
#102873=CARTESIAN_POINT ( 'NONE',  ( -109.8039227080000018, 1383.848756845119851, 297.0961322820589885 ) ) ;
#102895=CARTESIAN_POINT ( 'NONE',  ( -104.7469540929999994, 1389.907464193929854, 306.5069411088589391 ) ) ;
#102905=CARTESIAN_POINT ( 'NONE',  ( -14.28029386204369899, 1390.367275669339961, 209.8449220790990069 ) ) ;
#102946=CARTESIAN_POINT ( 'NONE',  ( -3.078458307160000018, 1389.883663780020015, 214.5934223984789924 ) ) ;
#102948=CARTESIAN_POINT ( 'NONE',  ( -8.945448071766088916, 1385.615055044318524, 218.6252746482883538 ) ) ;
#102957=B_SPLINE_CURVE_WITH_KNOTS ( 'NONE', 5,
 ( #52745, #1239, #94167, #51635, #26413, #60605 ),
 .UNSPECIFIED., .F., .F.,
 ( 6, 6 ),
 ( -2.000000000000000000, 0.000000000000000000 ),
 .UNSPECIFIED. ) ;
#102966=CARTESIAN_POINT ( 'NONE',  ( -13.66482009279999943, 1390.428771231109977, 209.8137776769819993 ) ) ;
#103003=CARTESIAN_POINT ( 'NONE',  ( -12.67911190924929876, 1390.817978749060103, 211.5986899158650090 ) ) ;
#103007=CARTESIAN_POINT ( 'NONE',  ( -108.4300939784633186, 1381.280801279105845, 310.3690016902303910 ) ) ;
#103008=CARTESIAN_POINT ( 'NONE',  ( -12.27979310579503114, 1377.633317686999817, 208.2390977848808404 ) ) ;
#103011=CARTESIAN_POINT ( 'NONE',  ( -12.30071208829999918, 1391.739025408870020, 208.7164210746560116 ) ) ;
#103012=CARTESIAN_POINT ( 'NONE',  ( -67.88634661955258309, 1385.101574011260027, 261.4157710435330273 ) ) ;
#103014=CARTESIAN_POINT ( 'NONE',  ( -37.65558013879999777, 1379.730903953030065, 220.7433301062589805 ) ) ;
#103018=ORIENTED_EDGE ( 'NONE', *, *, #96150, .F. ) ;
#103036=CARTESIAN_POINT ( 'NONE',  ( -68.77190087506669158, 1379.747925807530009, 280.3125204381590265 ) ) ;
#103038=AXIS2_PLACEMENT_3D ( 'NONE', #76544, #61433, #33989 ) ;
#103049=CARTESIAN_POINT ( 'NONE',  ( -12.95149561310000053, 1379.302527901269741, 208.6156618013899902 ) ) ;
#103072=CARTESIAN_POINT ( 'NONE',  ( -89.55229520999530735, 1384.836914095840029, 292.2851226604299768 ) ) ;
#103073=ORIENTED_EDGE ( 'NONE', *, *, #35568, .F. ) ;
#103090=CARTESIAN_POINT ( 'NONE',  ( -41.85969401239999854, 1379.735023715520128, 226.1594769080589913 ) ) ;
#103144=CARTESIAN_POINT ( 'NONE',  ( -65.00736949162829603, 1384.677693943300028, 288.7496629741240213 ) ) ;
#103145=CARTESIAN_POINT ( 'NONE',  ( -27.68635198675820064, 1384.964471995969916, 204.4027686579379974 ) ) ;
#103150=CARTESIAN_POINT ( 'NONE',  ( -8.848016400190001463, 1384.939924038890013, 199.9247971377489819 ) ) ;
#103162=CARTESIAN_POINT ( 'NONE',  ( -1.742717375088950107E-15, 1375.426148861440197, 209.1218459572589836 ) ) ;
#103174=CARTESIAN_POINT ( 'NONE',  ( -61.44418850211069838, 1379.737850744239950, 268.2889715896209850 ) ) ;
#103180=CARTESIAN_POINT ( 'NONE',  ( -108.0661743619999982, 1378.913060387289988, 308.5496304198589996 ) ) ;
#103205=CARTESIAN_POINT ( 'NONE',  ( -60.87734639771428391, 1379.727522264731078, 263.3640292216577450 ) ) ;
#103208=VERTEX_POINT ( 'NONE', #4109 ) ;
#103210=EDGE_LOOP ( 'NONE', ( #79905, #28416, #10829, #82110, #4412, #102103, #75369 ) ) ;
#103233=CARTESIAN_POINT ( 'NONE',  ( -76.09690353929998707, 1385.004314140359838, 301.2232021421590389 ) ) ;
#103236=EDGE_CURVE ( 'NONE', #53370, #40922, #38233, .T. ) ;
#103245=CARTESIAN_POINT ( 'NONE',  ( -107.6819331251149947, 1381.733213848179957, 310.0307816245309596 ) ) ;
#103246=ORIENTED_EDGE ( 'NONE', *, *, #56826, .T. ) ;
#103273=CARTESIAN_POINT ( 'NONE',  ( -17.16271615814169849, 1384.870831643229849, 219.9644665330189923 ) ) ;
#103274=B_SPLINE_CURVE_WITH_KNOTS ( 'NONE', 3,
 ( #44383, #27562, #61746, #33741, #69043, #34854, #85245, #67936, #94200, #102042, #1838, #9643, #10207, #77964, #34303, #18040, #78527, #104275, #59525, #1272, #85809, #25329, #76870, #26446, #95322, #183, #69599, #27018, #16372, #70163, #18584, #84696, #35411, #93637, #52779, #16917, #17471, #43274, #77420, #724, #103145, #60640, #38706, #104825, #79092, #87486, #80175, #106474, #2945, #53910, #63949, #2400, #105942, #29221, #55540, #47131, #97525, #11330, #10773, #29759, #95868, #20795, #20252, #11871, #21334, #38164, #4036, #72882, #107020, #37066, #98063, #30308, #12409, #37619, #71821, #19707, #79643, #54997, #63410, #89664, #12950, #44945, #81257, #46593, #89120, #4572, #46043, #54452, #71262, #62302, #80728, #19134, #53338, #36518, #70711, #72345, #3491, #28111, #105383, #96429, #88045, #45501, #28671, #62876, #96988, #88588, #5676, #39822, #56077, #31963, #73983, #108113, #109782, #49885, #90766, #84018, #75093, #7318, #58283, #15143, #5107, #66698, #90203, #100806, #39262, #109242, #83459, #82917, #47677, #65032, #6754, #48795, #99150, #92408, #24094, #65589, #41482, #107570, #15680, #22994, #75643, #40914, #49333, #6209, #73436, #64498, #100277, #31407, #23557, #91323, #14046, #66156, #14605, #98614, #81806, #57749, #21877, #13487, #48236, #32526, #30857, #22428, #91869, #40360, #74541, #56630, #82377, #99702, #108673, #57199, #77835, #24634, #77294, #103012, #25196, #18445, #60500, #42575, #86225, #9516, #101343, #86781, #67248, #10070, #61069, #94622, #51531, #26308, #85115, #43136, #592, #33599, #101904, #52644, #85665, #92968, #84569, #39, #44244, #50986, #25750, #76726, #78388, #33060, #59399, #58831, #43684, #16240, #26880, #17897, #7860, #59952, #34170, #52094, #67794, #68356, #103578, #95186, #68910, #42028, #110326, #17337, #93510, #50444, #76177, #102462, #16782, #8403, #35276, #94068, #8965, #69461, #1144, #34720, #12270, #104134, #27420, #70020, #37487, #62164, #88982, #3361, #62734, #29626, #19000, #80040, #35837, #3909, #106340, #29089, #61603, #21194, #104685, #71691, #36926, #20124, #53773, #53200, #63810, #12825, #47005, #96855, #46462, #19567, #70567, #80595, #95736, #11735, #45904, #72218, #97927, #105809, #27979, #87340, #38038, #1696, #36378, #96290, #55404, #10636, #87909, #89536, #44804, #78957, #2264, #11198, #45362, #54316, #88445, #79501, #2808, #71123, #105244, #28535, #63274, #97385, #20656, #54858, #82789, #109115, #58159, #4974, #39118, #57622 ),
 .UNSPECIFIED., .F., .F.,
 ( 4, 3, 3, 3, 3, 3, 3, 3, 3, 3, 3, 3, 3, 3, 3, 3, 3, 3, 3, 3, 3, 3, 3, 3, 3, 3, 3, 3, 3, 3, 3, 3, 3, 3, 3, 3, 3, 3, 3, 3, 3, 3, 3, 3, 3, 3, 3, 3, 3, 3, 3, 3, 3, 3, 3, 3, 3, 3, 3, 3, 3, 3, 3, 3, 3, 3, 3, 3, 3, 3, 3, 3, 3, 3, 3, 3, 3, 3, 3, 3, 3, 3, 3, 3, 3, 3, 3, 3, 3, 3, 3, 3, 3, 3, 3, 3, 3, 3, 3, 3, 3, 4 ),
 ( 8.502096524649999765, 10.07864787959089981, 11.93479254620110019, 13.53107985676839853, 14.91300515749670019, 15.39383910900589925, 16.53746239350300229, 17.65458387737769996, 18.74843729357949940, 19.85248863406109976, 20.89822462007209936, 21.92896863737080082, 22.94591180423740084, 23.95008399577969982, 24.93651389660379891, 25.91373036143600217, 26.87743017290080161, 27.58084801743209979, 28.63657303752779981, 29.71534806165689702, 30.81785565885160239, 31.94355054423600038, 33.12499366665170442, 34.29034599565019903, 35.45679948715110186, 36.61536720514430243, 37.81029928474870161, 38.92267659857289885, 40.01573463098910111, 41.08144785925959752, 41.39509552356179967, 42.90409533963379829, 44.42240685342919448, 45.95641701915690192, 47.50713568527189778, 49.07569676298640360, 50.66338138030639726, 52.27164696925940035, 53.93007767069119751, 55.59733588536930426, 57.29035514786890104, 59.01163268845090215, 60.78223427696999437, 62.58432007834910138, 64.44189006276219800, 65.53909258071379895, 67.04466091477729606, 68.62874293280711413, 70.27935153705820426, 72.01713397602310351, 73.87821637511270012, 75.94820385017399644, 78.63691978283431183, 80.96957215551108789, 82.94440381128279682, 84.75275152858640126, 86.41315054547159491, 88.01530566766550123, 89.54414943656179560, 90.91108773666839227, 93.83029885312799934, 96.80610674239019886, 99.57495006331539855, 102.2152258246999992, 104.7433345856459965, 107.1773875570659982, 109.5324586405310043, 111.7902715113670098, 114.0014454456810000, 116.1495204710570022, 117.6367619672259934, 119.0972352214530048, 120.5529424179680262, 122.0399992496289912, 123.4355467568209832, 124.8016281987520131, 126.1383812957949999, 127.4470804953769942, 128.7157394665759966, 129.9643185484640071, 131.2068578098609919, 132.4493970712580335, 133.6732891993179919, 135.0123274964250015, 136.6169184369290122, 138.3144093969239918, 139.6958786578699971, 140.9759288702229867, 142.1124124449380020, 143.2059073724689995, 144.2494749791640061, 144.8160795072840017, 146.1144237599960150, 147.4424597893359987, 148.8129228152089922, 150.2046619519239812, 151.6094994080520166, 153.0694599465389842, 154.4582506042169996, 155.8279853376390065, 157.1656630716910001, 157.4493415620000007 ),
 .UNSPECIFIED. ) ;
#103297=FACE_OUTER_BOUND ( 'NONE', #8237, .T. ) ;
#103310=EDGE_CURVE ( 'NONE', #40014, #68662, #31480, .T. ) ;
#103332=VERTEX_POINT ( 'NONE', #15750 ) ;
#103335=( BOUNDED_CURVE ( )  B_SPLINE_CURVE ( 3, ( #92221, #74890, #8199, #93857 ),
 .UNSPECIFIED., .F., .F. ) 
 B_SPLINE_CURVE_WITH_KNOTS ( ( 4, 4 ),
 ( 1.431195359047013893, 1.487065270106493919 ),
 .UNSPECIFIED. ) 
 CURVE ( )  GEOMETRIC_REPRESENTATION_ITEM ( )  RATIONAL_B_SPLINE_CURVE ( ( 1.000000000000000000, 0.9997398963350896395, 0.9997398963350896395, 1.000000000000000000 ) ) 
 REPRESENTATION_ITEM ( '' )  );
#103340=CARTESIAN_POINT ( 'NONE',  ( -39.75532303620000363, 1384.581637800209819, 212.4630896483189701 ) ) ;
#103342=CARTESIAN_POINT ( 'NONE',  ( -55.77908735024080045, 1384.648364377080043, 235.3611123942870051 ) ) ;
#103353=CARTESIAN_POINT ( 'NONE',  ( -68.34315272460000301, 1379.747704235549918, 279.2339980437589588 ) ) ;
#103360=CARTESIAN_POINT ( 'NONE',  ( -36.10875963189999283, 1384.937915446980014, 235.4744139267589844 ) ) ;
#103362=CARTESIAN_POINT ( 'NONE',  ( -14.82755886204359896, 1385.295373219239991, 219.3747924830010163 ) ) ;
#103381=CARTESIAN_POINT ( 'NONE',  ( -109.1311031668469411, 1384.887895505450388, 311.2646947245262368 ) ) ;
#103397=CIRCLE ( 'NONE', #55180, 6.868727599660006788 ) ;
#103409=CARTESIAN_POINT ( 'NONE',  ( -71.81454634048201058, 1383.783546078690051, 296.7712788830790487 ) ) ;
#103412=CARTESIAN_POINT ( 'NONE',  ( -106.4020496450190052, 1391.913060387289988, 304.2007955189830568 ) ) ;
#103417=CARTESIAN_POINT ( 'NONE',  ( -79.42094436850000250, 1379.292317202809954, 292.9105207063590228 ) ) ;
#103428=CARTESIAN_POINT ( 'NONE',  ( -108.8600183350000066, 1381.954052101950083, 297.7238345936590349 ) ) ;
#103445=CARTESIAN_POINT ( 'NONE',  ( -119.8718586775641484, 1384.899971913130003, 299.5197653927721149 ) ) ;
#103448=CARTESIAN_POINT ( 'NONE',  ( -8.861333410889999485, 1384.870662623839962, 218.6848950059789729 ) ) ;
#103458=EDGE_LOOP ( 'NONE', ( #3968, #108461, #71931, #60750 ) ) ;
#103478=VERTEX_POINT ( 'NONE', #37553 ) ;
#103484=ORIENTED_EDGE ( 'NONE', *, *, #104226, .T. ) ;
#103492=CIRCLE ( 'NONE', #73073, 0.9999999999999992228 ) ;
#103509=CARTESIAN_POINT ( 'NONE',  ( -14.90483084879999964, 1391.000798919190174, 209.4215842360250122 ) ) ;
#103517=B_SPLINE_CURVE_WITH_KNOTS ( 'NONE', 5,
 ( #76460, #32795, #15979, #101090, #59676, #93788, #8689, #17063, #85393, #7053, #75381, #32068, #83025, #40464, #5780, #74091, #15246, #39922 ),
 .UNSPECIFIED., .F., .F.,
 ( 6, 3, 3, 3, 3, 6 ),
 ( -66.06417000470000289, -61.46700666819999981, -43.61786061130000292, -17.15566543539999600, 15.57237739079999983, 26.25296013780000237 ),
 .UNSPECIFIED. ) ;
#103542=DIRECTION ( 'NONE',  ( 1.439455173507210273E-14, 1.000000000000000000, 2.465190328815660140E-31 ) ) ;
#103561=CARTESIAN_POINT ( 'NONE',  ( -10.24092311318542059, 1389.890054110666142, 202.1840738160088620 ) ) ;
#103567=B_SPLINE_SURFACE_WITH_KNOTS ( 'NONE', 5, 3, ( 
 ( #106387, #80639, #108027, #4490 ),
 ( #30214, #3953, #81174, #72799 ),
 ( #3401, #106926, #73901, #64405 ),
 ( #39735, #98528, #21795, #31324 ),
 ( #88491, #105850, #90119, #81714 ),
 ( #73342, #107476, #48149, #54361 ),
 ( #82287, #11775, #65507, #86007 ),
 ( #17669, #51871, #32971, #66619 ),
 ( #66065, #22901, #82829, #9307 ),
 ( #32442, #92327, #74462, #103340 ),
 ( #35050, #24003, #31877, #57666 ),
 ( #60841, #58199, #7236, #78156 ),
 ( #99616, #67160, #49803, #75561 ),
 ( #57109, #41396, #1466, #108590 ),
 ( #6121, #109158, #100721, #91236 ),
 ( #60270, #101258, #14515, #48705 ),
 ( #6677, #40277, #43470, #94389 ),
 ( #77615, #26079, #15598, #91778 ),
 ( #100189, #23473, #927, #15056 ),
 ( #83935, #49255, #26643, #69231 ),
 ( #109696, #83376, #40831, #94966 ),
 ( #75008, #18235, #52430, #86556 ),
 ( #9852, #44020, #36715, #97719 ),
 ( #63067, #44573, #105023, #19337 ),
 ( #27212, #61393, #80926, #70907 ),
 ( #10403, #88778, #80379, #28316 ),
 ( #95514, #10966, #61949, #20440 ),
 ( #78718, #104463, #3695, #62507 ),
 ( #87113, #37823, #106126, #54649 ),
 ( #96628, #2034, #37274, #72009 ) ),
 .UNSPECIFIED., .F., .F., .F.,
 ( 6, 3, 3, 3, 3, 3, 3, 3, 3, 6 ),
 ( 4, 4 ),
 ( 0.000000000000000000, 15.39383910899999997, 27.58084801740000103, 41.39509552349999666, 65.53909258059999843, 90.91108773649999364, 117.6367619669999982, 132.4493970709999928, 144.8160795070000120, 161.8240513320000105 ),
 ( 33.63253214979999939, 34.48604544350000367 ),
 .UNSPECIFIED. ) ;
#103569=CARTESIAN_POINT ( 'NONE',  ( -12.84953875605850016, 1390.894593418380055, 209.7715853971660067 ) ) ;
#103578=CARTESIAN_POINT ( 'NONE',  ( -82.48023544352470537, 1385.167086914460015, 286.1466225573760198 ) ) ;
#103580=CARTESIAN_POINT ( 'NONE',  ( -56.64534719470000113, 1379.747652096109960, 254.3393773118589536 ) ) ;
#103621=CIRCLE ( 'NONE', #32088, 2.000007659174134922 ) ;
#103623=CARTESIAN_POINT ( 'NONE',  ( -14.15592233437959990, 1379.713028150099944, 208.2740576972960014 ) ) ;
#103627=ORIENTED_EDGE ( 'NONE', *, *, #38350, .F. ) ;
#103645=CARTESIAN_POINT ( 'NONE',  ( -97.83172781913290805, 1384.867102923100219, 295.7948235560999706 ) ) ;
#103653=ORIENTED_EDGE ( 'NONE', *, *, #108224, .T. ) ;
#103663=CARTESIAN_POINT ( 'NONE',  ( -18.81083778160000008, 1379.661349286479890, 209.0395301435680153 ) ) ;
#103707=CARTESIAN_POINT ( 'NONE',  ( -8.751535168777641260, 1384.847616307870112, 220.6818258576190033 ) ) ;
#103716=CARTESIAN_POINT ( 'NONE',  ( -71.28397327874120037, 1384.659025300439907, 296.4637328428320302 ) ) ;
#103724=CARTESIAN_POINT ( 'NONE',  ( -9.094692777799998851, 1384.940603055749989, 199.9428207063789955 ) ) ;
#103733=CARTESIAN_POINT ( 'NONE',  ( -106.4363417272620040, 1391.913060387289988, 304.7483998906039915 ) ) ;
#103737=CARTESIAN_POINT ( 'NONE',  ( -9.052531689720000330, 1381.507819611680134, 200.6139546878390263 ) ) ;
#103749=AXIS2_PLACEMENT_3D ( 'NONE', #53065, #26169, #78807 ) ;
#103752=CARTESIAN_POINT ( 'NONE',  ( -64.31310606715069866, 1379.736843722260119, 273.6487788150259917 ) ) ;
#103753=ORIENTED_EDGE ( 'NONE', *, *, #28360, .F. ) ;
#103777=ORIENTED_EDGE ( 'NONE', *, *, #89465, .T. ) ;
#103787=CARTESIAN_POINT ( 'NONE',  ( -49.28052484613377260, 1379.685954563121641, 238.1922399297049537 ) ) ;
#103794=CARTESIAN_POINT ( 'NONE',  ( -103.6155712370580062, 1379.922240051319932, 305.0844860589629661 ) ) ;
#103804=CARTESIAN_POINT ( 'NONE',  ( -96.24750340660000347, 1384.324597676740041, 310.5510276952589948 ) ) ;
#103807=DIRECTION ( 'NONE',  ( -3.237679667471999896E-17, -1.000000000000000000, -6.999474336859099157E-17 ) ) ;
#103815=CARTESIAN_POINT ( 'NONE',  ( -83.35163594419999811, 1388.281121046439921, 288.8577119767590489 ) ) ;
#103826=CARTESIAN_POINT ( 'NONE',  ( -108.6610895849279927, 1383.759820234390190, 311.0754968279820218 ) ) ;
#103853=CARTESIAN_POINT ( 'NONE',  ( -15.09720442233679805, 1384.876713416460007, 219.4545074913159795 ) ) ;
#103874=CARTESIAN_POINT ( 'NONE',  ( -113.4000000000000057, 1377.020218211860083, 306.8927966156020375 ) ) ;
#103883=CARTESIAN_POINT ( 'NONE',  ( -110.0629314620319974, 1384.917035430780061, 296.9512851041370141 ) ) ;
#103906=CARTESIAN_POINT ( 'NONE',  ( -65.41103462389999379, 1377.321258373460068, 268.8604125841590076 ) ) ;
#103907=TOROIDAL_SURFACE ( 'NONE', #28789, 6.868727599660000571, 1.000000000000000000 ) ;
#103908=CARTESIAN_POINT ( 'NONE',  ( -106.4561910723670053, 1378.913060387289988, 301.9552841335789708 ) ) ;
#103913=CARTESIAN_POINT ( 'NONE',  ( -66.58891394985930390, 1384.715272088890060, 258.5866899849719971 ) ) ;
#103925=CARTESIAN_POINT ( 'NONE',  ( -68.64142316320000248, 1379.747636946170132, 279.8413332628590524 ) ) ;
#103933=CARTESIAN_POINT ( 'NONE',  ( -47.37590574939999755, 1384.752751010099928, 256.2773158601589785 ) ) ;
#103954=FACE_OUTER_BOUND ( 'NONE', #97711, .T. ) ;
#103962=CARTESIAN_POINT ( 'NONE',  ( -14.47191459792289869, 1379.648775954749908, 208.1784578746709826 ) ) ;
#103978=CARTESIAN_POINT ( 'NONE',  ( -99.87664611743339549, 1383.764086582540131, 310.6354922946979968 ) ) ;
#103979=CARTESIAN_POINT ( 'NONE',  ( -109.9700156609570030, 1384.452758312609831, 311.4358946100080061 ) ) ;
#103985=CARTESIAN_POINT ( 'NONE',  ( -84.09514530399998478, 1383.332197241610174, 288.0930448863589959 ) ) ;
#103995=CARTESIAN_POINT ( 'NONE',  ( -109.1848878950000028, 1384.511724394249995, 297.1380044401590226 ) ) ;
#104057=CARTESIAN_POINT ( 'NONE',  ( -11.35998449626690032, 1391.913060387289988, 207.0982575650849924 ) ) ;
#104068=CARTESIAN_POINT ( 'NONE',  ( -16.33138198470000191, 1386.615434968630098, 200.5875628059090161 ) ) ;
#104069=CARTESIAN_POINT ( 'NONE',  ( -14.10024896163066188, 1390.294839404160484, 211.8274166821641984 ) ) ;
#104078=CARTESIAN_POINT ( 'NONE',  ( -8.834712661419999336, 1383.770682883139898, 218.4951700419789802 ) ) ;
#104109=CARTESIAN_POINT ( 'NONE',  ( -19.53142348151149932, 1383.854072636070214, 220.5763941096860208 ) ) ;
#104118=CARTESIAN_POINT ( 'NONE',  ( -10.11238584568503462, 1389.734820954164434, 201.9902729080233996 ) ) ;
#104125=CARTESIAN_POINT ( 'NONE',  ( -14.49971677770000156, 1379.923539855790068, 208.5574997035849947 ) ) ;
#104128=EDGE_CURVE ( 'NONE', #40412, #101907, #83840, .T. ) ;
#104133=CARTESIAN_POINT ( 'NONE',  ( -10.53295592549999959, 1391.913060387289988, 204.1405351054689845 ) ) ;
#104134=CARTESIAN_POINT ( 'NONE',  ( -87.47238879921440002, 1385.184608911460145, 290.8447695388430247 ) ) ;
#104158=DIRECTION ( 'NONE',  ( 0.05030786423734002338, 0.002305672611446700927, 0.9987310962765134636 ) ) ;
#104184=B_SPLINE_CURVE_WITH_KNOTS ( 'NONE', 5,
 ( #29676, #30778, #100194, #91783, #65511, #81178, #22905, #15060, #56000 ),
 .UNSPECIFIED., .F., .F.,
 ( 6, 3, 6 ),
 ( 0.000000000000000000, 0.5456913010464850000, 1.000000000000000000 ),
 .UNSPECIFIED. ) ;
#104202=EDGE_CURVE ( 'NONE', #41641, #52311, #11401, .T. ) ;
#104212=CARTESIAN_POINT ( 'NONE',  ( -109.9438493645591990, 1383.878411725401293, 297.0368449378275386 ) ) ;
#104214=CARTESIAN_POINT ( 'NONE',  ( -16.47481425009999967, 1379.657961281789767, 208.5229944698799898 ) ) ;
#104218=CARTESIAN_POINT ( 'NONE',  ( -68.50706126866759860, 1379.747743051572343, 280.0840774304766683 ) ) ;
#104226=EDGE_CURVE ( 'NONE', #33840, #35724, #76829, .T. ) ;
#104252=CARTESIAN_POINT ( 'NONE',  ( -12.28856626983460032, 1377.626870450839988, 208.3294650349379822 ) ) ;
#104259=CARTESIAN_POINT ( 'NONE',  ( -7.557748306139269623, 1384.394157022499940, 219.0612169397370224 ) ) ;
#104267=CARTESIAN_POINT ( 'NONE',  ( 2.375285482014719999E-15, 1391.913060387289988, 209.1218459572589836 ) ) ;
#104273=CARTESIAN_POINT ( 'NONE',  ( -62.63025033776229122, 1384.685893630349938, 285.2374344412770029 ) ) ;
#104275=CARTESIAN_POINT ( 'NONE',  ( -18.05670876470880160, 1384.947303455109932, 201.1907562702159851 ) ) ;
#104281=FACE_OUTER_BOUND ( 'NONE', #91381, .T. ) ;
#104286=CARTESIAN_POINT ( 'NONE',  ( -106.4029571836669987, 1391.913060387289988, 304.3198526369590127 ) ) ;
#104292=CARTESIAN_POINT ( 'NONE',  ( -8.672272362719999350, 1384.150546597180210, 199.9472511214389954 ) ) ;
#104303=CARTESIAN_POINT ( 'NONE',  ( -59.60612636626729710, 1379.726987694469926, 264.7824669088110454 ) ) ;
#104310=CARTESIAN_POINT ( 'NONE',  ( -109.3078499810000039, 1384.937516855040030, 311.2645914332589427 ) ) ;
#104315=CARTESIAN_POINT ( 'NONE',  ( -105.7942479044789934, 1378.913060387259975, 304.2294709827049815 ) ) ;
#104334=CARTESIAN_POINT ( 'NONE',  ( -58.69971502816261477, 1379.720317519436549, 258.4395855553975707 ) ) ;
#104347=CARTESIAN_POINT ( 'NONE',  ( -46.84911848401252144, 1379.681085501543976, 239.8728125796529298 ) ) ;
#104362=CARTESIAN_POINT ( 'NONE',  ( -87.55914429599999949, 1389.463764338810051, 294.7984051320589742 ) ) ;
#104376=CARTESIAN_POINT ( 'NONE',  ( -105.4614100663400080, 1378.948680768060058, 305.4850396033990023 ) ) ;
#104397=TOROIDAL_SURFACE ( 'NONE', #66852, 11.99982860380000105, 0.5000000000000000000 ) ;
#104405=CARTESIAN_POINT ( 'NONE',  ( -16.53951191381450059, 1384.872637633759950, 219.7923600667549806 ) ) ;
#104423=CARTESIAN_POINT ( 'NONE',  ( -109.9853818454200081, 1384.675995219419974, 311.4496462838500292 ) ) ;
#104429=CARTESIAN_POINT ( 'NONE',  ( -109.5441724319999963, 1378.085199107079916, 306.7703179349799711 ) ) ;
#104458=CARTESIAN_POINT ( 'NONE',  ( -72.27662900180000349, 1374.712643069990008, 284.7775436206590598 ) ) ;
#104459=CARTESIAN_POINT ( 'NONE',  ( -105.9291394038200025, 1378.913060387309770, 303.1458921680629715 ) ) ;
#104463=CARTESIAN_POINT ( 'NONE',  ( -106.7755317029999986, 1385.123395227499941, 297.1212035911590306 ) ) ;
#104464=CARTESIAN_POINT ( 'NONE',  ( -52.23400470469020007, 1384.630035204419983, 228.9130027668180105 ) ) ;
#104469=DIRECTION ( 'NONE',  ( -1.836970198721029688E-16, -1.000000000000000000, 0.000000000000000000 ) ) ;
#104472=CARTESIAN_POINT ( 'NONE',  ( -8.746836412960000473, 1384.203074880319946, 218.5235076343190030 ) ) ;
#104477=CARTESIAN_POINT ( 'NONE',  ( -66.59180496469998900, 1379.743803986980083, 275.7189149213589872 ) ) ;
#104487=CARTESIAN_POINT ( 'NONE',  ( -17.46768317430000295, 1384.870099884450156, 219.9576826991589940 ) ) ;
#104489=CARTESIAN_POINT ( 'NONE',  ( -19.48484630070749901, 1385.278268516279923, 220.7194127531260222 ) ) ;
#104501=CARTESIAN_POINT ( 'NONE',  ( -5.858855997866009524, 1391.912605642699873, 215.0838203321740139 ) ) ;
#104502=CARTESIAN_POINT ( 'NONE',  ( -107.4307047400000101, 1391.913060387289988, 300.8770155100590387 ) ) ;
#104536=CARTESIAN_POINT ( 'NONE',  ( -88.49165759785731211, 1383.771278392089926, 307.9869884267500311 ) ) ;
#104537=CARTESIAN_POINT ( 'NONE',  ( -109.9093271260659890, 1384.056711624799846, 311.3953200952379348 ) ) ;
#104542=ORIENTED_EDGE ( 'NONE', *, *, #12582, .T. ) ;
#104544=CARTESIAN_POINT ( 'NONE',  ( -69.46418562150000753, 1379.235091224930102, 280.3187033645589850 ) ) ;
#104553=AXIS2_PLACEMENT_3D ( 'NONE', #95533, #28334, #60288 ) ;
#104555=CARTESIAN_POINT ( 'NONE',  ( -109.8932579119999957, 1384.895258862230094, 297.0235774065590135 ) ) ;
#104625=CARTESIAN_POINT ( 'NONE',  ( -37.21633441560000222, 1384.983113612510124, 210.1703949109789846 ) ) ;
#104633=CARTESIAN_POINT ( 'NONE',  ( -9.454895823979999392, 1382.479201248260097, 217.9319156271789950 ) ) ;
#104661=CARTESIAN_POINT ( 'NONE',  ( -35.92588528242170298, 1383.834180000839979, 235.2311359915490243 ) ) ;
#104662=VECTOR ( 'NONE', #31482, 1000.000000000000000 ) ;
#104671=CARTESIAN_POINT ( 'NONE',  ( -8.467296363548342697, 1387.234424845827334, 200.0078932864855972 ) ) ;
#104677=CARTESIAN_POINT ( 'NONE',  ( -14.10038679502460113, 1390.294844427760154, 211.8274118880190144 ) ) ;
#104685=CARTESIAN_POINT ( 'NONE',  ( -92.29530878936199656, 1385.199744097189978, 293.8198967544350353 ) ) ;
#104686=CARTESIAN_POINT ( 'NONE',  ( -10.01339882083300026, 1391.913060387289988, 214.4629424297139906 ) ) ;
#104745=CARTESIAN_POINT ( 'NONE',  ( -12.06139973099999985, 1391.856450693919896, 210.3499673627589743 ) ) ;
#104748=ORIENTED_EDGE ( 'NONE', *, *, #15882, .F. ) ;
#104763=CARTESIAN_POINT ( 'NONE',  ( -103.5631853459999974, 1389.967198823729859, 302.9633942972590148 ) ) ;
#104764=CARTESIAN_POINT ( 'NONE',  ( -109.7827413208553509, 1383.386978333693150, 297.1311717743816416 ) ) ;
#104767=CARTESIAN_POINT ( 'NONE',  ( -42.07298630380000048, 1379.652797345190265, 226.0105342722590080 ) ) ;
#104777=CARTESIAN_POINT ( 'NONE',  ( -68.78023285115449426, 1385.028536229589918, 293.6602838790100236 ) ) ;
#104791=DIRECTION ( 'NONE',  ( -0.009376423277032341561, 0.9999478196825741794, -0.004054700802289810599 ) ) ;
#104802=CARTESIAN_POINT ( 'NONE',  ( -10.67458942334280003, 1390.939239166159950, 215.3172498179779666 ) ) ;
#104824=CARTESIAN_POINT ( 'NONE',  ( -79.14789062195450242, 1384.640371133850067, 303.2828232109690134 ) ) ;
#104825=CARTESIAN_POINT ( 'NONE',  ( -28.80985028338039911, 1384.966547565240262, 204.9440933951439945 ) ) ;
#104839=CARTESIAN_POINT ( 'NONE',  ( -106.8184672166400020, 1391.913060387289988, 306.2514081895690197 ) ) ;
#104855=CARTESIAN_POINT ( 'NONE',  ( -67.11452714873080083, 1379.744023253179876, 278.1888607204630262 ) ) ;
#104860=CARTESIAN_POINT ( 'NONE',  ( -105.6288035359999924, 1378.913058700080001, 304.0441401731590076 ) ) ;
#104868=CARTESIAN_POINT ( 'NONE',  ( -106.0563520787330134, 1378.913060388819986, 305.4990271455400261 ) ) ;
#104885=CARTESIAN_POINT ( 'NONE',  ( -8.297843638769998975, 1384.899870798449911, 218.7036046513889858 ) ) ;
#104889=CARTESIAN_POINT ( 'NONE',  ( -59.11373648366758715, 1379.721719983604544, 259.3782992626888131 ) ) ;
#104901=CARTESIAN_POINT ( 'NONE',  ( -45.22866404258923012, 1379.675374582019685, 237.0192218885333659 ) ) ;
#104923=CARTESIAN_POINT ( 'NONE',  ( -103.2203533160000006, 1390.533826207339871, 304.2968465863590382 ) ) ;
#104934=CARTESIAN_POINT ( 'NONE',  ( -106.5378846238329942, 1381.285095380909979, 309.2529097667930387 ) ) ;
#104952=APPLICATION_CONTEXT ( 'automotive_design' ) ;
#104958=CARTESIAN_POINT ( 'NONE',  ( -14.82216926960470182, 1384.877475996390103, 219.3981822003099751 ) ) ;
#104983=CARTESIAN_POINT ( 'NONE',  ( -54.29131571383740607, 1379.936403459110124, 253.6537993308690204 ) ) ;
#104992=CARTESIAN_POINT ( 'NONE',  ( -8.066920486049999894, 1384.201370995469915, 218.7301529432190250 ) ) ;
#105019=CARTESIAN_POINT ( 'NONE',  ( -101.9775983549999978, 1375.414493452870147, 301.8221755499590699 ) ) ;
#105020=CARTESIAN_POINT ( 'NONE',  ( -105.9034084253929962, 1378.913060387329779, 303.2380501759690219 ) ) ;
#105023=CARTESIAN_POINT ( 'NONE',  ( -92.78539381950000120, 1384.966825520919883, 294.1434271777590084 ) ) ;
#105038=CARTESIAN_POINT ( 'NONE',  ( -68.02027221699999870, 1379.746446890080051, 278.4719343715589730 ) ) ;
#105047=CARTESIAN_POINT ( 'NONE',  ( -49.58793988690000276, 1384.741903095260113, 260.9101892837590526 ) ) ;
#105049=CARTESIAN_POINT ( 'NONE',  ( -21.77341892320420058, 1385.269227909690017, 221.7389472576159903 ) ) ;
#105092=CARTESIAN_POINT ( 'NONE',  ( -81.76652289506799320, 1383.775734044670116, 304.7570926416640305 ) ) ;
#105094=CARTESIAN_POINT ( 'NONE',  ( -109.5071830355930018, 1383.951130388469892, 311.2194437626960166 ) ) ;
#105100=CARTESIAN_POINT ( 'NONE',  ( -92.77130722430000276, 1383.377570089289748, 294.1770395593590024 ) ) ;
#105105=CARTESIAN_POINT ( 'NONE',  ( -109.5353424460000014, 1384.935512065160083, 297.1231347603589938 ) ) ;
#105177=VERTEX_POINT ( 'NONE', #68047 ) ;
#105184=CARTESIAN_POINT ( 'NONE',  ( -20.57369194309999827, 1389.799942534980119, 216.9804166070690030 ) ) ;
#105185=CARTESIAN_POINT ( 'NONE',  ( -12.25810126567743907, 1388.996058220885516, 215.8687261311177963 ) ) ;
#105223=CARTESIAN_POINT ( 'NONE',  ( -27.09553561796830223, 1383.845623832669844, 225.0950745557760229 ) ) ;
#105231=CARTESIAN_POINT ( 'NONE',  ( -3.078458350170000024, 1381.390032981420063, 201.0850095095790095 ) ) ;
#105237=CARTESIAN_POINT ( 'NONE',  ( -9.537890462841289718, 1388.022264309169941, 217.5086179808309907 ) ) ;
#105244=CARTESIAN_POINT ( 'NONE',  ( -105.5431657123439919, 1385.234305881529963, 296.9663787050429846 ) ) ;
#105267=CARTESIAN_POINT ( 'NONE',  ( -103.9362963259999901, 1380.106856784760112, 301.6745611782590117 ) ) ;
#105314=CARTESIAN_POINT ( 'NONE',  ( -103.8055019550000111, 1389.814814112089834, 301.7479020532589971 ) ) ;
#105321=CARTESIAN_POINT ( 'NONE',  ( -63.34523448917954624, 1379.747030511724688, 271.7626510979175123 ) ) ;
#105328=CARTESIAN_POINT ( 'NONE',  ( -70.89913272470511174, 1385.021051334530057, 296.0640616977649984 ) ) ;
#105357=CARTESIAN_POINT ( 'NONE',  ( -14.17818885755020020, 1379.591559934480074, 207.8207570064110143 ) ) ;
#105365=CARTESIAN_POINT ( 'NONE',  ( -7.544733521240000407, 1384.899971913130003, 219.0877090842990071 ) ) ;
#105382=CARTESIAN_POINT ( 'NONE',  ( -97.12056875041480453, 1384.606167604229995, 310.4282471984710128 ) ) ;
#105383=CARTESIAN_POINT ( 'NONE',  ( -47.06618458142209249, 1385.009314242649907, 220.9877181434370073 ) ) ;
#105384=CARTESIAN_POINT ( 'NONE',  ( -5.014111827051360493, 1375.346567646530048, 214.7183233550310320 ) ) ;
#105394=CARTESIAN_POINT ( 'NONE',  ( -106.6593330254749930, 1391.913060387289988, 305.7868564143699928 ) ) ;
#105395=B_SPLINE_CURVE_WITH_KNOTS ( 'NONE', 5,
 ( #1662, #95704, #79465, #11166, #80007, #53741 ),
 .UNSPECIFIED., .F., .F.,
 ( 6, 6 ),
 ( 0.000000000000000000, 1.000000000000000000 ),
 .UNSPECIFIED. ) ;
#105399=CARTESIAN_POINT ( 'NONE',  ( -12.96458870010000020, 1380.564911143250129, 203.9320203105589826 ) ) ;
#105411=CARTESIAN_POINT ( 'NONE',  ( -68.05606538682749829, 1379.746262163739857, 279.5397730745099807 ) ) ;
#105445=CARTESIAN_POINT ( 'NONE',  ( -63.17697519130717154, 1379.734402953275776, 268.4289174494917916 ) ) ;
#105456=CARTESIAN_POINT ( 'NONE',  ( -57.46991821550079749, 1379.718150813474040, 260.7768847105036230 ) ) ;
#105476=CARTESIAN_POINT ( 'NONE',  ( -113.4000000000000057, 1390.498795466600086, 304.4869478500590390 ) ) ;
#105488=CARTESIAN_POINT ( 'NONE',  ( -104.7456079307379895, 1380.506914483850096, 307.5456015192170298 ) ) ;
#105495=ADVANCED_FACE ( 'NONE', ( #9082 ), #39230, .T. ) ;
#105517=CARTESIAN_POINT ( 'NONE',  ( -37.64110078237469992, 1384.797974306949982, 238.1784615367210165 ) ) ;
#105544=CARTESIAN_POINT ( 'NONE',  ( -55.53609276739749845, 1378.543823089900116, 260.2783981610180035 ) ) ;
#105555=CARTESIAN_POINT ( 'NONE',  ( -8.032185305569999656, 1384.475430595510034, 218.7662459373489980 ) ) ;
#105579=CARTESIAN_POINT ( 'NONE',  ( -88.45813511300001153, 1375.507175221300258, 298.0129420291590350 ) ) ;
#105582=CARTESIAN_POINT ( 'NONE',  ( -105.8445521485040075, 1378.913060387460064, 303.5212775329050032 ) ) ;
#105600=CARTESIAN_POINT ( 'NONE',  ( -65.86513797469999076, 1379.742265928139886, 274.2610620464590170 ) ) ;
#105608=CARTESIAN_POINT ( 'NONE',  ( -102.7364941740000006, 1384.940050820800025, 311.2335147922589726 ) ) ;
#105610=CARTESIAN_POINT ( 'NONE',  ( -36.74521059231790332, 1385.199967091270082, 236.7483831902960105 ) ) ;
#105633=AXIS2_PLACEMENT_3D ( 'NONE', #82482, #20899, #106038 ) ;
#105659=CARTESIAN_POINT ( 'NONE',  ( -77.25135237149000034, 1383.779025680539917, 301.6761197000710126 ) ) ;
#105660=CARTESIAN_POINT ( 'NONE',  ( -109.1401334702460133, 1384.096248926530052, 311.1747910708369886 ) ) ;
#105666=CARTESIAN_POINT ( 'NONE',  ( -88.44418928299998583, 1380.083824802999970, 304.2210320317589662 ) ) ;
#105696=CLOSED_SHELL ( 'NONE', ( #46609, #54994, #62697, #13313, #34357, #58981, #56614, #100886, #105495, #58502, #44028, #79553, #842, #34547, #29827, #7946, #40190, #100161, #76027, #69259, #99962, #37377, #20710, #38442, #30413, #52030, #1456, #65178, #60415, #37136, #89787, #109662, #6533, #87303, #30437, #25578, #33563, #98784, #86447, #737, #26985, #41420, #61198, #45267, #27487, #6489, #37513, #87108, #38583, #86352, #11081, #85658, #109215, #39149, #101268, #7598, #392, #66764, #86254, #18714, #45980, #11969, #69520, #46733, #76973, #91984, #11925, #2259, #98790, #3011, #63023, #45011, #49648, #73254, #22017, #74186, #28990, #19289, #79609, #82680, #67383, #3296, #17366 ) ) ;
#105747=CARTESIAN_POINT ( 'NONE',  ( -38.50281909529999780, 1385.190821792449924, 239.3058332809590070 ) ) ;
#105778=DIRECTION ( 'NONE',  ( -1.000000000000000000, 0.000000000000000000, 0.000000000000000000 ) ) ;
#105785=CARTESIAN_POINT ( 'NONE',  ( -23.21699021137670016, 1383.850094297019950, 222.3556410448979932 ) ) ;
#105794=CARTESIAN_POINT ( 'NONE',  ( -9.222898088157986507, 1388.549295314689516, 200.8262261746918114 ) ) ;
#105801=CARTESIAN_POINT ( 'NONE',  ( -10.63240336516950002, 1387.911495707119911, 217.3146354632350210 ) ) ;
#105809=CARTESIAN_POINT ( 'NONE',  ( -97.97442128001588912, 1385.215631988479799, 295.8423678355109701 ) ) ;
#105812=CARTESIAN_POINT ( 'NONE',  ( -68.67274465469999711, 1379.748163774529985, 279.9618448723590518 ) ) ;
#105829=CARTESIAN_POINT ( 'NONE',  ( -8.315526934679999371, 1385.338042180710090, 218.6773504991989796 ) ) ;
#105850=CARTESIAN_POINT ( 'NONE',  ( -16.33316124910000156, 1384.804537353890055, 200.5738954341890121 ) ) ;
#105859=EDGE_LOOP ( 'NONE', ( #98400, #16435, #81263, #40434, #53207, #18682, #37142, #96995 ) ) ;
#105881=CARTESIAN_POINT ( 'NONE',  ( -105.5476282266839974, 1391.479847970690116, 304.9206647878619947 ) ) ;
#105885=VERTEX_POINT ( 'NONE', #99695 ) ;
#105890=CARTESIAN_POINT ( 'NONE',  ( -59.61868368084140002, 1385.068020327440081, 280.3090023487520170 ) ) ;
#105891=CARTESIAN_POINT ( 'NONE',  ( -8.888758267720000106, 1385.314821192629779, 218.6605176881890031 ) ) ;
#105894=AXIS2_PLACEMENT_3D ( 'NONE', #58458, #15857, #67980 ) ;
#105917=CARTESIAN_POINT ( 'NONE',  ( -12.28062996578079868, 1378.241810724349989, 208.0559987543549880 ) ) ;
#105926=CARTESIAN_POINT ( 'NONE',  ( -7.551930971255839786, 1384.476535447399783, 219.0683411548229742 ) ) ;
#105936=CARTESIAN_POINT ( 'NONE',  ( -12.31949146158819985, 1378.253793448930082, 209.5105130821430066 ) ) ;
#105942=CARTESIAN_POINT ( 'NONE',  ( -31.77495577332650001, 1384.972186697860025, 206.5720684459180063 ) ) ;
#105948=ORIENTED_EDGE ( 'NONE', *, *, #38350, .T. ) ;
#105949=CARTESIAN_POINT ( 'NONE',  ( -109.6574261609999894, 1384.907292521180125, 311.3230475462589766 ) ) ;
#105972=CARTESIAN_POINT ( 'NONE',  ( -67.34501255021619670, 1379.744579630669932, 278.5325692663910218 ) ) ;
#105977=CARTESIAN_POINT ( 'NONE',  ( -105.0454790209999913, 1379.237143502780100, 304.6380415787589868 ) ) ;
#105978=CARTESIAN_POINT ( 'NONE',  ( -109.1320112420000044, 1384.953741877089897, 311.2644403302589353 ) ) ;
#105979=SHAPE_REPRESENTATION ( 'Crank Arm', ( #21632 ), #46788 ) ;
#105999=CARTESIAN_POINT ( 'NONE',  ( -8.023395094369998759, 1384.908845605290026, 218.7875321875989982 ) ) ;
#106002=CARTESIAN_POINT ( 'NONE',  ( -63.87106590895305658, 1379.736345038605350, 269.9222812701415251 ) ) ;
#106038=DIRECTION ( 'NONE',  ( 0.03206272707449610987, 0.004242270441052224499, 0.9994768554969400975 ) ) ;
#106042=CARTESIAN_POINT ( 'NONE',  ( -105.7945529881810103, 1378.894406107679970, 306.4862516817319715 ) ) ;
#106063=CARTESIAN_POINT ( 'NONE',  ( -40.87587467545650100, 1384.783584316470069, 243.6885206019040027 ) ) ;
#106070=EDGE_LOOP ( 'NONE', ( #101548, #101417, #105948, #90801, #74604 ) ) ;
#106085=CARTESIAN_POINT ( 'NONE',  ( -50.14845714630110507, 1380.010081755269994, 242.5009527263639768 ) ) ;
#106095=CARTESIAN_POINT ( 'NONE',  ( -8.018637776459998534, 1384.752548399070065, 218.7860119703690032 ) ) ;
#106118=CARTESIAN_POINT ( 'NONE',  ( -87.43041093610000303, 1374.577971548089863, 299.9734862988590294 ) ) ;
#106126=CARTESIAN_POINT ( 'NONE',  ( -109.9987473190000031, 1385.017600419090058, 297.1692069989590550 ) ) ;
#106137=CARTESIAN_POINT ( 'NONE',  ( -67.47186131060000491, 1379.745269727820187, 277.3594581318590144 ) ) ;
#106147=CARTESIAN_POINT ( 'NONE',  ( -109.9987472809999929, 1384.694936393889975, 311.2694678342589896 ) ) ;
#106149=CARTESIAN_POINT ( 'NONE',  ( -20.12001630530539842, 1385.275803444980056, 220.9734419276739743 ) ) ;
#106179=ORIENTED_EDGE ( 'NONE', *, *, #106886, .F. ) ;
#106192=CARTESIAN_POINT ( 'NONE',  ( -90.89540613257170776, 1383.769753454369948, 308.8054560215319952 ) ) ;
#106193=CARTESIAN_POINT ( 'NONE',  ( -109.9358763820779927, 1384.187282608590067, 311.4119166190040460 ) ) ;
#106197=CARTESIAN_POINT ( 'NONE',  ( -97.71463903750000668, 1379.367587121119868, 302.5561533006589912 ) ) ;
#106202=CARTESIAN_POINT ( 'NONE',  ( -109.8947400899999991, 1384.917309675210163, 297.0284544140590128 ) ) ;
#106252=CARTESIAN_POINT ( 'NONE',  ( -24.94190653805079805, 1384.544460101560162, 203.2666405366809954 ) ) ;
#106279=CARTESIAN_POINT ( 'NONE',  ( -9.122696901847419326, 1384.513827595119892, 199.9705375801759999 ) ) ;
#106283=CARTESIAN_POINT ( 'NONE',  ( -14.08191331708516358, 1379.630701899112864, 211.6533031874265873 ) ) ;
#106314=CARTESIAN_POINT ( 'NONE',  ( -5.013435694540000043, 1375.426148861440197, 214.7180213005390215 ) ) ;
#106316=CARTESIAN_POINT ( 'NONE',  ( -28.27275148466259935, 1383.844209727440102, 226.1197677515999942 ) ) ;
#106326=CARTESIAN_POINT ( 'NONE',  ( -30.57150941279999756, 1379.881520546990032, 222.4328286988589980 ) ) ;
#106332=CARTESIAN_POINT ( 'NONE',  ( -9.567963333730000741, 1388.728411291870088, 217.1955492302289770 ) ) ;
#106340=CARTESIAN_POINT ( 'NONE',  ( -90.92127573589050371, 1385.195597713360030, 293.1101517920880042 ) ) ;
#106342=CARTESIAN_POINT ( 'NONE',  ( -68.74147317429999759, 1379.748081684489989, 280.1371050876589948 ) ) ;
#106345=ORIENTED_EDGE ( 'NONE', *, *, #81894, .T. ) ;
#106358=EDGE_CURVE ( 'NONE', #7780, #40166, #50133, .T. ) ;
#106359=CARTESIAN_POINT ( 'NONE',  ( 1.715743480078970019E-15, 1374.913060387289988, 209.1218459572589836 ) ) ;
#106363=CARTESIAN_POINT ( 'NONE',  ( -8.871284928439999717, 1385.205931087319868, 218.6719299737089841 ) ) ;
#106387=CARTESIAN_POINT ( 'NONE',  ( -1.973729821559999912E-15, 1384.913060387289988, 199.6218459572590120 ) ) ;
#106412=CARTESIAN_POINT ( 'NONE',  ( -108.2039566672529958, 1378.913060387289988, 299.7295690038039879 ) ) ;
#106420=CARTESIAN_POINT ( 'NONE',  ( -57.01644491674332471, 1379.744987729992772, 259.4421383630754576 ) ) ;
#106427=CARTESIAN_POINT ( 'NONE',  ( -86.82655498892479784, 1384.976974444049802, 307.5220928825150395 ) ) ;
#106473=CARTESIAN_POINT ( 'NONE',  ( -94.45993641895300641, 1384.611044289900065, 309.9217182750660413 ) ) ;
#106474=CARTESIAN_POINT ( 'NONE',  ( -30.26357380513479711, 1384.969279520580130, 205.7050507507260022 ) ) ;
#106494=CARTESIAN_POINT ( 'NONE',  ( -13.26994390069999952, 1379.834384431509989, 206.1416992256990000 ) ) ;
#106495=CARTESIAN_POINT ( 'NONE',  ( -10.49767883750000053, 1382.256743515189783, 217.7001910593189677 ) ) ;
#106504=CARTESIAN_POINT ( 'NONE',  ( -68.29979175837739547, 1379.746978049359996, 279.8462751379269662 ) ) ;
#106511=CARTESIAN_POINT ( 'NONE',  ( -109.9852357310000031, 1384.922450477979964, 311.4561609882589437 ) ) ;
#106524=VERTEX_POINT ( 'NONE', #76192 ) ;
#106535=CARTESIAN_POINT ( 'NONE',  ( -67.62101597386647711, 1379.745593051518881, 277.6608951446080482 ) ) ;
#106540=CARTESIAN_POINT ( 'NONE',  ( -63.26676713937528973, 1384.693636663830148, 251.1880306028709811 ) ) ;
#106545=B_SPLINE_CURVE_WITH_KNOTS ( 'NONE', 5,
 ( #107143, #32093, #29880, #22002, #30435, #15270 ),
 .UNSPECIFIED., .F., .F.,
 ( 6, 6 ),
 ( 1.385794409258260110E-07, 0.5294135995224299451 ),
 .UNSPECIFIED. ) ;
#106550=CARTESIAN_POINT ( 'NONE',  ( -108.8494111198608323, 1383.998126889661307, 311.1481491610576882 ) ) ;
#106569=CARTESIAN_POINT ( 'NONE',  ( -103.7369032989999909, 1385.230281736809957, 296.9336279125589613 ) ) ;
#106571=CARTESIAN_POINT ( 'NONE',  ( -8.848209551960000141, 1384.890560814510081, 199.9248350966889802 ) ) ;
#106585=AXIS2_PLACEMENT_3D ( 'NONE', #15285, #57881, #92550 ) ;
#106602=CARTESIAN_POINT ( 'NONE',  ( -25.61501306685740076, 1384.843999110390087, 224.1472815994760026 ) ) ;
#106603=CARTESIAN_POINT ( 'NONE',  ( -106.1058971500000041, 1378.913060387289988, 302.5343330838589395 ) ) ;
#106617=CARTESIAN_POINT ( 'NONE',  ( -13.69967938769999982, 1380.327631092480033, 209.8719513141080029 ) ) ;
#106623=CARTESIAN_POINT ( 'NONE',  ( -93.66127265309958716, 1377.138788487970032, 305.4911171557070020 ) ) ;
#106634=CARTESIAN_POINT ( 'NONE',  ( -103.9057015030000031, 1389.915727242629828, 305.4069455405589792 ) ) ;
#106643=ORIENTED_EDGE ( 'NONE', *, *, #87706, .F. ) ;
#106653=CARTESIAN_POINT ( 'NONE',  ( -12.31905933190130042, 1378.298490798669945, 209.5595369833839925 ) ) ;
#106658=CARTESIAN_POINT ( 'NONE',  ( -62.88186284109999491, 1374.821258372890043, 270.0876510056589836 ) ) ;
#106672=CARTESIAN_POINT ( 'NONE',  ( -13.38802240389999909, 1383.860181226410077, 218.7963554078490063 ) ) ;
#106676=CARTESIAN_POINT ( 'NONE',  ( -67.91765045250001265, 1379.745871413030045, 278.2920511910589880 ) ) ;
#106682=CARTESIAN_POINT ( 'NONE',  ( -106.5585968837300044, 1390.939245634569943, 300.3884029622149683 ) ) ;
#106684=CARTESIAN_POINT ( 'NONE',  ( -96.24057774249999397, 1384.839338083349958, 310.5876767322589558 ) ) ;
#106686=CARTESIAN_POINT ( 'NONE',  ( -20.43314471396830001, 1385.274570738710054, 221.1097988323519985 ) ) ;
#106702=CIRCLE ( 'NONE', #13729, 2.000048766321055993 ) ;
#106711=CARTESIAN_POINT ( 'NONE',  ( -107.9045857630000000, 1389.125896740649978, 298.5296598085590176 ) ) ;
#106743=CARTESIAN_POINT ( 'NONE',  ( -8.359385560594374098, 1382.870626080099782, 199.9003235427358334 ) ) ;
#106790=CARTESIAN_POINT ( 'NONE',  ( -16.59437507809930068, 1384.525787470290197, 200.9191608993760099 ) ) ;
#106816=CARTESIAN_POINT ( 'NONE',  ( -9.092793663155459782, 1384.840586518749888, 199.9433582416939998 ) ) ;
#106836=CARTESIAN_POINT ( 'NONE',  ( -107.1138176589999915, 1379.788324461719867, 299.4659512524589786 ) ) ;
#106839=CARTESIAN_POINT ( 'NONE',  ( -110.0632053599999978, 1385.194747628709820, 296.9590720091590015 ) ) ;
#106851=CARTESIAN_POINT ( 'NONE',  ( -43.05153967746429799, 1383.823344776070144, 247.3619861808770111 ) ) ;
#106861=CARTESIAN_POINT ( 'NONE',  ( -13.70246959700000033, 1380.890122814619872, 216.8472876221590013 ) ) ;
#106869=CARTESIAN_POINT ( 'NONE',  ( -8.546537168396879380, 1387.684766926490056, 218.1936297957030035 ) ) ;
#106881=CARTESIAN_POINT ( 'NONE',  ( -68.77339414690014507, 1379.748013015986317, 280.2450576337279813 ) ) ;
#106886=EDGE_CURVE ( 'NONE', #26163, #73589, #48074, .T. ) ;
#106889=B_SPLINE_CURVE_WITH_KNOTS ( 'NONE', 5,
 ( #6556, #107358, #6003, #73781, #15482, #22222, #101142, #39611, #7651, #66495, #100601, #58624, #92755, #56420, #90551 ),
 .UNSPECIFIED., .F., .F.,
 ( 6, 3, 3, 3, 6 ),
 ( 0.000000000000000000, 0.3703688121675461908, 0.5769812935202122128, 0.8426640375833164276, 1.000000000000000000 ),
 .UNSPECIFIED. ) ;
#106893=CARTESIAN_POINT ( 'NONE',  ( -109.4097255559999979, 1385.247472506640179, 311.2758024732589774 ) ) ;
#106904=CARTESIAN_POINT ( 'NONE',  ( -8.863675502250000449, 1385.133167759019898, 218.6777116865889923 ) ) ;
#106926=CARTESIAN_POINT ( 'NONE',  ( -6.355004503990000053, 1384.784618782699908, 199.7177247563389813 ) ) ;
#106961=CARTESIAN_POINT ( 'NONE',  ( -105.9134890463210041, 1391.838458166060036, 304.2044508906599845 ) ) ;
#106964=CIRCLE ( 'NONE', #58704, 7.842199003069996621 ) ;
#106970=CARTESIAN_POINT ( 'NONE',  ( -103.2673858233620052, 1384.938584610499902, 311.1084624176889974 ) ) ;
#106971=CARTESIAN_POINT ( 'NONE',  ( -8.372400094640001456, 1385.986562127730167, 199.8257561305989896 ) ) ;
#106984=CARTESIAN_POINT ( 'NONE',  ( -109.3697155611655489, 1387.313440419162134, 297.3840239876012674 ) ) ;
#107018=CARTESIAN_POINT ( 'NONE',  ( -93.24815347825941103, 1384.613258628189897, 309.6385292495870090 ) ) ;
#107020=CARTESIAN_POINT ( 'NONE',  ( -37.82349669198160313, 1384.984812771009729, 210.9237282750169982 ) ) ;
#107029=CARTESIAN_POINT ( 'NONE',  ( -109.3085299140000046, 1384.876463468619932, 311.2645433622590190 ) ) ;
#107040=CARTESIAN_POINT ( 'NONE',  ( -11.03395607409999890, 1380.324975612369826, 203.1430293853689761 ) ) ;
#107041=CARTESIAN_POINT ( 'NONE',  ( -13.08811655757008374, 1380.207677608032782, 214.5718171420391229 ) ) ;
#107053=CARTESIAN_POINT ( 'NONE',  ( -67.57970925394799622, 1379.745139398459969, 278.8730669361860350 ) ) ;
#107080=CARTESIAN_POINT ( 'NONE',  ( -14.53473250189999888, 1379.710786837239993, 208.2794111059409943 ) ) ;
#107081=CARTESIAN_POINT ( 'NONE',  ( -65.61919861378314067, 1379.740928103604574, 273.5950405564674952 ) ) ;
#107085=CARTESIAN_POINT ( 'NONE',  ( -54.32597545910780212, 1384.640566766860047, 232.6159698627500063 ) ) ;
#107086=ORIENTED_EDGE ( 'NONE', *, *, #12582, .F. ) ;
#107116=ORIENTED_EDGE ( 'NONE', *, *, #41222, .T. ) ;
#107143=CARTESIAN_POINT ( 'NONE',  ( -12.31949146158819985, 1378.253793448930082, 209.5105130821430066 ) ) ;
#107151=CARTESIAN_POINT ( 'NONE',  ( -28.43252842688429993, 1384.834145945409773, 226.5024172414440216 ) ) ;
#107178=CARTESIAN_POINT ( 'NONE',  ( -53.42892008310190022, 1379.491042053530009, 254.0488722920499640 ) ) ;
#107192=CARTESIAN_POINT ( 'NONE',  ( -104.2118261680000018, 1389.977870280240040, 305.3688602097590206 ) ) ;
#107210=CARTESIAN_POINT ( 'NONE',  ( -108.9869942201588913, 1387.752788737366473, 310.8052485749022367 ) ) ;
#107213=CARTESIAN_POINT ( 'NONE',  ( -12.60028346443769998, 1379.611581493590165, 209.5698690232689785 ) ) ;
#107217=CARTESIAN_POINT ( 'NONE',  ( -43.21650806019999891, 1376.046645985830082, 226.3493147691589797 ) ) ;
#107229=CARTESIAN_POINT ( 'NONE',  ( -54.13602515839999541, 1384.720040384200047, 270.3656545589590223 ) ) ;
#107233=CARTESIAN_POINT ( 'NONE',  ( -56.64534719470000113, 1379.747652096109960, 254.3393773118589536 ) ) ;
#107243=CARTESIAN_POINT ( 'NONE',  ( -31.71748227402730080, 1385.225470378949922, 229.9276196292890120 ) ) ;
#107249=CARTESIAN_POINT ( 'NONE',  ( -106.5186165409613466, 1391.553752504539716, 307.6918442614858122 ) ) ;
#107270=CARTESIAN_POINT ( 'NONE',  ( -105.7579672239999979, 1388.939243398469898, 299.5452684353589916 ) ) ;
#107272=CARTESIAN_POINT ( 'NONE',  ( -106.5656785119999910, 1391.248054752850067, 300.3923073593589947 ) ) ;
#107276=CARTESIAN_POINT ( 'NONE',  ( -105.3812639519999976, 1378.843495839950037, 304.0411346596590079 ) ) ;
#107278=CARTESIAN_POINT ( 'NONE',  ( -113.4000000000000057, 1379.886883438980021, 304.2218459572590064 ) ) ;
#107280=DIRECTION ( 'NONE',  ( -0.8090169943751894799, 3.009330011589934659E-31, -0.5877852522921398482 ) ) ;
#107289=CARTESIAN_POINT ( 'NONE',  ( -102.6163738449689902, 1383.762319109039936, 310.8816873798210167 ) ) ;
#107303=DIRECTION ( 'NONE',  ( -1.836970198721029688E-16, -1.000000000000000000, 0.000000000000000000 ) ) ;
#107308=CARTESIAN_POINT ( 'NONE',  ( -12.28946836655069852, 1378.262473314609906, 210.0681950494530099 ) ) ;
#107350=CARTESIAN_POINT ( 'NONE',  ( -25.73887467969239751, 1384.546265937980024, 203.5795097568579877 ) ) ;
#107357=CARTESIAN_POINT ( 'NONE',  ( -121.3986813195241723, 1384.899971913130003, 304.3468000529767323 ) ) ;
#107358=CARTESIAN_POINT ( 'NONE',  ( -14.05078142410000019, 1379.708754511839743, 206.9026084073089748 ) ) ;
#107377=CARTESIAN_POINT ( 'NONE',  ( -5.013264327984152224, 1375.413060387289988, 203.5257471471711312 ) ) ;
#107394=CARTESIAN_POINT ( 'NONE',  ( -109.1553531783490030, 1385.186054570089937, 297.1423525096689673 ) ) ;
#107409=CARTESIAN_POINT ( 'NONE',  ( -52.62061106118209608, 1383.807654112509908, 266.7032437734779933 ) ) ;
#107412=CARTESIAN_POINT ( 'NONE',  ( -9.094257307180781069, 1384.874748761890260, 199.9429999480310016 ) ) ;
#107417=CARTESIAN_POINT ( 'NONE',  ( -35.14840751239999861, 1380.299282000710036, 212.7497223807189926 ) ) ;
#107424=CARTESIAN_POINT ( 'NONE',  ( -11.34773204379960099, 1388.518463159120074, 216.6153406976970075 ) ) ;
#107443=AXIS2_PLACEMENT_3D ( 'NONE', #16885, #66261, #100378 ) ;
#107447=CARTESIAN_POINT ( 'NONE',  ( -108.9463587139999845, 1386.276479558989877, 311.0446671882590408 ) ) ;
#107457=CARTESIAN_POINT ( 'NONE',  ( -7.767268757120000089, 1385.037450386940009, 218.9155715650490208 ) ) ;
#107475=ORIENTED_EDGE ( 'NONE', *, *, #91070, .T. ) ;
#107476=CARTESIAN_POINT ( 'NONE',  ( -23.00263897809999847, 1384.817261601950122, 202.3843131321090141 ) ) ;
#107513=CARTESIAN_POINT ( 'NONE',  ( -106.0556850682889944, 1391.049837136749829, 307.0681549835799728 ) ) ;
#107520=CARTESIAN_POINT ( 'NONE',  ( -95.07483883942900604, 1384.957810138419973, 310.0626363712590319 ) ) ;
#107521=CARTESIAN_POINT ( 'NONE',  ( -9.930017291230001319, 1389.522641720639967, 201.7040244565289981 ) ) ;
#107536=CARTESIAN_POINT ( 'NONE',  ( -108.4312383940858382, 1388.726877007316716, 298.0798814299226365 ) ) ;
#107562=CARTESIAN_POINT ( 'NONE',  ( -104.4567500548372578, 1380.520305296903643, 307.5064808547090820 ) ) ;
#107568=CARTESIAN_POINT ( 'NONE',  ( -14.29022294670000015, 1380.323766294540064, 210.1136064056900068 ) ) ;
#107570=CARTESIAN_POINT ( 'NONE',  ( -58.47517137479839988, 1385.054044359190129, 240.7570610490290051 ) ) ;
#107578=ORIENTED_EDGE ( 'NONE', *, *, #43355, .T. ) ;
#107579=CARTESIAN_POINT ( 'NONE',  ( -109.9857366969999930, 1384.899971912069987, 311.4562997972589642 ) ) ;
#107582=CARTESIAN_POINT ( 'NONE',  ( -109.2989494770000078, 1384.622952429599763, 311.2534360572589662 ) ) ;
#107603=CARTESIAN_POINT ( 'NONE',  ( -67.63909761182219427, 1379.745505766160022, 278.9989825627670257 ) ) ;
#107618=CARTESIAN_POINT ( 'NONE',  ( -14.42577973733840047, 1379.717605820849940, 208.2725693216679872 ) ) ;
#107636=CARTESIAN_POINT ( 'NONE',  ( -63.57354255950622957, 1379.735521214616938, 269.2845494244093629 ) ) ;
#107641=CARTESIAN_POINT ( 'NONE',  ( -71.90316716507038564, 1384.749119938380090, 269.7490035479099788 ) ) ;
#107709=CARTESIAN_POINT ( 'NONE',  ( -24.59239876478699927, 1384.847462785510061, 223.4254781314130014 ) ) ;
#107713=CARTESIAN_POINT ( 'NONE',  ( -105.3194880639999980, 1379.015581655369942, 303.4536826814589858 ) ) ;
#107733=CARTESIAN_POINT ( 'NONE',  ( -11.16990621730810140, 1377.949346146600192, 211.9847173479319906 ) ) ;
#107735=CARTESIAN_POINT ( 'NONE',  ( -19.29089395862319734, 1379.713382923030167, 212.5251929917019993 ) ) ;
#107758=VERTEX_POINT ( 'NONE', #90333 ) ;
#107765=CARTESIAN_POINT ( 'NONE',  ( -12.33083890915290048, 1378.999358067989988, 209.7207202901829817 ) ) ;
#107769=CARTESIAN_POINT ( 'NONE',  ( -29.97486656939999961, 1379.299027991060029, 213.1946222551189862 ) ) ;
#107783=CARTESIAN_POINT ( 'NONE',  ( -96.27487712110000473, 1383.766385264410019, 310.4021576922589816 ) ) ;
#107788=CARTESIAN_POINT ( 'NONE',  ( -47.76848070539999469, 1379.673518999439921, 235.2760716095589828 ) ) ;
#107797=CARTESIAN_POINT ( 'NONE',  ( -96.24310955420000369, 1384.607824056739901, 310.5744048422590140 ) ) ;
#107798=CARTESIAN_POINT ( 'NONE',  ( -32.10879564089999860, 1385.224147136040074, 229.9470470709589733 ) ) ;
#107800=CARTESIAN_POINT ( 'NONE',  ( -47.10980919147239376, 1385.139645660309952, 255.7820939229709722 ) ) ;
#107825=CARTESIAN_POINT ( 'NONE',  ( -108.0060064069999868, 1388.416414365789933, 298.3043112637590184 ) ) ;
#107844=CARTESIAN_POINT ( 'NONE',  ( -103.7379217180000097, 1384.886069803950022, 296.9203887490589864 ) ) ;
#107872=CARTESIAN_POINT ( 'NONE',  ( 7.932410439648875489, 1391.426148861440197, 209.1218459572589836 ) ) ;
#107874=CARTESIAN_POINT ( 'NONE',  ( -8.379472588110001396, 1384.543820896499938, 199.7942522451990044 ) ) ;
#107896=CARTESIAN_POINT ( 'NONE',  ( -14.95647597185759992, 1384.522095472869751, 200.6334766323439851 ) ) ;
#107928=CARTESIAN_POINT ( 'NONE',  ( -9.123736379228210680, 1384.508619151900120, 199.9712811155520171 ) ) ;
#107944=EDGE_CURVE ( 'NONE', #110657, #109170, #102035, .T. ) ;
#107952=CARTESIAN_POINT ( 'NONE',  ( -121.3980906523484009, 1384.913060387289988, 304.3966198592502792 ) ) ;
#107962=CARTESIAN_POINT ( 'NONE',  ( -38.38927993948440331, 1383.830596176209838, 239.0580260840490041 ) ) ;
#107970=CARTESIAN_POINT ( 'NONE',  ( -8.870422689270000660, 1380.884123086199907, 216.4346137712589950 ) ) ;
#107976=CARTESIAN_POINT ( 'NONE',  ( -7.873989245522249547, 1386.913809585709942, 218.7666999748780086 ) ) ;
#107978=AXIS2_PLACEMENT_3D ( 'NONE', #38209, #12461, #29810 ) ;
#107980=CARTESIAN_POINT ( 'NONE',  ( -106.1530010540000006, 1379.143473661730013, 300.9588320359590057 ) ) ;
#107987=CARTESIAN_POINT ( 'NONE',  ( -67.87070494639999652, 1379.748617063760094, 278.3152404517590526 ) ) ;
#107997=CARTESIAN_POINT ( 'NONE',  ( -108.5006393170000081, 1386.602053732790182, 310.8681882702589974 ) ) ;
#108021=CARTESIAN_POINT ( 'NONE',  ( -107.6858065237089903, 1378.913060387379801, 300.3274025718760072 ) ) ;
#108027=CARTESIAN_POINT ( 'NONE',  ( -2.185878866602459838E-15, 1384.627966395730027, 199.6314228471690058 ) ) ;
#108044=EDGE_LOOP ( 'NONE', ( #85386, #72669, #78946, #84500, #100716, #57476 ) ) ;
#108053=CARTESIAN_POINT ( 'NONE',  ( -108.8100569807280351, 1381.628441269055884, 297.7725132315368910 ) ) ;
#108055=AXIS2_PLACEMENT_3D ( 'NONE', #16438, #76380, #93705 ) ;
#108058=CARTESIAN_POINT ( 'NONE',  ( -106.9652640938700046, 1391.913060387289988, 306.6581628094390339 ) ) ;
#108066=CARTESIAN_POINT ( 'NONE',  ( -94.96697414727451303, 1384.958059057069704, 310.0402463594970186 ) ) ;
#108068=CARTESIAN_POINT ( 'NONE',  ( -8.151272894939999958, 1385.300637405240195, 199.6428762611590173 ) ) ;
#108092=DIRECTION ( 'NONE',  ( 0.03618059822125301722, -0.9992709451211057026, -0.01218780329364530825 ) ) ;
#108098=CARTESIAN_POINT ( 'NONE',  ( -113.4000000000000057, 1384.913060387289988, 304.2218459572590064 ) ) ;
#108105=CARTESIAN_POINT ( 'NONE',  ( -103.6083266501182436, 1379.909801553448006, 304.7209094884234446 ) ) ;
#108109=CARTESIAN_POINT ( 'NONE',  ( -109.1309839890330124, 1384.924126711810004, 311.2646841801559958 ) ) ;
#108111=CARTESIAN_POINT ( 'NONE',  ( -12.29824070849999806, 1378.903937160740043, 210.1974271105389960 ) ) ;
#108113=CARTESIAN_POINT ( 'NONE',  ( -51.31128716130019995, 1385.023817170500024, 227.3449767567900039 ) ) ;
#108121=CARTESIAN_POINT ( 'NONE',  ( -109.8262407909999894, 1384.894770813300056, 311.3808759242589872 ) ) ;
#108140=AXIS2_PLACEMENT_3D ( 'NONE', #50794, #32874, #15509 ) ;
#108141=CARTESIAN_POINT ( 'NONE',  ( -5.065976868932539290, 1375.180419861180098, 203.5022389763250033 ) ) ;
#108149=CARTESIAN_POINT ( 'NONE',  ( -68.61976775002999318, 1379.747679567690057, 280.2166557527820032 ) ) ;
#108160=CARTESIAN_POINT ( 'NONE',  ( -107.1247494950929990, 1378.913060387289988, 307.3562546172859697 ) ) ;
#108175=CARTESIAN_POINT ( 'NONE',  ( -13.18452986259999982, 1379.569437749970120, 208.3223905408900123 ) ) ;
#108181=CARTESIAN_POINT ( 'NONE',  ( -82.48335923482800069, 1384.806338349549833, 286.1427824359119541 ) ) ;
#108220=CARTESIAN_POINT ( 'NONE',  ( -109.9019402774279968, 1384.041146777030008, 311.3911408799560263 ) ) ;
#108224=EDGE_CURVE ( 'NONE', #56949, #46666, #108450, .T. ) ;
#108227=CARTESIAN_POINT ( 'NONE',  ( -12.91238589569339901, 1379.507750453399922, 211.2365448389620042 ) ) ;
#108254=CARTESIAN_POINT ( 'NONE',  ( -50.54537835619269970, 1384.737437541280087, 262.8619960603269874 ) ) ;
#108255=CARTESIAN_POINT ( 'NONE',  ( -107.2521063185319861, 1391.913060387289988, 301.2044319119630131 ) ) ;
#108283=CARTESIAN_POINT ( 'NONE',  ( -11.23768197768379906, 1379.896853569739960, 211.2083033905840352 ) ) ;
#108314=CARTESIAN_POINT ( 'NONE',  ( -109.4770690486002422, 1386.916355746966929, 311.1337243306537061 ) ) ;
#108316=CARTESIAN_POINT ( 'NONE',  ( -12.31936382470650138, 1378.277364386369982, 209.5341328486059922 ) ) ;
#108321=CARTESIAN_POINT ( 'NONE',  ( -29.97486656949999784, 1376.157435337470133, 213.1946222555589827 ) ) ;
#108323=VERTEX_POINT ( 'NONE', #11092 ) ;
#108335=CARTESIAN_POINT ( 'NONE',  ( -47.38717424370000231, 1384.438055640320044, 256.2720914158589949 ) ) ;
#108351=CARTESIAN_POINT ( 'NONE',  ( -28.59007200240000302, 1388.502510938900059, 224.5857233694589752 ) ) ;
#108353=CARTESIAN_POINT ( 'NONE',  ( -50.29540186739819774, 1385.120236129709838, 262.3351411316949680 ) ) ;
#108363=CARTESIAN_POINT ( 'NONE',  ( -8.861845913810000752, 1384.884034691229999, 218.6850541249889943 ) ) ;
#108380=CARTESIAN_POINT ( 'NONE',  ( -106.9747615859999996, 1387.585777271070128, 298.0968282848589865 ) ) ;
#108383=CARTESIAN_POINT ( 'NONE',  ( -106.1541768740000009, 1391.913060387289988, 303.5024934578589750 ) ) ;
#108404=VERTEX_POINT ( 'NONE', #40131 ) ;
#108432=CARTESIAN_POINT ( 'NONE',  ( -8.154251837229999467, 1384.787012670900140, 199.6488997829790151 ) ) ;
#108446=EDGE_CURVE ( 'NONE', #19741, #74400, #5508, .T. ) ;
#108450=B_SPLINE_CURVE_WITH_KNOTS ( 'NONE', 5,
 ( #59296, #43034, #92861, #44141, #1046, #41922, #68257, #86127, #58726, #34618, #50877, #16138, #68803, #76078, #102905 ),
 .UNSPECIFIED., .F., .F.,
 ( 6, 3, 3, 3, 6 ),
 ( 0.000000000000000000, 0.1365561072326384739, 0.2978444876294450983, 0.5106123751859845683, 1.000000000000000000 ),
 .UNSPECIFIED. ) ;
#108461=ORIENTED_EDGE ( 'NONE', *, *, #96150, .T. ) ;
#108469=CARTESIAN_POINT ( 'NONE',  ( -68.77345375519999493, 1379.748012843780089, 280.2452975165590487 ) ) ;
#108519=CARTESIAN_POINT ( 'NONE',  ( -50.70725589956350632, 1383.810751608489909, 262.7987874578989818 ) ) ;
#108528=CARTESIAN_POINT ( 'NONE',  ( -45.95279786519999732, 1383.059815259339985, 219.1337940620589961 ) ) ;
#108531=ORIENTED_EDGE ( 'NONE', *, *, #104202, .T. ) ;
#108533=CARTESIAN_POINT ( 'NONE',  ( -7.984562924460901101, 1386.832004956829905, 218.6792132728400020 ) ) ;
#108538=CARTESIAN_POINT ( 'NONE',  ( -105.2984536779999871, 1379.565129866090047, 301.9749307548589741 ) ) ;
#108549=DIRECTION ( 'NONE',  ( 0.9702683578407125253, 0.000000000000000000, -0.2420316379589395328 ) ) ;
#108557=CARTESIAN_POINT ( 'NONE',  ( -108.9096775629999883, 1387.161515960729957, 310.8237188872590195 ) ) ;
#108590=CARTESIAN_POINT ( 'NONE',  ( -58.29236204880000116, 1384.661700128139955, 240.0739325125589971 ) ) ;
#108604=CARTESIAN_POINT ( 'NONE',  ( -8.861482052969998691, 1384.950957082100103, 218.6848127019790127 ) ) ;
#108605=CYLINDRICAL_SURFACE ( 'NONE', #61662, 2.500000000000001776 ) ;
#108619=CIRCLE ( 'NONE', #37176, 7.868384924639995504 ) ;
#108621=CARTESIAN_POINT ( 'NONE',  ( -13.08811969939999997, 1380.207675299450102, 214.5718119823889936 ) ) ;
#108626=CIRCLE ( 'NONE', #38839, 2.000079913604663417 ) ;
#108627=CARTESIAN_POINT ( 'NONE',  ( -103.9199421708199935, 1384.937015199220014, 311.1477413758909734 ) ) ;
#108628=CARTESIAN_POINT ( 'NONE',  ( -7.954531997339999272, 1385.329339385649973, 199.4936033243889710 ) ) ;
#108644=CARTESIAN_POINT ( 'NONE',  ( 8.432239102140002274, 1391.913060387289988, 209.1218459572589836 ) ) ;
#108663=CARTESIAN_POINT ( 'NONE',  ( -5.432410439472700858, 1391.426148861440197, 203.3415300314919989 ) ) ;
#108665=CARTESIAN_POINT ( 'NONE',  ( -105.2424085362494139, 1381.071453570725225, 308.6724721103511229 ) ) ;
#108669=CARTESIAN_POINT ( 'NONE',  ( -109.1311308840000009, 1384.934002237980167, 311.2646438852589768 ) ) ;
#108671=CARTESIAN_POINT ( 'NONE',  ( -12.30621109530000012, 1378.371660281350159, 209.8675522742090038 ) ) ;
#108673=CARTESIAN_POINT ( 'NONE',  ( -66.81779111251940151, 1385.096065578679827, 259.0793199826619571 ) ) ;
#108685=CARTESIAN_POINT ( 'NONE',  ( -109.4663766940000045, 1384.534820742290094, 311.2654509672589711 ) ) ;
#108703=CARTESIAN_POINT ( 'NONE',  ( -68.46221940491409441, 1379.747295280180197, 280.0472515979760146 ) ) ;
#108706=CARTESIAN_POINT ( 'NONE',  ( -9.029782795278201490, 1380.828793225110530, 217.6116281277577684 ) ) ;
#108715=CARTESIAN_POINT ( 'NONE',  ( -108.0661742336610018, 1378.913060387289988, 308.5496305239910271 ) ) ;
#108722=ORIENTED_EDGE ( 'NONE', *, *, #90209, .F. ) ;
#108733=CARTESIAN_POINT ( 'NONE',  ( -5.013435694540000043, 1375.426148861440197, 203.5256706139790310 ) ) ;
#108734=CARTESIAN_POINT ( 'NONE',  ( -13.86144133729999872, 1379.734592797399955, 208.2043628488259799 ) ) ;
#108738=FACE_OUTER_BOUND ( 'NONE', #92170, .T. ) ;
#108739=CARTESIAN_POINT ( 'NONE',  ( -83.31223204895070467, 1384.810193783940122, 287.0493513657310132 ) ) ;
#108774=CARTESIAN_POINT ( 'NONE',  ( -109.9698195215979979, 1384.452562162210143, 311.4357956501490321 ) ) ;
#108788=AXIS2_PLACEMENT_3D ( 'NONE', #108098, #91852, #48777 ) ;
#108789=CYLINDRICAL_SURFACE ( 'NONE', #40710, 0.5000000000000031086 ) ;
#108792=CARTESIAN_POINT ( 'NONE',  ( -8.723519235820038631, 1388.537837264801283, 217.9447364732859853 ) ) ;
#108809=CARTESIAN_POINT ( 'NONE',  ( -51.28913027418060011, 1384.733897297830026, 264.3868833375080385 ) ) ;
#108810=CARTESIAN_POINT ( 'NONE',  ( -107.3690818753550076, 1391.913060387289988, 300.9869897165519887 ) ) ;
#108824=CARTESIAN_POINT ( 'NONE',  ( -12.45150583203999872, 1379.026621145309946, 211.0139914652599771 ) ) ;
#108833=CARTESIAN_POINT ( 'NONE',  ( -11.40323313910470127, 1380.342188320790001, 209.3118107140630002 ) ) ;
#108835=CARTESIAN_POINT ( 'NONE',  ( -54.27049659481630073, 1379.703136558600136, 254.1616898847049981 ) ) ;
#108864=CARTESIAN_POINT ( 'NONE',  ( -109.4829888131453259, 1386.904664127187289, 311.1374333086192223 ) ) ;
#108866=CARTESIAN_POINT ( 'NONE',  ( -13.12422835985349856, 1380.070863199510086, 209.3681815004020166 ) ) ;
#108872=CARTESIAN_POINT ( 'NONE',  ( -29.19545364349999872, 1380.228231664269970, 214.3784411298690031 ) ) ;
#108885=CARTESIAN_POINT ( 'NONE',  ( -36.11164246829999769, 1384.804902789069956, 235.4725595070590032 ) ) ;
#108901=CARTESIAN_POINT ( 'NONE',  ( -50.81938515019999869, 1390.824046508720130, 243.7260639249589929 ) ) ;
#108903=CARTESIAN_POINT ( 'NONE',  ( -49.76867394811179679, 1385.123425707419756, 261.2502804024239822 ) ) ;
#108914=CARTESIAN_POINT ( 'NONE',  ( -8.297441882400001134, 1384.888147545379979, 218.7035559121489996 ) ) ;
#108934=CARTESIAN_POINT ( 'NONE',  ( -104.8482432769999946, 1389.575902442549932, 300.8837059871590327 ) ) ;
#108980=EDGE_LOOP ( 'NONE', ( #104748, #9869, #37768, #3711, #72657 ) ) ;
#108991=CARTESIAN_POINT ( 'NONE',  ( -8.845811798939999804, 1384.799939604860128, 199.9263747969989709 ) ) ;
#109010=B_SPLINE_SURFACE_WITH_KNOTS ( 'NONE', 5, 5, ( 
 ( #88854, #4308, #12138, #80460, #79911, #79358 ),
 ( #21619, #12692, #13219, #105105, #2672, #45776 ),
 ( #70989, #3224, #3773, #28396, #36797, #73157 ),
 ( #37906, #106202, #62596, #63680, #87768, #98346 ),
 ( #11049, #81531, #38980, #72611, #63143, #37351 ),
 ( #28954, #55274, #55824, #97244, #96713, #97791 ) ),
 .UNSPECIFIED., .F., .F., .F.,
 ( 6, 6 ),
 ( 6, 6 ),
 ( 0.9031050603770000018, 1.041569279630000011 ),
 ( 0.000000000000000000, 2.000000000000000000 ),
 .UNSPECIFIED. ) ;
#109018=CARTESIAN_POINT ( 'NONE',  ( -41.60088707320420554, 1384.587835658240010, 214.5004774267979997 ) ) ;
#109034=CARTESIAN_POINT ( 'NONE',  ( -68.77631069450001178, 1379.747998137240074, 280.2624785784589676 ) ) ;
#109051=CARTESIAN_POINT ( 'NONE',  ( -10.22326110114815201, 1374.913060387290216, 213.8507217284212345 ) ) ;
#109077=DIRECTION ( 'NONE',  ( -0.02617070069600989368, -0.9996573249755577040, 0.0005718809247485686070 ) ) ;
#109089=CARTESIAN_POINT ( 'NONE',  ( -37.20393503414990022, 1383.832344231630032, 237.1622210560479971 ) ) ;
#109098=B_SPLINE_SURFACE_WITH_KNOTS ( 'NONE', 5, 5, ( 
 ( #92180, #7074, #83779, #110082, #66460, #41230 ),
 ( #75929, #92722, #13796, #57503, #5973, #101109 ),
 ( #67552, #108432, #83230, #74847, #108991, #47981 ),
 ( #22738, #32813, #5420, #39579, #73751, #56942 ),
 ( #50200, #24406, #65352, #82683, #91071, #31162 ),
 ( #58591, #15998, #107874, #84326, #99460, #7616 ),
 ( #41773, #101654, #14354, #40118, #24942, #110632 ),
 ( #85410, #353, #43993, #17084, #68654, #69202 ),
 ( #94939, #44546, #8159, #43442, #102755, #51278 ) ),
 .UNSPECIFIED., .F., .F., .F.,
 ( 6, 3, 6 ),
 ( 6, 6 ),
 ( 4.382742598350000129, 4.857690652960000577, 5.332638707570000136 ),
 ( 0.000000000000000000, 2.000000000000000000 ),
 .UNSPECIFIED. ) ;
#109099=CARTESIAN_POINT ( 'NONE',  ( -55.92238506969999889, 1380.972976875320001, 269.5160511658589826 ) ) ;
#109103=CARTESIAN_POINT ( 'NONE',  ( -8.801669235211798892, 1386.375422881679924, 218.4188921187869994 ) ) ;
#109109=CARTESIAN_POINT ( 'NONE',  ( -105.5449098450000065, 1380.452663771340212, 300.3143822648590344 ) ) ;
#109115=CARTESIAN_POINT ( 'NONE',  ( -108.4578349762840048, 1385.240951097619927, 297.1233463436130364 ) ) ;
#109128=CARTESIAN_POINT ( 'NONE',  ( -109.7404430409999918, 1384.933520221859908, 311.3564660812589864 ) ) ;
#109141=ORIENTED_EDGE ( 'NONE', *, *, #7673, .T. ) ;
#109158=CARTESIAN_POINT ( 'NONE',  ( -62.46146343959999570, 1384.944962066419976, 249.2984044847590042 ) ) ;
#109170=VERTEX_POINT ( 'NONE', #34774 ) ;
#109190=CARTESIAN_POINT ( 'NONE',  ( -12.82201593589999966, 1380.181586896640056, 214.4577599001689805 ) ) ;
#109198=CARTESIAN_POINT ( 'NONE',  ( -9.439187927669999922, 1387.430105989039930, 200.7363142262489930 ) ) ;
#109203=CARTESIAN_POINT ( 'NONE',  ( -9.046479669355809605, 1384.024798239620168, 218.5728259558869979 ) ) ;
#109209=CARTESIAN_POINT ( 'NONE',  ( -109.4150851273395091, 1387.231176170051413, 297.3550453227194339 ) ) ;
#109215=ADVANCED_FACE ( 'NONE', ( #47590 ), #103567, .F. ) ;
#109231=CARTESIAN_POINT ( 'NONE',  ( -110.0631564100000048, 1384.903609496989930, 296.9512625404590267 ) ) ;
#109235=CARTESIAN_POINT ( 'NONE',  ( -108.6616353267809956, 1383.758284946439971, 311.0749865448200353 ) ) ;
#109240=CARTESIAN_POINT ( 'NONE',  ( -13.07882001760000179, 1380.090973434839952, 209.8378495415080067 ) ) ;
#109242=CARTESIAN_POINT ( 'NONE',  ( -55.50096278363709956, 1385.040616669380142, 234.7978539123299981 ) ) ;
#109243=CARTESIAN_POINT ( 'NONE',  ( -10.98637326466459996, 1391.913060387289988, 212.5523432083540172 ) ) ;
#109254=CARTESIAN_POINT ( 'NONE',  ( -109.4849127990000142, 1384.882923849199869, 311.2840631412590255 ) ) ;
#109257=CARTESIAN_POINT ( 'NONE',  ( -113.4825880485180960, 1391.913060387289988, 307.7208714236175524 ) ) ;
#109260=CARTESIAN_POINT ( 'NONE',  ( -14.01398736212220086, 1379.590348564800024, 211.9184487047760115 ) ) ;
#109270=CARTESIAN_POINT ( 'NONE',  ( -68.61722315264249517, 1379.747600866859784, 280.2192988058840228 ) ) ;
#109299=CARTESIAN_POINT ( 'NONE',  ( -12.33566090380000091, 1378.557429905330082, 208.8728726537019895 ) ) ;
#109303=CARTESIAN_POINT ( 'NONE',  ( -10.82294938829999964, 1391.816256682959875, 214.1756021292690093 ) ) ;
#109304=CARTESIAN_POINT ( 'NONE',  ( -81.68753388954969807, 1384.802559585820063, 285.2219065580749771 ) ) ;
#109354=COLOUR_RGB ( '', 0.66274510, 0.83137255, 0.94901961) ;
#109358=CARTESIAN_POINT ( 'NONE',  ( -9.835648583419363433, 1390.019383093769193, 216.6175827202515336 ) ) ;
#109377=CARTESIAN_POINT ( 'NONE',  ( -43.14089593232999675, 1384.773049472099956, 247.9047009284290084 ) ) ;
#109384=CARTESIAN_POINT ( 'NONE',  ( -10.94870340160153965, 1379.126484780772671, 203.4065785939058060 ) ) ;
#109404=CARTESIAN_POINT ( 'NONE',  ( -18.16996689059999781, 1377.005697473339978, 212.7263676204689773 ) ) ;
#109406=CARTESIAN_POINT ( 'NONE',  ( -40.54664627463470339, 1379.659233182239859, 229.3558487376700157 ) ) ;
#109407=ORIENTED_EDGE ( 'NONE', *, *, #81894, .F. ) ;
#109431=CARTESIAN_POINT ( 'NONE',  ( -107.7563153173368704, 1389.383687039567803, 309.7269953625564085 ) ) ;
#109437=CARTESIAN_POINT ( 'NONE',  ( -19.16011841990000164, 1375.603804398499960, 208.8610751811249884 ) ) ;
#109449=CARTESIAN_POINT ( 'NONE',  ( -59.23371022229999738, 1384.698177673139980, 279.9261678725590059 ) ) ;
#109462=CARTESIAN_POINT ( 'NONE',  ( -65.92084310709999784, 1389.515675200419764, 264.7571888138589316 ) ) ;
#109464=CARTESIAN_POINT ( 'NONE',  ( -44.14048389105859371, 1385.157692499700033, 249.8217694268669788 ) ) ;
#109473=CARTESIAN_POINT ( 'NONE',  ( -8.297292677819999795, 1384.885217424269740, 218.7035352472190084 ) ) ;
#109475=CARTESIAN_POINT ( 'NONE',  ( 11.13055623967079377, 1375.886883438980021, 203.9732913815154234 ) ) ;
#109486=CARTESIAN_POINT ( 'NONE',  ( -106.1567580175403265, 1391.062840735999316, 301.1121656807407021 ) ) ;
#109519=CARTESIAN_POINT ( 'NONE',  ( -12.30515845580959855, 1378.366303543320100, 209.8813026182200190 ) ) ;
#109559=CARTESIAN_POINT ( 'NONE',  ( -101.9775983549999978, 1378.556086106449811, 301.8221755499590699 ) ) ;
#109565=CARTESIAN_POINT ( 'NONE',  ( -38.17413872016189913, 1384.577420189890063, 211.2523201417219809 ) ) ;
#109577=CARTESIAN_POINT ( 'NONE',  ( -68.78035664479999411, 1379.747944962379961, 280.2443459286590155 ) ) ;
#109607=CARTESIAN_POINT ( 'NONE',  ( -7.545120860308170307, 1384.909328162950032, 219.0876147414010120 ) ) ;
#109617=EDGE_LOOP ( 'NONE', ( #91893, #8048, #80657, #1749 ) ) ;
#109629=CARTESIAN_POINT ( 'NONE',  ( -54.59994543616350171, 1383.804537930590186, 270.6530719560610123 ) ) ;
#109637=CARTESIAN_POINT ( 'NONE',  ( -39.62519685099999833, 1379.010909650270150, 224.0738340640590138 ) ) ;
#109646=CARTESIAN_POINT ( 'NONE',  ( -107.9473430369999960, 1380.764990262600122, 298.5035467044589836 ) ) ;
#109662=ADVANCED_FACE ( 'NONE', ( #13982 ), #25148, .T. ) ;
#109667=CARTESIAN_POINT ( 'NONE',  ( -105.3787933579999958, 1390.956730496739965, 305.3341016426589931 ) ) ;
#109692=CARTESIAN_POINT ( 'NONE',  ( -7.989567385690000023, 1384.306347471770096, 199.5291465469090042 ) ) ;
#109696=CARTESIAN_POINT ( 'NONE',  ( -84.12715333319998479, 1385.173288781940073, 288.0594686105589517 ) ) ;
#109699=CARTESIAN_POINT ( 'NONE',  ( -109.9852174251870025, 1384.905086218720044, 311.4561813548020268 ) ) ;
#109713=ORIENTED_EDGE ( 'NONE', *, *, #24086, .T. ) ;
#109726=CARTESIAN_POINT ( 'NONE',  ( -11.00250985070000098, 1379.595586062069970, 215.1074884732990142 ) ) ;
#109730=CARTESIAN_POINT ( 'NONE',  ( -5.513264357029999729, 1374.913060387289988, 214.9370262455390161 ) ) ;
#109737=CARTESIAN_POINT ( 'NONE',  ( -8.960270527080961500, 1384.233187754379969, 218.6195202797470074 ) ) ;
#109756=CARTESIAN_POINT ( 'NONE',  ( -109.2297890131749938, 1384.978503039539873, 295.1339919130639942 ) ) ;
#109767=CARTESIAN_POINT ( 'NONE',  ( -109.8948235710000034, 1384.907847270719913, 297.0284604404590141 ) ) ;
#109781=B_SPLINE_SURFACE_WITH_KNOTS ( 'NONE', 5, 5, ( 
 ( #101354, #49345, #100288, #109254, #57762, #99714 ),
 ( #99160, #49897, #84029, #40927, #82929, #75106 ),
 ( #31419, #22440, #73995, #5119, #48806, #15154 ),
 ( #23568, #32537, #83471, #39275, #56642, #47689 ),
 ( #14059, #73449, #6221, #109792, #90776, #75653 ),
 ( #7330, #48246, #6765, #91334, #23007, #31977 ),
 ( #41493, #66709, #81817, #40373, #107582, #100817 ),
 ( #24104, #14619, #33071, #74552, #58296, #67262 ),
 ( #82389, #30868, #65601, #108685, #66167, #65045 ) ),
 .UNSPECIFIED., .F., .F., .F.,
 ( 6, 3, 6 ),
 ( 6, 6 ),
 ( 3.112795738710000037, 3.535848030919999996, 3.958900323119999953 ),
 ( 0.000000000000000000, 2.000000000000000000 ),
 .UNSPECIFIED. ) ;
#109782=CARTESIAN_POINT ( 'NONE',  ( -51.62800087644459524, 1385.024991398460088, 227.8640657499650217 ) ) ;
#109783=CARTESIAN_POINT ( 'NONE',  ( -10.57737777167070092, 1391.913060387289988, 213.4296204213179919 ) ) ;
#109792=CARTESIAN_POINT ( 'NONE',  ( -109.4849921600000044, 1384.708507898549897, 311.2789825532589703 ) ) ;
#109808=CARTESIAN_POINT ( 'NONE',  ( -109.1340195298539868, 1384.837378371770001, 311.2641337568139761 ) ) ;
#109810=CARTESIAN_POINT ( 'NONE',  ( -68.63115668882700504, 1379.747695794610081, 280.2278140600810161 ) ) ;
#109813=CARTESIAN_POINT ( 'NONE',  ( -8.155564057308037462, 1382.295710237911635, 218.5042669288760351 ) ) ;
#109846=CARTESIAN_POINT ( 'NONE',  ( -10.57531603410000010, 1391.913060387289988, 213.4590788534990224 ) ) ;
#109847=CARTESIAN_POINT ( 'NONE',  ( -70.69354556520289634, 1384.741626837030026, 267.3362997785129664 ) ) ;
#109863=CARTESIAN_POINT ( 'NONE',  ( -63.97154863419999771, 1379.735362472459883, 270.2946752427589558 ) ) ;
#109877=CARTESIAN_POINT ( 'NONE',  ( -9.095131050099999115, 1384.919789133580025, 199.9427535748389744 ) ) ;
#109895=CARTESIAN_POINT ( 'NONE',  ( -8.203619622988481908, 1387.619530229529573, 218.4591758698915385 ) ) ;
#109914=CARTESIAN_POINT ( 'NONE',  ( -48.31785227133409677, 1384.748160175390012, 258.2760858809979823 ) ) ;
#109915=CARTESIAN_POINT ( 'NONE',  ( -107.4307047400000101, 1391.913060387289988, 300.8770155100590387 ) ) ;
#109919=CARTESIAN_POINT ( 'NONE',  ( -107.2490594869999967, 1379.226189117420063, 299.5843691631590104 ) ) ;
#109923=CARTESIAN_POINT ( 'NONE',  ( -9.715864373837542090, 1380.601324416629950, 201.4379534463959089 ) ) ;
#109934=DIRECTION ( 'NONE',  ( -1.000000000000000000, 0.000000000000000000, 0.000000000000000000 ) ) ;
#109945=CARTESIAN_POINT ( 'NONE',  ( -40.62420891447809623, 1380.117468965909893, 228.1401504654660073 ) ) ;
#109947=CARTESIAN_POINT ( 'NONE',  ( -43.37329540369329806, 1379.677816877510168, 233.3348431341099740 ) ) ;
#109948=EDGE_LOOP ( 'NONE', ( #106643, #77036, #88095, #68216 ) ) ;
#109953=CARTESIAN_POINT ( 'NONE',  ( -106.4659219139999919, 1378.913060387289988, 306.4416122446589839 ) ) ;
#109963=( NAMED_UNIT ( * ) PLANE_ANGLE_UNIT ( ) SI_UNIT ( $, .RADIAN. ) );
#109969=ORIENTED_EDGE ( 'NONE', *, *, #30123, .F. ) ;
#109981=CARTESIAN_POINT ( 'NONE',  ( -25.65041448810000091, 1375.250345454859826, 213.2122020707489867 ) ) ;
#109986=CARTESIAN_POINT ( 'NONE',  ( -104.1899534433839989, 1379.825714327339938, 304.5166623431679795 ) ) ;
#109995=DIRECTION ( 'NONE',  ( 1.000000000000000000, 0.000000000000000000, 0.000000000000000000 ) ) ;
#110005=CARTESIAN_POINT ( 'NONE',  ( -64.63783698019999235, 1389.443172118360053, 283.2195019318589857 ) ) ;
#110007=CARTESIAN_POINT ( 'NONE',  ( -52.46234346565999829, 1385.107285400780029, 266.7644260104040086 ) ) ;
#110016=CARTESIAN_POINT ( 'NONE',  ( -8.023236064449998040, 1384.902848846080133, 218.7875339973990094 ) ) ;
#110018=CARTESIAN_POINT ( 'NONE',  ( -108.2726263712360009, 1382.330192459420005, 310.4990597502870173 ) ) ;
#110024=DIRECTION ( 'NONE',  ( -0.8090169943751635007, 0.000000000000000000, -0.5877852522921759304 ) ) ;
#110031=CARTESIAN_POINT ( 'NONE',  ( -109.1662451990000022, 1385.640949607019820, 297.1854764981590051 ) ) ;
#110035=( BOUNDED_CURVE ( )  B_SPLINE_CURVE ( 3, ( #58310, #24659, #30884, #99732 ),
 .UNSPECIFIED., .F., .F. ) 
 B_SPLINE_CURVE_WITH_KNOTS ( ( 4, 4 ),
 ( 0.003816089188682000085, 0.02499446558039379943 ),
 .UNSPECIFIED. ) 
 CURVE ( )  GEOMETRIC_REPRESENTATION_ITEM ( )  RATIONAL_B_SPLINE_CURVE ( ( 1.000000000000000000, 0.9999626233803757813, 0.9999626233803757813, 1.000000000000000000 ) ) 
 REPRESENTATION_ITEM ( '' )  );
#110045=B_SPLINE_SURFACE_WITH_KNOTS ( 'NONE', 5, 5, ( 
 ( #67487, #25984, #51215, #34412, #85346, #42263, #1372, #68584, #103826 ),
 ( #9758, #43379, #86465, #18693, #76411, #102689, #8642, #94872, #102152 ),
 ( #43922, #93738, #9221, #110565, #35514, #18149, #77528, #42818, #60749 ),
 ( #59084, #60184, #52890, #87018, #110018, #52344, #10310, #33294, #50665 ),
 ( #34957, #17016, #69707, #94301, #103245, #25431, #69141, #17578, #51779 ),
 ( #68042, #59627, #85917, #16474, #27126, #84797, #75868, #101590, #24876 ),
 ( #93204, #45605, #29319, #80287, #3603, #104934, #46157, #88146, #62408 ),
 ( #97091, #70267, #62979, #97635, #11434, #36624, #44483, #37180, #27672 ),
 ( #20904, #71376, #36082, #79747, #96536, #3054, #19810, #53447, #63519 ),
 ( #55105, #89229, #71930, #20356, #37726, #12525, #87593, #105488, #54016 ),
 ( #2503, #11976, #106042, #28221, #28779, #10881, #46703, #80833, #54561 ),
 ( #78629, #1944, #88695, #104376, #61857, #95977, #19238, #45053, #79197 ),
 ( #70822, #60715, #794, #85880, #42782, #43346, #27094, #69672, #103794 ),
 ( #16983, #51182, #94267, #75836, #34379, #93168, #109986, #94836, #33263 ),
 ( #42232, #84219, #50632, #77494, #78032, #102652, #41677, #76941, #34923 ) ),
 .UNSPECIFIED., .F., .F., .F.,
 ( 6, 3, 3, 3, 6 ),
 ( 6, 3, 6 ),
 ( 7.295781771626849377, 12.20883758960000165, 16.12185770279999986, 21.25293827189999973, 26.14845333426159968 ),
 ( 0.000000000000000000, 1.000000000000000000, 2.002578320861649885 ),
 .UNSPECIFIED. ) ;
#110064=CARTESIAN_POINT ( 'NONE',  ( -12.31034457511139912, 1378.376182853990031, 209.7966525762110166 ) ) ;
#110082=CARTESIAN_POINT ( 'NONE',  ( -8.604091700990000646, 1384.887133332230178, 199.8687248843490067 ) ) ;
#110085=CARTESIAN_POINT ( 'NONE',  ( 0.000000000000000000, 0.000000000000000000, 0.000000000000000000 ) ) ;
#110092=CARTESIAN_POINT ( 'NONE',  ( -12.56636063060000019, 1391.397300678690044, 209.2272092290610033 ) ) ;
#110107=CARTESIAN_POINT ( 'NONE',  ( -44.53110276769830023, 1384.597785574959971, 217.7731154659030040 ) ) ;
#110108=CIRCLE ( 'NONE', #88454, 0.9999999999999956701 ) ;
#110120=CARTESIAN_POINT ( 'NONE',  ( -68.13004150250000635, 1379.747519519559773, 278.8017379516589926 ) ) ;
#110150=CARTESIAN_POINT ( 'NONE',  ( -103.5806803890000083, 1389.940350142260058, 304.1776731731589507 ) ) ;
#110163=VERTEX_POINT ( 'NONE', #6915 ) ;
#110173=CARTESIAN_POINT ( 'NONE',  ( -62.79534954047180406, 1383.793091064959981, 285.1732082431380491 ) ) ;
#110180=CARTESIAN_POINT ( 'NONE',  ( -64.43287619839999536, 1383.188014472239956, 254.0808989357590235 ) ) ;
#110183=ORIENTED_EDGE ( 'NONE', *, *, #4553, .T. ) ;
#110185=CARTESIAN_POINT ( 'NONE',  ( -7.973011292860630483, 1385.871086923890061, 218.7772657474099844 ) ) ;
#110189=CARTESIAN_POINT ( 'NONE',  ( -106.6038969349999945, 1381.976044154610008, 298.3535665123590093 ) ) ;
#110211=CARTESIAN_POINT ( 'NONE',  ( -107.5382083149999914, 1388.218888600149967, 309.8897308892589990 ) ) ;
#110222=ORIENTED_EDGE ( 'NONE', *, *, #18438, .F. ) ;
#110258=CARTESIAN_POINT ( 'NONE',  ( -9.656246557070002012, 1389.622605478320111, 203.2012388434289960 ) ) ;
#110267=CARTESIAN_POINT ( 'NONE',  ( -13.01267508979999832, 1379.476792316909950, 212.2796297140689887 ) ) ;
#110274=CARTESIAN_POINT ( 'NONE',  ( -12.85016526419999927, 1389.184315283510159, 203.6059765727289914 ) ) ;
#110282=CARTESIAN_POINT ( 'NONE',  ( -8.868004540950760628, 1384.633249023989947, 218.6740787338979999 ) ) ;
#110315=EDGE_CURVE ( 'NONE', #34413, #55324, #52123, .T. ) ;
#110321=CARTESIAN_POINT ( 'NONE',  ( -108.4550367074038633, 1381.313848681411628, 310.3901933583101140 ) ) ;
#110325=CARTESIAN_POINT ( 'NONE',  ( -11.06863488910000015, 1391.913060387289988, 206.1140686093889940 ) ) ;
#110326=CARTESIAN_POINT ( 'NONE',  ( -83.57052189370659789, 1385.171097491720047, 287.3315033242400318 ) ) ;
#110327=CARTESIAN_POINT ( 'NONE',  ( -10.95274535029249918, 1391.913060387289988, 212.6322721876839807 ) ) ;
#110351=CARTESIAN_POINT ( 'NONE',  ( -68.62231159920000323, 1379.747791814530046, 280.2140134006589847 ) ) ;
#110352=ORIENTED_EDGE ( 'NONE', *, *, #76182, .F. ) ;
#110354=CARTESIAN_POINT ( 'NONE',  ( -10.78658054680221134, 1378.764302627705092, 215.1167326068625414 ) ) ;
#110386=DIRECTION ( 'NONE',  ( -1.000000000000000000, 0.000000000000000000, 0.000000000000000000 ) ) ;
#110387=CARTESIAN_POINT ( 'NONE',  ( -9.809994181400000457, 1391.913060387289988, 214.8154632703889888 ) ) ;
#110388=CARTESIAN_POINT ( 'NONE',  ( -93.79108000015780533, 1384.853053930580018, 294.4783922775349652 ) ) ;
#110406=CARTESIAN_POINT ( 'NONE',  ( -54.48829305249999777, 1379.705335535419863, 248.9076988030590201 ) ) ;
#110411=AXIS2_PLACEMENT_3D ( 'NONE', #87734, #96676, #19949 ) ;
#110422=CARTESIAN_POINT ( 'NONE',  ( -7.966081158779999782, 1384.918389535180040, 199.4892681704289998 ) ) ;
#110434=CIRCLE ( 'NONE', #10286, 7.868384924639995504 ) ;
#110457=CARTESIAN_POINT ( 'NONE',  ( -12.17955882736053930, 1377.723645317214277, 210.9225509704534716 ) ) ;
#110463=CARTESIAN_POINT ( 'NONE',  ( -49.22008464409690021, 1384.743802012480046, 260.1336803388579710 ) ) ;
#110471=CARTESIAN_POINT ( 'NONE',  ( -8.465783460212520595, 1382.621316526051260, 200.0067512675162504 ) ) ;
#110479=CARTESIAN_POINT ( 'NONE',  ( 1.756561144747210293E-16, 1391.913060387289988, 209.1218459572589836 ) ) ;
#110493=CARTESIAN_POINT ( 'NONE',  ( -29.69371359589970183, 1379.627920369189951, 218.1711912100410018 ) ) ;
#110498=VERTEX_POINT ( 'NONE', #65353 ) ;
#110499=CARTESIAN_POINT ( 'NONE',  ( -106.2815828819999950, 1378.913060986889832, 306.5512043212590356 ) ) ;
#110525=CARTESIAN_POINT ( 'NONE',  ( -3.771520295670000245, 1377.889610323579973, 206.3143083597190071 ) ) ;
#110537=AXIS2_PLACEMENT_3D ( 'NONE', #76555, #93349, #67628 ) ;
#110553=CARTESIAN_POINT ( 'NONE',  ( -49.59345295620000371, 1385.124330617979922, 260.9076469794590025 ) ) ;
#110555=CARTESIAN_POINT ( 'NONE',  ( -74.11717081736961177, 1385.010645261289937, 299.2649584196010437 ) ) ;
#110565=CARTESIAN_POINT ( 'NONE',  ( -108.8094171845170024, 1382.492531679610011, 310.7655809651279810 ) ) ;
#110586=DIRECTION ( 'NONE',  ( 1.836970198721029688E-16, 1.000000000000000000, 0.000000000000000000 ) ) ;
#110614=CARTESIAN_POINT ( 'NONE',  ( -12.29553027537570031, 1378.313034645889957, 210.0045240490580056 ) ) ;
#110632=CARTESIAN_POINT ( 'NONE',  ( -9.110137399830000149, 1384.581616693699971, 199.9614059229390080 ) ) ;
#110643=CARTESIAN_POINT ( 'NONE',  ( -5.432410439472700858, 1391.426148861440197, 203.3415300314919989 ) ) ;
#110653=CARTESIAN_POINT ( 'NONE',  ( -31.38068168340650033, 1384.559508582369972, 206.3649650040269989 ) ) ;
#110654=CARTESIAN_POINT ( 'NONE',  ( -14.48104889709779997, 1379.655349290230106, 208.1922004443790115 ) ) ;
#110657=VERTEX_POINT ( 'NONE', #74848 ) ;
#110660=CARTESIAN_POINT ( 'NONE',  ( -48.91304988690782807, 1379.688432508924052, 243.6725008576361802 ) ) ;
#110665=CARTESIAN_POINT ( 'NONE',  ( -68.15046949569999413, 1379.746499244090046, 278.7918009234589363 ) ) ;
#110675=CARTESIAN_POINT ( 'NONE',  ( -12.75453511212650071, 1385.302433149910257, 219.0254989633160108 ) ) ;
#110722=LINE ( 'NONE', #17173, #21810 ) ;
#110724=CARTESIAN_POINT ( 'NONE',  ( -54.89834970837709704, 1383.804077747929796, 271.2376706240149815 ) ) ;
#110732=CARTESIAN_POINT ( 'NONE',  ( -57.27373091850000009, 1381.636262940560073, 240.5709706821589862 ) ) ;
#110737=DIRECTION ( 'NONE',  ( 1.402715769532790202E-14, -1.000000000000000000, 4.930380657631320281E-31 ) ) ;
#110742=CARTESIAN_POINT ( 'NONE',  ( -107.5634112720000104, 1382.701802836779962, 297.7923862875589975 ) ) ;
#110766=CARTESIAN_POINT ( 'NONE',  ( -105.7479675089999915, 1388.624540799249871, 309.0709673806589990 ) ) ;
#110811=TOROIDAL_SURFACE ( 'NONE', #96525, 7.499828603750000156, 0.5000000000000000000 ) ;
#110814=CARTESIAN_POINT ( 'NONE',  ( -6.355004502469999927, 1386.605327393260040, 199.7233850259690087 ) ) ;
#110823=CARTESIAN_POINT ( 'NONE',  ( -13.88938984930000053, 1379.665435272789864, 212.4763918038889869 ) ) ;
#110830=CARTESIAN_POINT ( 'NONE',  ( -13.43109441729999887, 1390.552119206370207, 208.3926299382939931 ) ) ;
ENDSEC;
END-ISO-10303-21;
